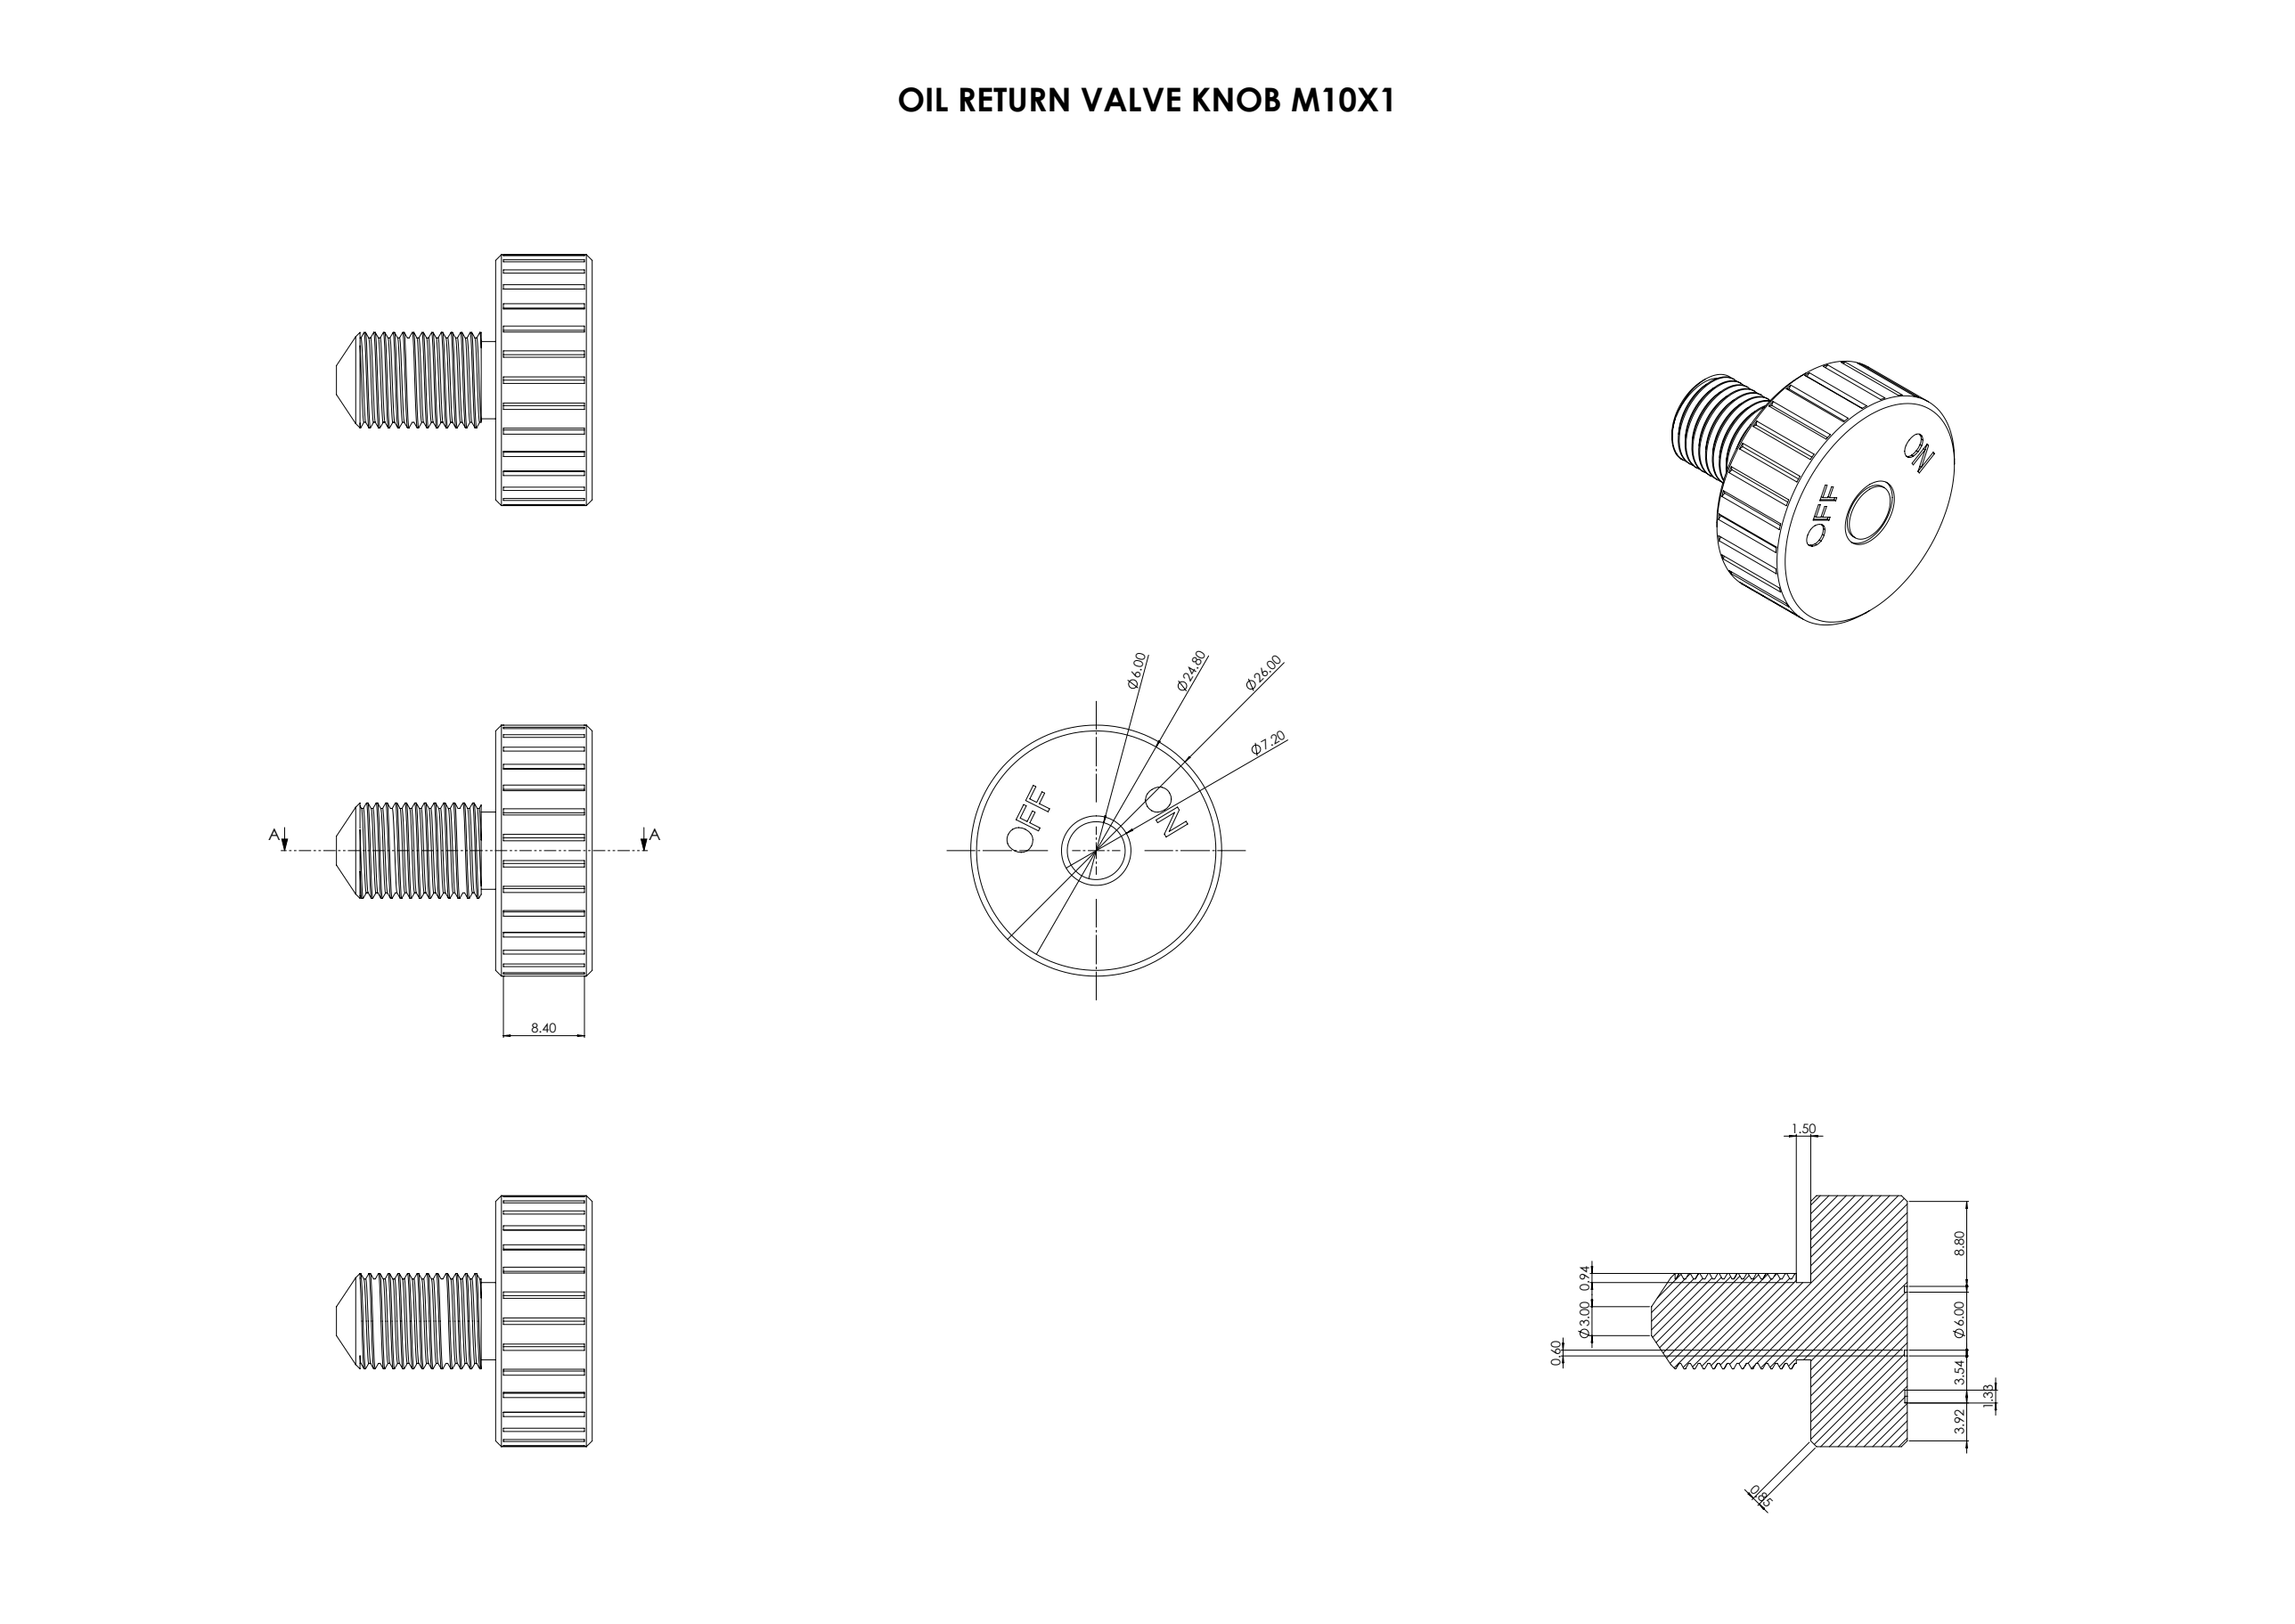
ISO-10303-21;
HEADER;
/* Generated by software containing ST-Developer
 * from STEP Tools, Inc. (www.steptools.com) 
 */

FILE_DESCRIPTION(
/* description */ (''),
/* implementation_level */ '2;1');

FILE_NAME(
/* name */ '20_Oil_Return_Valve_Knob_M10x1.step',
/* time_stamp */ '2026-10-26T03:55:20-07:00',
/* author */ (''),
/* organization */ (''),
/* preprocessor_version */ 'ST-DEVELOPER v20.2',
/* originating_system */ 'Autodesk Translation Framework v15.15.0.0',
/* authorisation */ '');

FILE_SCHEMA (('AUTOMOTIVE_DESIGN { 1 0 10303 214 3 1 1 }'));
ENDSEC;

DATA;
#10=MECHANICAL_DESIGN_GEOMETRIC_PRESENTATION_REPRESENTATION('',(#188),#45236);
#148=SHAPE_REPRESENTATION_RELATIONSHIP('SRR','None',#45327,#168);
#168=ADVANCED_BREP_SHAPE_REPRESENTATION('',(#208),#45229);
#188=STYLED_ITEM('',(#45477),#208);
#208=MANIFOLD_SOLID_BREP('Body1',#16530);
#688=B_SPLINE_CURVE_WITH_KNOTS('',3,(#40645,#40646,#40647,#40648,#40649,
#40650,#40651,#40652,#40653,#40654),.UNSPECIFIED.,.F.,.F.,(4,3,3,4),(-4.09293042013065,
-3.99861591915004,-2.99896193936253,-2.06773127522702),.UNSPECIFIED.);
#689=B_SPLINE_CURVE_WITH_KNOTS('',3,(#40657,#40658,#40659,#40660,#40661,
#40662,#40663,#40664,#40665,#40666),.UNSPECIFIED.,.F.,.F.,(4,3,3,4),(0.,
0.499826989893744,0.999653979787498,1.11639350868611),.UNSPECIFIED.);
#690=B_SPLINE_CURVE_WITH_KNOTS('',3,(#40671,#40672,#40673,#40674,#40675,
#40676,#40677,#40678,#40679,#40680,#40681,#40682,#40683,#40684,#40685,#40686,
#40687,#40688,#40689,#40690,#40691,#40692),.UNSPECIFIED.,.F.,.F.,(4,3,3,
3,3,3,3,4),(-10.3761157273102,-9.99653979787509,-8.99688581808759,-7.99723183830008,
-6.99757785851257,-5.99792387872506,-4.99826989893755,-4.09293042013065),
 .UNSPECIFIED.);
#691=B_SPLINE_CURVE_WITH_KNOTS('',3,(#40693,#40694,#40695,#40696,#40697,
#40698,#40699,#40700,#40701,#40702,#40703,#40704,#40705,#40706,#40707,#40708,
#40709,#40710,#40711,#40712,#40713,#40714),.UNSPECIFIED.,.F.,.F.,(4,3,3,
3,3,3,3,4),(1.11639350868611,1.99930795957501,2.99896193936252,3.99861591915003,
4.99826989893754,5.99792387872506,6.99757785851257,7.39957881586569),
 .UNSPECIFIED.);
#692=B_SPLINE_CURVE_WITH_KNOTS('',3,(#40719,#40720,#40721,#40722,#40723,
#40724,#40725,#40726,#40727,#40728,#40729,#40730,#40731,#40732,#40733,#40734,
#40735,#40736,#40737,#40738,#40739,#40740),.UNSPECIFIED.,.F.,.F.,(4,3,3,
3,3,3,3,4),(-16.6593010344898,-15.9944636766002,-14.9948096968126,-13.9951557170251,
-12.9955017372376,-11.9958477574501,-10.9961937776626,-10.3761157273102),
 .UNSPECIFIED.);
#693=B_SPLINE_CURVE_WITH_KNOTS('',3,(#40741,#40742,#40743,#40744,#40745,
#40746,#40747,#40748,#40749,#40750,#40751,#40752,#40753,#40754,#40755,#40756,
#40757,#40758,#40759,#40760,#40761,#40762),.UNSPECIFIED.,.F.,.F.,(4,3,3,
3,3,3,3,4),(7.39957881586569,7.99723183830008,8.99688581808759,9.9965397978751,
10.9961937776626,11.9958477574501,12.9955017372376,13.6827641230453),
 .UNSPECIFIED.);
#694=B_SPLINE_CURVE_WITH_KNOTS('',3,(#40767,#40768,#40769,#40770,#40771,
#40772,#40773,#40774,#40775,#40776,#40777,#40778,#40779,#40780,#40781,#40782,
#40783,#40784,#40785,#40786,#40787,#40788),.UNSPECIFIED.,.F.,.F.,(4,3,3,
3,3,3,3,4),(-22.9424863416694,-21.9923875553252,-20.9927335755377,-19.9930795957502,
-18.9934256159627,-17.9937716361752,-16.9941176563877,-16.6593010344898),
 .UNSPECIFIED.);
#695=B_SPLINE_CURVE_WITH_KNOTS('',3,(#40789,#40790,#40791,#40792,#40793,
#40794,#40795,#40796,#40797,#40798,#40799,#40800,#40801,#40802,#40803,#40804,
#40805,#40806,#40807,#40808,#40809,#40810),.UNSPECIFIED.,.F.,.F.,(4,3,3,
3,3,3,3,4),(13.6827641230453,13.9951557170251,14.9948096968126,15.9944636766002,
16.9941176563877,17.9937716361752,18.9934256159627,19.9659494302249),
 .UNSPECIFIED.);
#696=B_SPLINE_CURVE_WITH_KNOTS('',3,(#40815,#40816,#40817,#40818,#40819,
#40820,#40821,#40822,#40823,#40824,#40825,#40826,#40827,#40828,#40829,#40830,
#40831,#40832,#40833,#40834,#40835,#40836,#40837,#40838,#40839),
 .UNSPECIFIED.,.F.,.F.,(4,3,3,3,3,3,3,3,4),(-29.225671648849,-28.9899654138378,
-27.9903114340503,-26.9906574542627,-25.9910034744752,-24.9913494946877,
-23.9916955149002,-22.9920415351127,-22.9424863416694),.UNSPECIFIED.);
#697=B_SPLINE_CURVE_WITH_KNOTS('',3,(#40840,#40841,#40842,#40843,#40844,
#40845,#40846,#40847,#40848,#40849,#40850,#40851,#40852,#40853,#40854,#40855,
#40856,#40857,#40858,#40859,#40860,#40861,#40862,#40863,#40864),
 .UNSPECIFIED.,.F.,.F.,(4,3,3,3,3,3,3,3,4),(19.9659494302249,19.9930795957502,
20.9927335755377,21.9923875553252,22.9920415351127,23.9916955149002,24.9913494946877,
25.9910034744752,26.2491347374045),.UNSPECIFIED.);
#698=B_SPLINE_CURVE_WITH_KNOTS('',3,(#40869,#40870,#40871,#40872,#40873,
#40874,#40875,#40876,#40877,#40878,#40879,#40880,#40881,#40882,#40883,#40884,
#40885,#40886,#40887,#40888,#40889,#40890),.UNSPECIFIED.,.F.,.F.,(4,3,3,
3,3,3,3,4),(-35.5088569560286,-34.9878892925628,-33.9882353127753,-32.9885813329878,
-31.9889273532003,-30.9892733734128,-29.9896193936253,-29.225671648849),
 .UNSPECIFIED.);
#699=B_SPLINE_CURVE_WITH_KNOTS('',3,(#40891,#40892,#40893,#40894,#40895,
#40896,#40897,#40898,#40899,#40900,#40901,#40902,#40903,#40904,#40905,#40906,
#40907,#40908,#40909,#40910,#40911,#40912),.UNSPECIFIED.,.F.,.F.,(4,3,3,
3,3,3,3,4),(26.2491347374045,26.9906574542628,27.9903114340503,28.9899654138378,
29.9896193936253,30.9892733734128,31.9889273532003,32.532320044584),
 .UNSPECIFIED.);
#700=B_SPLINE_CURVE_WITH_KNOTS('',3,(#40917,#40918,#40919,#40920,#40921,
#40922,#40923,#40924,#40925,#40926,#40927,#40928,#40929,#40930,#40931,#40932,
#40933,#40934,#40935,#40936,#40937,#40938),.UNSPECIFIED.,.F.,.F.,(4,3,3,
3,3,3,3,4),(-41.7920422632082,-40.9858131712879,-39.9861591915004,-38.9865052117129,
-37.9868512319254,-36.9871972521378,-35.9875432723503,-35.5088569560286),
 .UNSPECIFIED.);
#701=B_SPLINE_CURVE_WITH_KNOTS('',3,(#40939,#40940,#40941,#40942,#40943,
#40944,#40945,#40946,#40947,#40948,#40949,#40950,#40951,#40952,#40953,#40954,
#40955,#40956,#40957,#40958,#40959,#40960),.UNSPECIFIED.,.F.,.F.,(4,3,3,
3,3,3,3,4),(32.532320044584,32.9885813329878,33.9882353127753,34.9878892925628,
35.9875432723503,36.9871972521378,37.9868512319253,38.8155053517636),
 .UNSPECIFIED.);
#702=B_SPLINE_CURVE_WITH_KNOTS('',3,(#40965,#40966,#40967,#40968,#40969,
#40970,#40971,#40972,#40973,#40974,#40975,#40976,#40977,#40978,#40979,#40980,
#40981,#40982,#40983,#40984,#40985,#40986,#40987,#40988,#40989),
 .UNSPECIFIED.,.F.,.F.,(4,3,3,3,3,3,3,3,4),(-48.0752275703878,-47.9833910298005,
-46.9837370500129,-45.9840830702254,-44.9844290904379,-43.9847751106504,
-42.9851211308629,-41.9854671510754,-41.7920422632082),.UNSPECIFIED.);
#703=B_SPLINE_CURVE_WITH_KNOTS('',3,(#40990,#40991,#40992,#40993,#40994,
#40995,#40996,#40997,#40998,#40999,#41000,#41001,#41002,#41003,#41004,#41005,
#41006,#41007,#41008,#41009,#41010,#41011,#41012,#41013,#41014),
 .UNSPECIFIED.,.F.,.F.,(4,3,3,3,3,3,3,3,4),(38.8155053517636,38.9865052117129,
39.9861591915004,40.9858131712879,41.9854671510754,42.9851211308629,43.9847751106504,
44.9844290904379,45.0986906589432),.UNSPECIFIED.);
#704=B_SPLINE_CURVE_WITH_KNOTS('',3,(#41019,#41020,#41021,#41022,#41023,
#41024,#41025,#41026,#41027,#41028,#41029,#41030,#41031,#41032,#41033,#41034,
#41035,#41036,#41037,#41038,#41039,#41040),.UNSPECIFIED.,.F.,.F.,(4,3,3,
3,3,3,3,4),(-54.3584128775673,-53.9813149085255,-52.981660928738,-51.9820069489505,
-50.982352969163,-49.9826989893755,-48.983045009588,-48.0752275703878),
 .UNSPECIFIED.);
#705=B_SPLINE_CURVE_WITH_KNOTS('',3,(#41041,#41042,#41043,#41044,#41045,
#41046,#41047,#41048,#41049,#41050,#41051,#41052,#41053,#41054,#41055,#41056,
#41057,#41058,#41059,#41060,#41061,#41062),.UNSPECIFIED.,.F.,.F.,(4,3,3,
3,3,3,3,4),(45.0986906589432,45.9840830702254,46.9837370500129,47.9833910298004,
48.9830450095879,49.9826989893755,50.982352969163,51.3818759661228),
 .UNSPECIFIED.);
#706=B_SPLINE_CURVE_WITH_KNOTS('',3,(#41067,#41068,#41069,#41070,#41071,
#41072,#41073,#41074,#41075,#41076,#41077,#41078,#41079,#41080,#41081,#41082,
#41083,#41084,#41085,#41086,#41087,#41088),.UNSPECIFIED.,.F.,.F.,(4,3,3,
3,3,3,3,4),(-60.641598184747,-59.9792387872506,-58.979584807463,-57.9799308276755,
-56.980276847888,-55.9806228681005,-54.980968888313,-54.3584128775673),
 .UNSPECIFIED.);
#707=B_SPLINE_CURVE_WITH_KNOTS('',3,(#41089,#41090,#41091,#41092,#41093,
#41094,#41095,#41096,#41097,#41098,#41099,#41100,#41101,#41102,#41103,#41104,
#41105,#41106,#41107,#41108,#41109,#41110),.UNSPECIFIED.,.F.,.F.,(4,3,3,
3,3,3,3,4),(51.3818759661228,51.9820069489505,52.981660928738,53.9813149085255,
54.980968888313,55.9806228681005,56.980276847888,57.6650612733024),
 .UNSPECIFIED.);
#708=B_SPLINE_CURVE_WITH_KNOTS('',3,(#41115,#41116,#41117,#41118,#41119,
#41120,#41121,#41122,#41123,#41124,#41125,#41126,#41127,#41128,#41129,#41130,
#41131,#41132,#41133,#41134,#41135,#41136),.UNSPECIFIED.,.F.,.F.,(4,3,3,
3,3,3,3,4),(-66.9247834919265,-65.9771626659756,-64.9775086861881,-63.9778547064006,
-62.9782007266131,-61.9785467468256,-60.9788927670381,-60.641598184747),
 .UNSPECIFIED.);
#709=B_SPLINE_CURVE_WITH_KNOTS('',3,(#41137,#41138,#41139,#41140,#41141,
#41142,#41143,#41144,#41145,#41146,#41147,#41148,#41149,#41150,#41151,#41152,
#41153,#41154,#41155,#41156,#41157,#41158),.UNSPECIFIED.,.F.,.F.,(4,3,3,
3,3,3,3,4),(57.6650612733024,57.9799308276755,58.9795848074631,59.9792387872506,
60.9788927670381,61.9785467468256,62.9782007266131,63.948246580482),
 .UNSPECIFIED.);
#710=B_SPLINE_CURVE_WITH_KNOTS('',3,(#41163,#41164,#41165,#41166,#41167,
#41168,#41169,#41170,#41171,#41172,#41173,#41174,#41175,#41176,#41177,#41178,
#41179,#41180,#41181,#41182,#41183,#41184,#41185,#41186,#41187),
 .UNSPECIFIED.,.F.,.F.,(4,3,3,3,3,3,3,3,4),(-73.2079687991061,-72.9747405244882,
-71.9750865447007,-70.9754325649132,-69.9757785851257,-68.9761246053381,
-67.9764706255506,-66.9768166457631,-66.9247834919265),.UNSPECIFIED.);
#711=B_SPLINE_CURVE_WITH_KNOTS('',3,(#41188,#41189,#41190,#41191,#41192,
#41193,#41194,#41195,#41196,#41197,#41198,#41199,#41200,#41201,#41202,#41203,
#41204,#41205,#41206,#41207,#41208,#41209,#41210,#41211,#41212),
 .UNSPECIFIED.,.F.,.F.,(4,3,3,3,3,3,3,3,4),(63.948246580482,63.9778547064006,
64.9775086861881,65.9771626659756,66.9768166457631,67.9764706255506,68.9761246053382,
69.9757785851257,70.2314318876616),.UNSPECIFIED.);
#712=B_SPLINE_CURVE_WITH_KNOTS('',3,(#41217,#41218,#41219,#41220,#41221,
#41222,#41223,#41224,#41225,#41226,#41227,#41228,#41229,#41230,#41231,#41232,
#41233,#41234,#41235,#41236,#41237,#41238),.UNSPECIFIED.,.F.,.F.,(4,3,3,
3,3,3,3,4),(-79.4911541062857,-78.9726644032132,-77.9730104234257,-76.9733564436382,
-75.9737024638507,-74.9740484840632,-73.9743945042757,-73.2079687991061),
 .UNSPECIFIED.);
#713=B_SPLINE_CURVE_WITH_KNOTS('',3,(#41239,#41240,#41241,#41242,#41243,
#41244,#41245,#41246,#41247,#41248,#41249,#41250,#41251,#41252,#41253,#41254,
#41255,#41256,#41257,#41258,#41259,#41260),.UNSPECIFIED.,.F.,.F.,(4,3,3,
3,3,3,3,4),(70.2314318876616,70.9754325649132,71.9750865447007,72.9747405244882,
73.9743945042757,74.9740484840632,75.9737024638507,76.5146171948412),
 .UNSPECIFIED.);
#714=B_SPLINE_CURVE_WITH_KNOTS('',3,(#41266,#41267,#41268,#41269,#41270,
#41271,#41272,#41273,#41274),.UNSPECIFIED.,.F.,.F.,(4,1,1,1,1,1,4),(84.8230016469244,
85.5894273520939,86.5890813318814,87.588735311669,88.5883892914565,89.588043271244,
90.5192739353795),.UNSPECIFIED.);
#715=B_SPLINE_CURVE_WITH_KNOTS('',3,(#41277,#41278,#41279,#41280,#41281,
#41282,#41283,#41284,#41285),.UNSPECIFIED.,.F.,.F.,(4,1,1,1,1,1,4),(84.8230016469244,
85.2817408957214,86.2813948755089,87.2810488552964,88.2807028350839,88.7805298249777,
89.2803568148714),.UNSPECIFIED.);
#716=B_SPLINE_CURVE_WITH_KNOTS('',3,(#41290,#41291,#41292,#41293,#41294,
#41295,#41296,#41297,#41298,#41299,#41300),.UNSPECIFIED.,.F.,.F.,(4,1,1,
1,1,1,1,1,4),(78.5398163397448,78.5918494935814,79.5915034733689,80.5911574531564,
81.5908114329439,82.5904654127314,83.5901193925189,84.5897733723064,84.8230016469244),
 .UNSPECIFIED.);
#717=B_SPLINE_CURVE_WITH_KNOTS('',3,(#41301,#41302,#41303,#41304,#41305,
#41306,#41307,#41308,#41309,#41310),.UNSPECIFIED.,.F.,.F.,(4,1,1,1,1,1,
1,4),(78.5398163397448,79.2838170169963,80.2834709967838,81.2831249765713,
82.2827789563588,83.2824329361463,84.2820869159339,84.8230016469244),
 .UNSPECIFIED.);
#718=B_SPLINE_CURVE_WITH_KNOTS('',3,(#41315,#41316,#41317,#41318,#41319,
#41320,#41321,#41322,#41323,#41324),.UNSPECIFIED.,.F.,.F.,(4,1,1,1,1,1,
1,4),(72.2566310325652,72.5939256148563,73.5935795946438,74.5932335744313,
75.5928875542188,76.5925415340064,77.5921955137939,78.5398163397448),
 .UNSPECIFIED.);
#719=B_SPLINE_CURVE_WITH_KNOTS('',3,(#41325,#41326,#41327,#41328,#41329,
#41330,#41331,#41332,#41333,#41334,#41335),.UNSPECIFIED.,.F.,.F.,(4,1,1,
1,1,1,1,1,4),(72.2566310325652,72.2862391584838,73.2858931382713,74.2855471180588,
75.2852010978463,76.2848550776338,77.2845090574213,78.2841630372088,78.5398163397448),
 .UNSPECIFIED.);
#720=B_SPLINE_CURVE_WITH_KNOTS('',3,(#41340,#41341,#41342,#41343,#41344,
#41345,#41346,#41347,#41348,#41349),.UNSPECIFIED.,.F.,.F.,(4,1,1,1,1,1,
1,4),(65.9734457253856,66.5960017361313,67.5956557159188,68.5953096957063,
69.5949636754938,70.5946176552813,71.5942716350688,72.2566310325652),
 .UNSPECIFIED.);
#721=B_SPLINE_CURVE_WITH_KNOTS('',3,(#41350,#41351,#41352,#41353,#41354,
#41355,#41356,#41357,#41358,#41359),.UNSPECIFIED.,.F.,.F.,(4,1,1,1,1,1,
1,4),(65.9734457253856,66.2883152797587,67.2879692595462,68.2876232393337,
69.2872772191212,70.2869311989087,71.2865851786962,72.2566310325652),
 .UNSPECIFIED.);
#722=B_SPLINE_CURVE_WITH_KNOTS('',3,(#41364,#41365,#41366,#41367,#41368,
#41369,#41370,#41371,#41372,#41373),.UNSPECIFIED.,.F.,.F.,(4,1,1,1,1,1,
1,4),(59.690260418206,60.5980778574062,61.5977318371937,62.5973858169812,
63.5970397967687,64.5966937765562,65.5963477563437,65.9734457253856),
 .UNSPECIFIED.);
#723=B_SPLINE_CURVE_WITH_KNOTS('',3,(#41374,#41375,#41376,#41377,#41378,
#41379,#41380,#41381,#41382,#41383),.UNSPECIFIED.,.F.,.F.,(4,1,1,1,1,1,
1,4),(59.690260418206,60.2903914010336,61.2900453808211,62.2896993606087,
63.2893533403962,64.2890073201837,65.2886612999712,65.9734457253856),
 .UNSPECIFIED.);
#724=B_SPLINE_CURVE_WITH_KNOTS('',3,(#41388,#41389,#41390,#41391,#41392,
#41393,#41394,#41395,#41396,#41397,#41398),.UNSPECIFIED.,.F.,.F.,(4,1,1,
1,1,1,1,1,4),(53.4070751110265,53.6004999988936,54.6001539786812,55.5998079584687,
56.5994619382562,57.5991159180437,58.5987698978312,59.5984238776187,59.690260418206),
 .UNSPECIFIED.);
#725=B_SPLINE_CURVE_WITH_KNOTS('',3,(#41399,#41400,#41401,#41402,#41403,
#41404,#41405,#41406,#41407,#41408),.UNSPECIFIED.,.F.,.F.,(4,1,1,1,1,1,
1,4),(53.4070751110264,54.2924675223086,55.2921215020961,56.2917754818836,
57.2914294616711,58.2910834414586,59.2907374212461,59.690260418206),
 .UNSPECIFIED.);
#726=B_SPLINE_CURVE_WITH_KNOTS('',3,(#41413,#41414,#41415,#41416,#41417,
#41418,#41419,#41420,#41421,#41422),.UNSPECIFIED.,.F.,.F.,(4,1,1,1,1,1,
1,4),(47.1238898038469,47.6025761201686,48.6022300999561,49.6018840797436,
50.6015380595311,51.6011920393186,52.6008460191061,53.4070751110265),
 .UNSPECIFIED.);
#727=B_SPLINE_CURVE_WITH_KNOTS('',3,(#41423,#41424,#41425,#41426,#41427,
#41428,#41429,#41430,#41431,#41432,#41433),.UNSPECIFIED.,.F.,.F.,(4,1,1,
1,1,1,1,1,4),(47.1238898038468,47.294889663796,48.2945436435835,49.294197623371,
50.2938516031585,51.2935055829461,52.2931595627336,53.2928135425211,53.4070751110264),
 .UNSPECIFIED.);
#728=B_SPLINE_CURVE_WITH_KNOTS('',3,(#41438,#41439,#41440,#41441,#41442,
#41443,#41444,#41445,#41446,#41447),.UNSPECIFIED.,.F.,.F.,(4,1,1,1,1,1,
1,4),(40.8407044966673,41.6046522414435,42.604306221231,43.6039602010186,
44.6036141808061,45.6032681605936,46.6029221403811,47.1238898038469),
 .UNSPECIFIED.);
#729=B_SPLINE_CURVE_WITH_KNOTS('',3,(#41448,#41449,#41450,#41451,#41452,
#41453,#41454,#41455,#41456,#41457),.UNSPECIFIED.,.F.,.F.,(4,1,1,1,1,1,
1,4),(40.8407044966673,41.296965785071,42.2966197648585,43.296273744646,
44.2959277244335,45.295581704221,46.2952356840085,47.1238898038468),
 .UNSPECIFIED.);
#730=B_SPLINE_CURVE_WITH_KNOTS('',3,(#41462,#41463,#41464,#41465,#41466,
#41467,#41468,#41469,#41470,#41471,#41472),.UNSPECIFIED.,.F.,.F.,(4,1,1,
1,1,1,1,1,4),(34.5575191894877,34.607074382931,35.6067283627185,36.606382342506,
37.6060363222935,38.605690302081,39.6053442818685,40.604998261656,40.8407044966673),
 .UNSPECIFIED.);
#731=B_SPLINE_CURVE_WITH_KNOTS('',3,(#41473,#41474,#41475,#41476,#41477,
#41478,#41479,#41480,#41481,#41482),.UNSPECIFIED.,.F.,.F.,(4,1,1,1,1,1,
1,4),(34.5575191894877,35.2990419063459,36.2986958861334,37.2983498659209,
38.2980038457084,39.2976578254959,40.2973118052834,40.8407044966673),
 .UNSPECIFIED.);
#732=B_SPLINE_CURVE_WITH_KNOTS('',3,(#41487,#41488,#41489,#41490,#41491,
#41492,#41493,#41494,#41495,#41496),.UNSPECIFIED.,.F.,.F.,(4,1,1,1,1,1,
1,4),(28.2743338823081,28.6091505042059,29.6088044839934,30.6084584637809,
31.6081124435684,32.6077664233559,33.6074204031435,34.5575191894877),
 .UNSPECIFIED.);
#733=B_SPLINE_CURVE_WITH_KNOTS('',3,(#41497,#41498,#41499,#41500,#41501,
#41502,#41503,#41504,#41505,#41506,#41507),.UNSPECIFIED.,.F.,.F.,(4,1,1,
1,1,1,1,1,4),(28.2743338823081,28.3014640478333,29.3011180276209,30.3007720074084,
31.3004259871959,32.3000799669834,33.2997339467709,34.2993879265584,34.5575191894877),
 .UNSPECIFIED.);
#734=B_SPLINE_CURVE_WITH_KNOTS('',3,(#41512,#41513,#41514,#41515,#41516,
#41517,#41518,#41519,#41520,#41521),.UNSPECIFIED.,.F.,.F.,(4,1,1,1,1,1,
1,4),(21.9911485751285,22.6112266254809,23.6108806052684,24.6105345850559,
25.6101885648434,26.6098425446309,27.6094965244184,28.2743338823081),
 .UNSPECIFIED.);
#735=B_SPLINE_CURVE_WITH_KNOTS('',3,(#41522,#41523,#41524,#41525,#41526,
#41527,#41528,#41529,#41530,#41531),.UNSPECIFIED.,.F.,.F.,(4,1,1,1,1,1,
1,4),(21.9911485751285,22.3035401691083,23.3031941488958,24.3028481286833,
25.3025021084708,26.3021560882583,27.3018100680458,28.2743338823081),
 .UNSPECIFIED.);
#736=B_SPLINE_CURVE_WITH_KNOTS('',3,(#41536,#41537,#41538,#41539,#41540,
#41541,#41542,#41543,#41544,#41545),.UNSPECIFIED.,.F.,.F.,(4,1,1,1,1,1,
1,4),(15.7079632679489,16.6133027467558,17.6129567265433,18.6126107063308,
19.6122646861183,20.6119186659058,21.6115726456933,21.9911485751285),
 .UNSPECIFIED.);
#737=B_SPLINE_CURVE_WITH_KNOTS('',3,(#41546,#41547,#41548,#41549,#41550,
#41551,#41552,#41553,#41554,#41555),.UNSPECIFIED.,.F.,.F.,(4,1,1,1,1,1,
1,4),(15.7079632679489,16.3056162903832,17.3052702701707,18.3049242499582,
19.3045782297458,20.3042322095333,21.3038861893208,21.9911485751285),
 .UNSPECIFIED.);
#738=B_SPLINE_CURVE_WITH_KNOTS('',3,(#41901,#41902,#41903,#41904,#41905,
#41906,#41907,#41908,#41909,#41910,#41911,#41912,#41913,#41914,#41915,#41916,
#41917,#41918,#41919,#41920,#41921,#41922,#41923,#41924,#41925,#41926,#41927,
#41928,#41929,#41930,#41931,#41932,#41933,#41934,#41935,#41936,#41937,#41938,
#41939,#41940,#41941,#41942,#41943,#41944,#41945,#41946,#41947,#41948,#41949,
#41950,#41951,#41952,#41953,#41954,#41955,#41956,#41957,#41958,#41959,#41960,
#41961,#41962,#41963,#41964,#41965,#41966,#41967,#41968,#41969,#41970,#41971,
#41972,#41973,#41974,#41975,#41976,#41977,#41978,#41979,#41980,#41981,#41982,
#41983,#41984,#41985,#41986,#41987,#41988,#41989,#41990,#41991,#41992,#41993,
#41994,#41995,#41996,#41997,#41998,#41999,#42000,#42001,#42002,#42003,#42004,
#42005,#42006),.UNSPECIFIED.,.F.,.F.,(4,3,3,3,3,3,3,3,3,3,3,3,3,3,3,3,3,
3,3,3,3,3,3,3,3,3,3,3,3,3,3,3,3,3,3,4),(0.,0.0338555796810951,0.0769233841266441,
0.120787014647652,0.164925431151007,0.18768890800956,0.194695307248219,
0.238000863207828,0.281439200502724,0.324499409932901,0.366791407667859,
0.3748100813225,0.380721434265749,0.423140467769373,0.465072972528112,0.506007047124889,
0.514994378647384,0.543782123537011,0.559160795079789,0.5652443143728,0.606242278680173,
0.647897807448946,0.68940569438575,0.717351016075074,0.73199453794532,0.73810671067074,
0.744081074726445,0.745296337764399,0.786338138284623,0.827324070719474,
0.844968273899783,0.854029216944208,0.860905275211015,0.901330989685579,
0.941119121741644,0.968477696161942),.UNSPECIFIED.);
#739=B_SPLINE_CURVE_WITH_KNOTS('',3,(#42007,#42008,#42009,#42010,#42011,
#42012,#42013,#42014,#42015,#42016),.UNSPECIFIED.,.F.,.F.,(4,3,3,4),(76.5146171948412,
76.9733564436382,77.9730104234257,78.9042410875612),.UNSPECIFIED.);
#740=B_SPLINE_CURVE_WITH_KNOTS('',3,(#42018,#42019,#42020,#42021,#42022,
#42023,#42024,#42025,#42026,#42027,#42028,#42029,#42030,#42031,#42032,#42033,
#42034,#42035,#42036,#42037,#42038,#42039,#42040,#42041,#42042,#42043,#42044,
#42045,#42046,#42047,#42048,#42049,#42050,#42051,#42052,#42053,#42054,#42055,
#42056,#42057,#42058,#42059,#42060,#42061,#42062,#42063,#42064,#42065,#42066,
#42067,#42068,#42069,#42070,#42071,#42072,#42073,#42074,#42075,#42076,#42077,
#42078,#42079,#42080,#42081,#42082,#42083,#42084,#42085,#42086,#42087,#42088,
#42089,#42090,#42091,#42092,#42093,#42094,#42095,#42096,#42097,#42098,#42099,
#42100,#42101,#42102,#42103,#42104,#42105,#42106,#42107,#42108,#42109,#42110,
#42111,#42112,#42113,#42114,#42115,#42116,#42117,#42118,#42119,#42120,#42121,
#42122,#42123),.UNSPECIFIED.,.F.,.F.,(4,3,3,3,3,3,3,3,3,3,3,3,3,3,3,3,3,
3,3,3,3,3,3,3,3,3,3,3,3,3,3,3,3,3,3,4),(-0.968477696161962,-0.93834507440756,
-0.898946379179402,-0.87294341376282,-0.858683439823016,-0.849690155368511,
-0.809511368983842,-0.768684814425123,-0.750823196805684,-0.741908901548402,
-0.734140763767536,-0.692650400513915,-0.650694074697968,-0.608745289151999,
-0.577283699992522,-0.564269250932409,-0.556001088558624,-0.513396717295649,
-0.482898932514091,-0.441404470015905,-0.399314127094565,-0.388144431730235,
-0.378349906522554,-0.373280079897934,-0.331122936037102,-0.287943314322124,
-0.244763692607147,-0.214168231031253,-0.200545763543443,-0.193054146419399,
-0.187017976020424,-0.143637415837001,-0.0997905213121978,-0.0560615532128227,
-0.0129908569656951,0.),.UNSPECIFIED.);
#741=B_SPLINE_CURVE_WITH_KNOTS('',3,(#42124,#42125,#42126,#42127,#42128,
#42129,#42130,#42131,#42132),.UNSPECIFIED.,.F.,.F.,(4,1,1,1,1,1,4),(10.3761157273102,
11.3073463914457,12.3070003712332,13.3066543510207,14.3063083308082,15.3059623105957,
15.7079632679489),.UNSPECIFIED.);
#742=B_SPLINE_CURVE_WITH_KNOTS('',3,(#42138,#42139,#42140,#42141,#42142,
#42143,#42144,#42145,#42146,#42147,#42148,#42149,#42150,#42151,#42152,#42153,
#42154,#42155,#42156,#42157,#42158,#42159,#42160,#42161,#42162,#42163,#42164,
#42165,#42166,#42167,#42168,#42169,#42170,#42171,#42172,#42173,#42174,#42175,
#42176,#42177,#42178,#42179,#42180,#42181,#42182,#42183,#42184,#42185,#42186,
#42187,#42188,#42189,#42190,#42191,#42192,#42193,#42194,#42195,#42196,#42197,
#42198,#42199,#42200,#42201,#42202,#42203,#42204,#42205,#42206,#42207,#42208,
#42209,#42210,#42211,#42212,#42213,#42214,#42215,#42216,#42217,#42218,#42219,
#42220,#42221,#42222,#42223,#42224,#42225,#42226,#42227,#42228,#42229,#42230,
#42231,#42232,#42233,#42234,#42235,#42236,#42237,#42238,#42239,#42240,#42241,
#42242,#42243,#42244,#42245,#42246,#42247,#42248,#42249),.UNSPECIFIED.,
 .F.,.F.,(4,3,3,3,3,3,3,3,3,3,3,3,3,3,3,3,3,3,3,3,3,3,3,3,3,3,3,3,3,3,3,
3,3,3,3,3,3,4),(-0.965990216419493,-0.932232205964582,-0.888725512381132,
-0.86148182111266,-0.845752215774746,-0.838628962985686,-0.795398770998977,
-0.752577231134802,-0.732526991421503,-0.722290315506079,-0.715478178658122,
-0.709647482806995,-0.666593990274609,-0.623625418609477,-0.580925676978502,
-0.54890087075527,-0.536423601193463,-0.530582682015647,-0.525159930165745,
-0.483534316458395,-0.452826452085574,-0.410953138863345,-0.368980079811334,
-0.356959708801849,-0.350330796437256,-0.345496631210951,-0.304366782550378,
-0.263166867623492,-0.222981343541229,-0.195108675598575,-0.181421822833585,
-0.173192140728228,-0.16726444049677,-0.125448330372578,-0.0850057436766688,
-0.0449541457505024,-0.00571652159400748,0.),.UNSPECIFIED.);
#743=B_SPLINE_CURVE_WITH_KNOTS('',3,(#42252,#42253,#42254,#42255,#42256,
#42257,#42258,#42259,#42260),.UNSPECIFIED.,.F.,.F.,(4,1,1,1,1,1,4),(11.6150328478183,
12.114859837712,12.6146868276058,13.6143408073933,14.6139947871808,15.6136487669683,
15.7079632679489),.UNSPECIFIED.);
#744=B_SPLINE_CURVE_WITH_KNOTS('',3,(#42606,#42607,#42608,#42609,#42610,
#42611,#42612,#42613,#42614,#42615,#42616,#42617,#42618,#42619,#42620,#42621,
#42622,#42623,#42624,#42625,#42626,#42627,#42628,#42629,#42630,#42631,#42632,
#42633,#42634,#42635,#42636,#42637,#42638,#42639,#42640,#42641,#42642,#42643,
#42644,#42645,#42646,#42647,#42648,#42649,#42650,#42651,#42652,#42653,#42654,
#42655,#42656,#42657,#42658,#42659,#42660,#42661,#42662,#42663,#42664,#42665,
#42666,#42667,#42668,#42669,#42670,#42671,#42672,#42673,#42674,#42675,#42676,
#42677,#42678,#42679,#42680,#42681,#42682,#42683,#42684,#42685,#42686,#42687,
#42688,#42689,#42690,#42691,#42692,#42693,#42694,#42695,#42696,#42697,#42698,
#42699,#42700,#42701,#42702,#42703,#42704,#42705,#42706,#42707,#42708,#42709,
#42710,#42711,#42712,#42713,#42714),.UNSPECIFIED.,.F.,.F.,(4,3,3,3,3,3,
3,3,3,3,3,3,3,3,3,3,3,3,3,3,3,3,3,3,3,3,3,3,3,3,3,3,3,3,3,3,4),(0.,0.0300808882250601,
0.0690837691274257,0.108977971558979,0.149535303300715,0.161775980247188,
0.169677926634296,0.176345077737452,0.217218238973177,0.258694872125898,
0.300344044967144,0.341653389143491,0.347771209594167,0.352609284959025,
0.39494049143562,0.437189104774325,0.478722267806855,0.48483985412653,0.51451003945568,
0.524490292215405,0.530274299792254,0.571233373520478,0.613481573281312,
0.656140144392953,0.689170740576341,0.705686038668035,0.714536893087061,
0.720494023679387,0.722201336759729,0.765231119221639,0.808568534613332,
0.828246244839095,0.838610463895481,0.846178719169224,0.890004704789425,
0.933557298850571,0.965990216419437),.UNSPECIFIED.);
#745=B_SPLINE_CURVE_WITH_KNOTS('',3,(#42715,#42716,#42717,#42718,#42719,
#42720,#42721,#42722,#42723,#42724),.UNSPECIFIED.,.F.,.F.,(4,3,3,4),(-80.9719723627883,
-80.4721453728945,-79.9723183830007,-79.4911541062857),.UNSPECIFIED.);
#746=B_SPLINE_CURVE_WITH_KNOTS('',2,(#42737,#42738,#42739),
 .UNSPECIFIED.,.F.,.F.,(3,3),(0.,1.),.UNSPECIFIED.);
#747=B_SPLINE_CURVE_WITH_KNOTS('',2,(#42743,#42744,#42745),
 .UNSPECIFIED.,.F.,.F.,(3,3),(0.,1.),.UNSPECIFIED.);
#748=B_SPLINE_CURVE_WITH_KNOTS('',2,(#42754,#42755,#42756),
 .UNSPECIFIED.,.F.,.F.,(3,3),(0.,1.),.UNSPECIFIED.);
#749=B_SPLINE_CURVE_WITH_KNOTS('',2,(#42759,#42760,#42761),
 .UNSPECIFIED.,.F.,.F.,(3,3),(0.,1.),.UNSPECIFIED.);
#750=B_SPLINE_CURVE_WITH_KNOTS('',2,(#42769,#42770,#42771),
 .UNSPECIFIED.,.F.,.F.,(3,3),(0.,1.),.UNSPECIFIED.);
#751=B_SPLINE_CURVE_WITH_KNOTS('',2,(#42774,#42775,#42776),
 .UNSPECIFIED.,.F.,.F.,(3,3),(0.,1.),.UNSPECIFIED.);
#752=B_SPLINE_CURVE_WITH_KNOTS('',2,(#42784,#42785,#42786),
 .UNSPECIFIED.,.F.,.F.,(3,3),(0.,1.),.UNSPECIFIED.);
#753=B_SPLINE_CURVE_WITH_KNOTS('',2,(#42789,#42790,#42791),
 .UNSPECIFIED.,.F.,.F.,(3,3),(0.,1.),.UNSPECIFIED.);
#754=B_SPLINE_CURVE_WITH_KNOTS('',2,(#42799,#42800,#42801),
 .UNSPECIFIED.,.F.,.F.,(3,3),(0.,1.),.UNSPECIFIED.);
#755=B_SPLINE_CURVE_WITH_KNOTS('',2,(#42804,#42805,#42806),
 .UNSPECIFIED.,.F.,.F.,(3,3),(0.,1.),.UNSPECIFIED.);
#756=B_SPLINE_CURVE_WITH_KNOTS('',2,(#42814,#42815,#42816),
 .UNSPECIFIED.,.F.,.F.,(3,3),(0.,1.),.UNSPECIFIED.);
#757=B_SPLINE_CURVE_WITH_KNOTS('',2,(#42819,#42820,#42821),
 .UNSPECIFIED.,.F.,.F.,(3,3),(0.,1.),.UNSPECIFIED.);
#758=B_SPLINE_CURVE_WITH_KNOTS('',2,(#42829,#42830,#42831),
 .UNSPECIFIED.,.F.,.F.,(3,3),(0.,1.),.UNSPECIFIED.);
#759=B_SPLINE_CURVE_WITH_KNOTS('',2,(#42834,#42835,#42836),
 .UNSPECIFIED.,.F.,.F.,(3,3),(0.,1.),.UNSPECIFIED.);
#760=B_SPLINE_CURVE_WITH_KNOTS('',2,(#42844,#42845,#42846),
 .UNSPECIFIED.,.F.,.F.,(3,3),(0.,1.),.UNSPECIFIED.);
#761=B_SPLINE_CURVE_WITH_KNOTS('',2,(#42849,#42850,#42851),
 .UNSPECIFIED.,.F.,.F.,(3,3),(0.,1.),.UNSPECIFIED.);
#762=B_SPLINE_CURVE_WITH_KNOTS('',2,(#42859,#42860,#42861),
 .UNSPECIFIED.,.F.,.F.,(3,3),(0.,1.),.UNSPECIFIED.);
#763=B_SPLINE_CURVE_WITH_KNOTS('',2,(#42864,#42865,#42866),
 .UNSPECIFIED.,.F.,.F.,(3,3),(0.,1.),.UNSPECIFIED.);
#764=B_SPLINE_CURVE_WITH_KNOTS('',2,(#42874,#42875,#42876),
 .UNSPECIFIED.,.F.,.F.,(3,3),(0.,1.),.UNSPECIFIED.);
#765=B_SPLINE_CURVE_WITH_KNOTS('',2,(#42879,#42880,#42881),
 .UNSPECIFIED.,.F.,.F.,(3,3),(0.,1.),.UNSPECIFIED.);
#766=B_SPLINE_CURVE_WITH_KNOTS('',2,(#42888,#42889,#42890),
 .UNSPECIFIED.,.F.,.F.,(3,3),(0.,1.),.UNSPECIFIED.);
#767=B_SPLINE_CURVE_WITH_KNOTS('',2,(#42891,#42892,#42893),
 .UNSPECIFIED.,.F.,.F.,(3,3),(0.,1.),.UNSPECIFIED.);
#768=B_SPLINE_CURVE_WITH_KNOTS('',2,(#42964,#42965,#42966),
 .UNSPECIFIED.,.F.,.F.,(3,3),(0.,1.),.UNSPECIFIED.);
#769=B_SPLINE_CURVE_WITH_KNOTS('',2,(#42970,#42971,#42972),
 .UNSPECIFIED.,.F.,.F.,(3,3),(0.,1.),.UNSPECIFIED.);
#770=B_SPLINE_CURVE_WITH_KNOTS('',2,(#42981,#42982,#42983),
 .UNSPECIFIED.,.F.,.F.,(3,3),(0.,1.),.UNSPECIFIED.);
#771=B_SPLINE_CURVE_WITH_KNOTS('',2,(#42986,#42987,#42988),
 .UNSPECIFIED.,.F.,.F.,(3,3),(0.,1.),.UNSPECIFIED.);
#772=B_SPLINE_CURVE_WITH_KNOTS('',2,(#42996,#42997,#42998),
 .UNSPECIFIED.,.F.,.F.,(3,3),(0.,1.),.UNSPECIFIED.);
#773=B_SPLINE_CURVE_WITH_KNOTS('',2,(#43001,#43002,#43003),
 .UNSPECIFIED.,.F.,.F.,(3,3),(0.,1.),.UNSPECIFIED.);
#774=B_SPLINE_CURVE_WITH_KNOTS('',2,(#43011,#43012,#43013),
 .UNSPECIFIED.,.F.,.F.,(3,3),(0.,1.),.UNSPECIFIED.);
#775=B_SPLINE_CURVE_WITH_KNOTS('',2,(#43016,#43017,#43018),
 .UNSPECIFIED.,.F.,.F.,(3,3),(0.,1.),.UNSPECIFIED.);
#776=B_SPLINE_CURVE_WITH_KNOTS('',2,(#43026,#43027,#43028),
 .UNSPECIFIED.,.F.,.F.,(3,3),(0.,1.),.UNSPECIFIED.);
#777=B_SPLINE_CURVE_WITH_KNOTS('',2,(#43031,#43032,#43033),
 .UNSPECIFIED.,.F.,.F.,(3,3),(0.,1.),.UNSPECIFIED.);
#778=B_SPLINE_CURVE_WITH_KNOTS('',2,(#43041,#43042,#43043),
 .UNSPECIFIED.,.F.,.F.,(3,3),(0.,1.),.UNSPECIFIED.);
#779=B_SPLINE_CURVE_WITH_KNOTS('',2,(#43046,#43047,#43048),
 .UNSPECIFIED.,.F.,.F.,(3,3),(0.,1.),.UNSPECIFIED.);
#780=B_SPLINE_CURVE_WITH_KNOTS('',2,(#43056,#43057,#43058),
 .UNSPECIFIED.,.F.,.F.,(3,3),(0.,1.),.UNSPECIFIED.);
#781=B_SPLINE_CURVE_WITH_KNOTS('',2,(#43061,#43062,#43063),
 .UNSPECIFIED.,.F.,.F.,(3,3),(0.,1.),.UNSPECIFIED.);
#782=B_SPLINE_CURVE_WITH_KNOTS('',2,(#43071,#43072,#43073),
 .UNSPECIFIED.,.F.,.F.,(3,3),(0.,1.),.UNSPECIFIED.);
#783=B_SPLINE_CURVE_WITH_KNOTS('',2,(#43076,#43077,#43078),
 .UNSPECIFIED.,.F.,.F.,(3,3),(0.,1.),.UNSPECIFIED.);
#784=B_SPLINE_CURVE_WITH_KNOTS('',2,(#43086,#43087,#43088),
 .UNSPECIFIED.,.F.,.F.,(3,3),(0.,1.),.UNSPECIFIED.);
#785=B_SPLINE_CURVE_WITH_KNOTS('',2,(#43091,#43092,#43093),
 .UNSPECIFIED.,.F.,.F.,(3,3),(0.,1.),.UNSPECIFIED.);
#786=B_SPLINE_CURVE_WITH_KNOTS('',2,(#43101,#43102,#43103),
 .UNSPECIFIED.,.F.,.F.,(3,3),(0.,1.),.UNSPECIFIED.);
#787=B_SPLINE_CURVE_WITH_KNOTS('',2,(#43106,#43107,#43108),
 .UNSPECIFIED.,.F.,.F.,(3,3),(0.,1.),.UNSPECIFIED.);
#788=B_SPLINE_CURVE_WITH_KNOTS('',2,(#43115,#43116,#43117),
 .UNSPECIFIED.,.F.,.F.,(3,3),(0.,1.),.UNSPECIFIED.);
#789=B_SPLINE_CURVE_WITH_KNOTS('',2,(#43118,#43119,#43120),
 .UNSPECIFIED.,.F.,.F.,(3,3),(0.,1.),.UNSPECIFIED.);
#907=B_SPLINE_SURFACE_WITH_KNOTS('',3,3,((#41556,#41557,#41558,#41559,#41560,
#41561,#41562,#41563,#41564,#41565,#41566,#41567,#41568,#41569,#41570,#41571,
#41572,#41573,#41574,#41575,#41576,#41577,#41578,#41579,#41580,#41581,#41582,
#41583,#41584,#41585,#41586,#41587,#41588,#41589,#41590,#41591,#41592,#41593,
#41594,#41595,#41596,#41597,#41598,#41599,#41600,#41601,#41602,#41603,#41604,
#41605,#41606,#41607,#41608,#41609,#41610,#41611,#41612,#41613,#41614,#41615,
#41616,#41617,#41618,#41619,#41620,#41621,#41622,#41623,#41624,#41625,#41626,
#41627,#41628,#41629,#41630,#41631,#41632,#41633,#41634,#41635,#41636,#41637,
#41638,#41639,#41640,#41641),(#41642,#41643,#41644,#41645,#41646,#41647,
#41648,#41649,#41650,#41651,#41652,#41653,#41654,#41655,#41656,#41657,#41658,
#41659,#41660,#41661,#41662,#41663,#41664,#41665,#41666,#41667,#41668,#41669,
#41670,#41671,#41672,#41673,#41674,#41675,#41676,#41677,#41678,#41679,#41680,
#41681,#41682,#41683,#41684,#41685,#41686,#41687,#41688,#41689,#41690,#41691,
#41692,#41693,#41694,#41695,#41696,#41697,#41698,#41699,#41700,#41701,#41702,
#41703,#41704,#41705,#41706,#41707,#41708,#41709,#41710,#41711,#41712,#41713,
#41714,#41715,#41716,#41717,#41718,#41719,#41720,#41721,#41722,#41723,#41724,
#41725,#41726,#41727),(#41728,#41729,#41730,#41731,#41732,#41733,#41734,
#41735,#41736,#41737,#41738,#41739,#41740,#41741,#41742,#41743,#41744,#41745,
#41746,#41747,#41748,#41749,#41750,#41751,#41752,#41753,#41754,#41755,#41756,
#41757,#41758,#41759,#41760,#41761,#41762,#41763,#41764,#41765,#41766,#41767,
#41768,#41769,#41770,#41771,#41772,#41773,#41774,#41775,#41776,#41777,#41778,
#41779,#41780,#41781,#41782,#41783,#41784,#41785,#41786,#41787,#41788,#41789,
#41790,#41791,#41792,#41793,#41794,#41795,#41796,#41797,#41798,#41799,#41800,
#41801,#41802,#41803,#41804,#41805,#41806,#41807,#41808,#41809,#41810,#41811,
#41812,#41813),(#41814,#41815,#41816,#41817,#41818,#41819,#41820,#41821,
#41822,#41823,#41824,#41825,#41826,#41827,#41828,#41829,#41830,#41831,#41832,
#41833,#41834,#41835,#41836,#41837,#41838,#41839,#41840,#41841,#41842,#41843,
#41844,#41845,#41846,#41847,#41848,#41849,#41850,#41851,#41852,#41853,#41854,
#41855,#41856,#41857,#41858,#41859,#41860,#41861,#41862,#41863,#41864,#41865,
#41866,#41867,#41868,#41869,#41870,#41871,#41872,#41873,#41874,#41875,#41876,
#41877,#41878,#41879,#41880,#41881,#41882,#41883,#41884,#41885,#41886,#41887,
#41888,#41889,#41890,#41891,#41892,#41893,#41894,#41895,#41896,#41897,#41898,
#41899)),.UNSPECIFIED.,.F.,.F.,.F.,(4,4),(4,1,1,1,1,1,1,1,1,1,1,1,1,1,1,
1,1,1,1,1,1,1,1,1,1,1,1,1,1,1,1,1,1,1,1,1,1,1,1,1,1,1,1,1,1,1,1,1,1,1,1,
1,1,1,1,1,1,1,1,1,1,1,1,1,1,1,1,1,1,1,1,1,1,1,1,1,1,1,1,1,1,1,1,4),(0.,
0.0658179306876173),(8.30838445208316,8.80821144197691,9.30803843187066,
10.3076924116582,11.3073463914457,12.3070003712332,13.3066543510207,14.3063083308082,
15.3059623105957,16.3056162903832,17.3052702701707,18.3049242499582,19.3045782297458,
20.3042322095333,21.3038861893208,22.3035401691083,23.3031941488958,24.3028481286833,
25.3025021084708,26.3021560882583,27.3018100680458,28.3014640478333,29.3011180276209,
30.3007720074084,31.3004259871959,32.3000799669834,33.2997339467709,34.2993879265584,
35.2990419063459,36.2986958861334,37.2983498659209,38.2980038457084,39.2976578254959,
40.2973118052834,41.296965785071,42.2966197648585,43.296273744646,44.2959277244335,
45.295581704221,46.2952356840085,47.294889663796,48.2945436435835,49.294197623371,
50.2938516031585,51.2935055829461,52.2931595627336,53.2928135425211,54.2924675223086,
55.2921215020961,56.2917754818836,57.2914294616711,58.2910834414586,59.2907374212461,
60.2903914010336,61.2900453808211,62.2896993606087,63.2893533403962,64.2890073201837,
65.2886612999712,66.2883152797587,67.2879692595462,68.2876232393337,69.2872772191212,
70.2869311989087,71.2865851786962,72.2862391584838,73.2858931382713,74.2855471180588,
75.2852010978463,76.2848550776338,77.2845090574213,78.2841630372088,79.2838170169963,
80.2834709967838,81.2831249765713,82.2827789563588,83.2824329361463,84.2820869159339,
85.2817408957214,86.2813948755089,87.2810488552964,88.2807028350839,88.7805298249777,
89.2803568148714),.UNSPECIFIED.);
#908=B_SPLINE_SURFACE_WITH_KNOTS('',3,3,((#42261,#42262,#42263,#42264,#42265,
#42266,#42267,#42268,#42269,#42270,#42271,#42272,#42273,#42274,#42275,#42276,
#42277,#42278,#42279,#42280,#42281,#42282,#42283,#42284,#42285,#42286,#42287,
#42288,#42289,#42290,#42291,#42292,#42293,#42294,#42295,#42296,#42297,#42298,
#42299,#42300,#42301,#42302,#42303,#42304,#42305,#42306,#42307,#42308,#42309,
#42310,#42311,#42312,#42313,#42314,#42315,#42316,#42317,#42318,#42319,#42320,
#42321,#42322,#42323,#42324,#42325,#42326,#42327,#42328,#42329,#42330,#42331,
#42332,#42333,#42334,#42335,#42336,#42337,#42338,#42339,#42340,#42341,#42342,
#42343,#42344,#42345,#42346),(#42347,#42348,#42349,#42350,#42351,#42352,
#42353,#42354,#42355,#42356,#42357,#42358,#42359,#42360,#42361,#42362,#42363,
#42364,#42365,#42366,#42367,#42368,#42369,#42370,#42371,#42372,#42373,#42374,
#42375,#42376,#42377,#42378,#42379,#42380,#42381,#42382,#42383,#42384,#42385,
#42386,#42387,#42388,#42389,#42390,#42391,#42392,#42393,#42394,#42395,#42396,
#42397,#42398,#42399,#42400,#42401,#42402,#42403,#42404,#42405,#42406,#42407,
#42408,#42409,#42410,#42411,#42412,#42413,#42414,#42415,#42416,#42417,#42418,
#42419,#42420,#42421,#42422,#42423,#42424,#42425,#42426,#42427,#42428,#42429,
#42430,#42431,#42432),(#42433,#42434,#42435,#42436,#42437,#42438,#42439,
#42440,#42441,#42442,#42443,#42444,#42445,#42446,#42447,#42448,#42449,#42450,
#42451,#42452,#42453,#42454,#42455,#42456,#42457,#42458,#42459,#42460,#42461,
#42462,#42463,#42464,#42465,#42466,#42467,#42468,#42469,#42470,#42471,#42472,
#42473,#42474,#42475,#42476,#42477,#42478,#42479,#42480,#42481,#42482,#42483,
#42484,#42485,#42486,#42487,#42488,#42489,#42490,#42491,#42492,#42493,#42494,
#42495,#42496,#42497,#42498,#42499,#42500,#42501,#42502,#42503,#42504,#42505,
#42506,#42507,#42508,#42509,#42510,#42511,#42512,#42513,#42514,#42515,#42516,
#42517,#42518),(#42519,#42520,#42521,#42522,#42523,#42524,#42525,#42526,
#42527,#42528,#42529,#42530,#42531,#42532,#42533,#42534,#42535,#42536,#42537,
#42538,#42539,#42540,#42541,#42542,#42543,#42544,#42545,#42546,#42547,#42548,
#42549,#42550,#42551,#42552,#42553,#42554,#42555,#42556,#42557,#42558,#42559,
#42560,#42561,#42562,#42563,#42564,#42565,#42566,#42567,#42568,#42569,#42570,
#42571,#42572,#42573,#42574,#42575,#42576,#42577,#42578,#42579,#42580,#42581,
#42582,#42583,#42584,#42585,#42586,#42587,#42588,#42589,#42590,#42591,#42592,
#42593,#42594,#42595,#42596,#42597,#42598,#42599,#42600,#42601,#42602,#42603,
#42604)),.UNSPECIFIED.,.F.,.F.,.F.,(4,4),(4,1,1,1,1,1,1,1,1,1,1,1,1,1,1,
1,1,1,1,1,1,1,1,1,1,1,1,1,1,1,1,1,1,1,1,1,1,1,1,1,1,1,1,1,1,1,1,1,1,1,1,
1,1,1,1,1,1,1,1,1,1,1,1,1,1,1,1,1,1,1,1,1,1,1,1,1,1,1,1,1,1,1,1,4),(0.,
0.0658179306876173),(11.6150328478183,12.114859837712,12.6146868276058,
13.6143408073933,14.6139947871808,15.6136487669683,16.6133027467558,17.6129567265433,
18.6126107063308,19.6122646861183,20.6119186659058,21.6115726456933,22.6112266254809,
23.6108806052684,24.6105345850559,25.6101885648434,26.6098425446309,27.6094965244184,
28.6091505042059,29.6088044839934,30.6084584637809,31.6081124435684,32.6077664233559,
33.6074204031435,34.607074382931,35.6067283627185,36.606382342506,37.6060363222935,
38.605690302081,39.6053442818685,40.604998261656,41.6046522414435,42.604306221231,
43.6039602010186,44.6036141808061,45.6032681605936,46.6029221403811,47.6025761201686,
48.6022300999561,49.6018840797436,50.6015380595311,51.6011920393186,52.6008460191061,
53.6004999988936,54.6001539786812,55.5998079584687,56.5994619382562,57.5991159180437,
58.5987698978312,59.5984238776187,60.5980778574062,61.5977318371937,62.5973858169812,
63.5970397967687,64.5966937765562,65.5963477563437,66.5960017361313,67.5956557159188,
68.5953096957063,69.5949636754938,70.5946176552813,71.5942716350688,72.5939256148563,
73.5935795946438,74.5932335744313,75.5928875542188,76.5925415340064,77.5921955137939,
78.5918494935814,79.5915034733689,80.5911574531564,81.5908114329439,82.5904654127314,
83.5901193925189,84.5897733723064,85.5894273520939,86.5890813318814,87.588735311669,
88.5883892914565,89.588043271244,90.5876972510315,91.587351230819,92.0871782207128,
92.5870052106065),.UNSPECIFIED.);
#909=B_SPLINE_SURFACE_WITH_KNOTS('',2,1,((#42729,#42730),(#42731,#42732),
(#42733,#42734)),.UNSPECIFIED.,.F.,.F.,.F.,(3,3),(2,2),(0.,1.),(0.,0.0249999999999999),
 .UNSPECIFIED.);
#910=B_SPLINE_SURFACE_WITH_KNOTS('',2,1,((#42747,#42748),(#42749,#42750),
(#42751,#42752)),.UNSPECIFIED.,.F.,.F.,.F.,(3,3),(2,2),(0.,1.),(0.,0.0249999999999999),
 .UNSPECIFIED.);
#911=B_SPLINE_SURFACE_WITH_KNOTS('',2,1,((#42762,#42763),(#42764,#42765),
(#42766,#42767)),.UNSPECIFIED.,.F.,.F.,.F.,(3,3),(2,2),(0.,1.),(0.,0.0249999999999999),
 .UNSPECIFIED.);
#912=B_SPLINE_SURFACE_WITH_KNOTS('',2,1,((#42777,#42778),(#42779,#42780),
(#42781,#42782)),.UNSPECIFIED.,.F.,.F.,.F.,(3,3),(2,2),(0.,1.),(0.,0.0249999999999999),
 .UNSPECIFIED.);
#913=B_SPLINE_SURFACE_WITH_KNOTS('',2,1,((#42792,#42793),(#42794,#42795),
(#42796,#42797)),.UNSPECIFIED.,.F.,.F.,.F.,(3,3),(2,2),(0.,1.),(0.,0.0249999999999999),
 .UNSPECIFIED.);
#914=B_SPLINE_SURFACE_WITH_KNOTS('',2,1,((#42807,#42808),(#42809,#42810),
(#42811,#42812)),.UNSPECIFIED.,.F.,.F.,.F.,(3,3),(2,2),(0.,1.),(0.,0.0249999999999999),
 .UNSPECIFIED.);
#915=B_SPLINE_SURFACE_WITH_KNOTS('',2,1,((#42822,#42823),(#42824,#42825),
(#42826,#42827)),.UNSPECIFIED.,.F.,.F.,.F.,(3,3),(2,2),(0.,1.),(0.,0.0249999999999999),
 .UNSPECIFIED.);
#916=B_SPLINE_SURFACE_WITH_KNOTS('',2,1,((#42837,#42838),(#42839,#42840),
(#42841,#42842)),.UNSPECIFIED.,.F.,.F.,.F.,(3,3),(2,2),(0.,1.),(0.,0.0249999999999999),
 .UNSPECIFIED.);
#917=B_SPLINE_SURFACE_WITH_KNOTS('',2,1,((#42852,#42853),(#42854,#42855),
(#42856,#42857)),.UNSPECIFIED.,.F.,.F.,.F.,(3,3),(2,2),(0.,1.),(0.,0.0249999999999999),
 .UNSPECIFIED.);
#918=B_SPLINE_SURFACE_WITH_KNOTS('',2,1,((#42867,#42868),(#42869,#42870),
(#42871,#42872)),.UNSPECIFIED.,.F.,.F.,.F.,(3,3),(2,2),(0.,1.),(0.,0.0249999999999999),
 .UNSPECIFIED.);
#919=B_SPLINE_SURFACE_WITH_KNOTS('',2,1,((#42882,#42883),(#42884,#42885),
(#42886,#42887)),.UNSPECIFIED.,.F.,.F.,.F.,(3,3),(2,2),(0.,1.),(0.,0.0249999999999999),
 .UNSPECIFIED.);
#920=B_SPLINE_SURFACE_WITH_KNOTS('',2,1,((#42956,#42957),(#42958,#42959),
(#42960,#42961)),.UNSPECIFIED.,.F.,.F.,.F.,(3,3),(2,2),(0.,1.),(0.,0.0249999999999999),
 .UNSPECIFIED.);
#921=B_SPLINE_SURFACE_WITH_KNOTS('',2,1,((#42974,#42975),(#42976,#42977),
(#42978,#42979)),.UNSPECIFIED.,.F.,.F.,.F.,(3,3),(2,2),(0.,1.),(0.,0.0249999999999999),
 .UNSPECIFIED.);
#922=B_SPLINE_SURFACE_WITH_KNOTS('',2,1,((#42989,#42990),(#42991,#42992),
(#42993,#42994)),.UNSPECIFIED.,.F.,.F.,.F.,(3,3),(2,2),(0.,1.),(0.,0.0249999999999999),
 .UNSPECIFIED.);
#923=B_SPLINE_SURFACE_WITH_KNOTS('',2,1,((#43004,#43005),(#43006,#43007),
(#43008,#43009)),.UNSPECIFIED.,.F.,.F.,.F.,(3,3),(2,2),(0.,1.),(0.,0.0249999999999999),
 .UNSPECIFIED.);
#924=B_SPLINE_SURFACE_WITH_KNOTS('',2,1,((#43019,#43020),(#43021,#43022),
(#43023,#43024)),.UNSPECIFIED.,.F.,.F.,.F.,(3,3),(2,2),(0.,1.),(0.,0.0249999999999999),
 .UNSPECIFIED.);
#925=B_SPLINE_SURFACE_WITH_KNOTS('',2,1,((#43034,#43035),(#43036,#43037),
(#43038,#43039)),.UNSPECIFIED.,.F.,.F.,.F.,(3,3),(2,2),(0.,1.),(0.,0.0249999999999999),
 .UNSPECIFIED.);
#926=B_SPLINE_SURFACE_WITH_KNOTS('',2,1,((#43049,#43050),(#43051,#43052),
(#43053,#43054)),.UNSPECIFIED.,.F.,.F.,.F.,(3,3),(2,2),(0.,1.),(0.,0.0249999999999999),
 .UNSPECIFIED.);
#927=B_SPLINE_SURFACE_WITH_KNOTS('',2,1,((#43064,#43065),(#43066,#43067),
(#43068,#43069)),.UNSPECIFIED.,.F.,.F.,.F.,(3,3),(2,2),(0.,1.),(0.,0.0249999999999999),
 .UNSPECIFIED.);
#928=B_SPLINE_SURFACE_WITH_KNOTS('',2,1,((#43079,#43080),(#43081,#43082),
(#43083,#43084)),.UNSPECIFIED.,.F.,.F.,.F.,(3,3),(2,2),(0.,1.),(0.,0.0249999999999999),
 .UNSPECIFIED.);
#929=B_SPLINE_SURFACE_WITH_KNOTS('',2,1,((#43094,#43095),(#43096,#43097),
(#43098,#43099)),.UNSPECIFIED.,.F.,.F.,.F.,(3,3),(2,2),(0.,1.),(0.,0.0249999999999999),
 .UNSPECIFIED.);
#930=B_SPLINE_SURFACE_WITH_KNOTS('',2,1,((#43109,#43110),(#43111,#43112),
(#43113,#43114)),.UNSPECIFIED.,.F.,.F.,.F.,(3,3),(2,2),(0.,1.),(0.,0.0249999999999999),
 .UNSPECIFIED.);
#1004=FACE_BOUND('',#3508,.T.);
#1005=FACE_BOUND('',#3567,.T.);
#1006=FACE_BOUND('',#3697,.T.);
#1007=FACE_BOUND('',#3700,.T.);
#1008=FACE_BOUND('',#3701,.T.);
#1009=FACE_BOUND('',#3702,.T.);
#1010=FACE_BOUND('',#3703,.T.);
#1011=FACE_BOUND('',#3704,.T.);
#1012=FACE_BOUND('',#3705,.T.);
#1013=FACE_BOUND('',#3706,.T.);
#1014=FACE_BOUND('',#3707,.T.);
#1015=FACE_BOUND('',#3708,.T.);
#1016=FACE_BOUND('',#3709,.T.);
#1017=FACE_BOUND('',#3710,.T.);
#1018=FACE_BOUND('',#3711,.T.);
#1019=FACE_BOUND('',#3712,.T.);
#1020=FACE_BOUND('',#3713,.T.);
#1021=FACE_BOUND('',#3714,.T.);
#1022=FACE_BOUND('',#3715,.T.);
#1023=FACE_BOUND('',#3716,.T.);
#1024=FACE_BOUND('',#3717,.T.);
#1025=FACE_BOUND('',#3718,.T.);
#1026=FACE_BOUND('',#3719,.T.);
#1027=FACE_BOUND('',#3720,.T.);
#1028=FACE_BOUND('',#3721,.T.);
#1029=FACE_BOUND('',#3722,.T.);
#1030=FACE_BOUND('',#3723,.T.);
#1031=FACE_BOUND('',#3724,.T.);
#1032=FACE_BOUND('',#3725,.T.);
#1033=FACE_BOUND('',#3726,.T.);
#1034=FACE_BOUND('',#3727,.T.);
#1035=FACE_BOUND('',#3728,.T.);
#1036=FACE_BOUND('',#3731,.T.);
#1037=FACE_BOUND('',#3732,.T.);
#1038=FACE_BOUND('',#3733,.T.);
#1039=FACE_BOUND('',#3734,.T.);
#1040=FACE_BOUND('',#3735,.T.);
#1041=FACE_BOUND('',#3736,.T.);
#1336=PLANE('',#17629);
#1337=PLANE('',#17634);
#1338=PLANE('',#17637);
#1339=PLANE('',#17638);
#1340=PLANE('',#17639);
#1341=PLANE('',#17640);
#1342=PLANE('',#17641);
#1343=PLANE('',#17642);
#1344=PLANE('',#17643);
#1345=PLANE('',#17644);
#1346=PLANE('',#17645);
#1347=PLANE('',#17646);
#1348=PLANE('',#17647);
#1349=PLANE('',#17648);
#1350=PLANE('',#17649);
#1351=PLANE('',#17650);
#1352=PLANE('',#17651);
#1353=PLANE('',#17652);
#1354=PLANE('',#17653);
#1355=PLANE('',#17654);
#1356=PLANE('',#17655);
#1357=PLANE('',#17656);
#1358=PLANE('',#17657);
#1359=PLANE('',#17658);
#1360=PLANE('',#17659);
#1361=PLANE('',#17660);
#1362=PLANE('',#17661);
#1363=PLANE('',#17662);
#1364=PLANE('',#17663);
#1365=PLANE('',#17664);
#1366=PLANE('',#17665);
#1367=PLANE('',#17666);
#1368=PLANE('',#17667);
#1369=PLANE('',#17668);
#1370=PLANE('',#17669);
#1371=PLANE('',#17670);
#1372=PLANE('',#17671);
#1373=PLANE('',#17672);
#1374=PLANE('',#17679);
#1375=PLANE('',#17680);
#1376=PLANE('',#17681);
#1377=PLANE('',#17683);
#1378=PLANE('',#17684);
#1379=PLANE('',#17686);
#1380=PLANE('',#17687);
#1381=PLANE('',#17689);
#1382=PLANE('',#17690);
#1383=PLANE('',#17692);
#1384=PLANE('',#17693);
#1385=PLANE('',#17695);
#1386=PLANE('',#17696);
#1387=PLANE('',#17698);
#1388=PLANE('',#17699);
#1389=PLANE('',#17701);
#1390=PLANE('',#17702);
#1391=PLANE('',#17704);
#1392=PLANE('',#17705);
#1393=PLANE('',#17707);
#1394=PLANE('',#17708);
#1395=PLANE('',#17710);
#1396=PLANE('',#17711);
#1397=PLANE('',#17713);
#1398=PLANE('',#17714);
#1399=PLANE('',#17716);
#1400=PLANE('',#17717);
#1401=PLANE('',#17719);
#1402=PLANE('',#17720);
#1403=PLANE('',#17722);
#1404=PLANE('',#17723);
#1405=PLANE('',#17725);
#1406=PLANE('',#17726);
#1407=PLANE('',#17728);
#1408=PLANE('',#17729);
#1409=PLANE('',#17731);
#1410=PLANE('',#17732);
#1411=PLANE('',#17734);
#1412=PLANE('',#17735);
#1413=PLANE('',#17737);
#1414=PLANE('',#17738);
#1415=PLANE('',#17740);
#1416=PLANE('',#17741);
#1417=PLANE('',#17743);
#1418=PLANE('',#17744);
#1419=PLANE('',#17746);
#1420=PLANE('',#17747);
#1421=PLANE('',#17749);
#1422=PLANE('',#17750);
#1423=PLANE('',#17752);
#1424=PLANE('',#17753);
#1425=PLANE('',#17755);
#1426=PLANE('',#17756);
#1427=PLANE('',#17758);
#1428=PLANE('',#17759);
#1429=PLANE('',#17761);
#1430=PLANE('',#17762);
#1431=PLANE('',#17764);
#1432=PLANE('',#17765);
#1433=PLANE('',#17768);
#1434=PLANE('',#17769);
#1435=PLANE('',#17772);
#1436=PLANE('',#17773);
#1437=PLANE('',#17775);
#1438=PLANE('',#17776);
#1439=PLANE('',#17778);
#1440=PLANE('',#17779);
#1441=PLANE('',#17781);
#1442=PLANE('',#17782);
#1443=PLANE('',#17784);
#1444=PLANE('',#17785);
#1445=PLANE('',#17787);
#1446=PLANE('',#17788);
#1447=PLANE('',#17790);
#1448=PLANE('',#17791);
#1449=PLANE('',#17793);
#1450=PLANE('',#17794);
#1451=PLANE('',#17796);
#1452=PLANE('',#17797);
#1453=PLANE('',#17799);
#1454=PLANE('',#17800);
#1455=PLANE('',#17802);
#1456=PLANE('',#17803);
#1457=PLANE('',#17805);
#1458=PLANE('',#17806);
#1459=PLANE('',#17808);
#1460=PLANE('',#17809);
#1461=PLANE('',#17811);
#1462=PLANE('',#17812);
#1463=PLANE('',#17814);
#1464=PLANE('',#17815);
#1465=PLANE('',#17817);
#1466=PLANE('',#17818);
#1467=PLANE('',#17820);
#1468=PLANE('',#17821);
#1469=PLANE('',#17823);
#1470=PLANE('',#17824);
#1471=PLANE('',#17826);
#1472=PLANE('',#17827);
#1473=PLANE('',#17829);
#1474=PLANE('',#17830);
#1475=PLANE('',#17832);
#1476=PLANE('',#17833);
#1477=PLANE('',#17835);
#1478=PLANE('',#17836);
#1479=PLANE('',#17838);
#1480=PLANE('',#17839);
#1481=PLANE('',#17841);
#1482=PLANE('',#17842);
#1483=PLANE('',#17844);
#1484=PLANE('',#17845);
#1485=PLANE('',#17847);
#1486=PLANE('',#17848);
#1487=PLANE('',#17850);
#1488=PLANE('',#17851);
#1489=PLANE('',#17853);
#1490=PLANE('',#17854);
#1491=PLANE('',#17856);
#1492=PLANE('',#17857);
#1493=PLANE('',#17859);
#1494=PLANE('',#17860);
#1495=PLANE('',#17862);
#1496=PLANE('',#17870);
#1497=PLANE('',#17878);
#1752=CYLINDRICAL_SURFACE('',#17602,4.942);
#1753=CYLINDRICAL_SURFACE('',#17604,4.942);
#1754=CYLINDRICAL_SURFACE('',#17605,4.942);
#1755=CYLINDRICAL_SURFACE('',#17606,4.942);
#1756=CYLINDRICAL_SURFACE('',#17607,4.942);
#1757=CYLINDRICAL_SURFACE('',#17608,4.942);
#1758=CYLINDRICAL_SURFACE('',#17609,4.942);
#1759=CYLINDRICAL_SURFACE('',#17610,4.942);
#1760=CYLINDRICAL_SURFACE('',#17611,4.942);
#1761=CYLINDRICAL_SURFACE('',#17612,4.942);
#1762=CYLINDRICAL_SURFACE('',#17613,4.942);
#1763=CYLINDRICAL_SURFACE('',#17614,4.942);
#1764=CYLINDRICAL_SURFACE('',#17615,4.942);
#1765=CYLINDRICAL_SURFACE('',#17616,4.372);
#1766=CYLINDRICAL_SURFACE('',#17618,4.372);
#1767=CYLINDRICAL_SURFACE('',#17619,4.372);
#1768=CYLINDRICAL_SURFACE('',#17620,4.372);
#1769=CYLINDRICAL_SURFACE('',#17621,4.372);
#1770=CYLINDRICAL_SURFACE('',#17622,4.372);
#1771=CYLINDRICAL_SURFACE('',#17623,4.372);
#1772=CYLINDRICAL_SURFACE('',#17624,4.372);
#1773=CYLINDRICAL_SURFACE('',#17625,4.372);
#1774=CYLINDRICAL_SURFACE('',#17626,4.372);
#1775=CYLINDRICAL_SURFACE('',#17627,4.372);
#1776=CYLINDRICAL_SURFACE('',#17628,4.372);
#1777=CYLINDRICAL_SURFACE('',#17633,4.372);
#1778=CYLINDRICAL_SURFACE('',#17675,3.6);
#1779=CYLINDRICAL_SURFACE('',#17677,3.);
#1780=CYLINDRICAL_SURFACE('',#17867,4.942);
#1781=CYLINDRICAL_SURFACE('',#17868,4.);
#1782=CYLINDRICAL_SURFACE('',#17874,13.);
#2439=FACE_OUTER_BOUND('',#3478,.T.);
#2440=FACE_OUTER_BOUND('',#3479,.T.);
#2441=FACE_OUTER_BOUND('',#3480,.T.);
#2442=FACE_OUTER_BOUND('',#3481,.T.);
#2443=FACE_OUTER_BOUND('',#3482,.T.);
#2444=FACE_OUTER_BOUND('',#3483,.T.);
#2445=FACE_OUTER_BOUND('',#3484,.T.);
#2446=FACE_OUTER_BOUND('',#3485,.T.);
#2447=FACE_OUTER_BOUND('',#3486,.T.);
#2448=FACE_OUTER_BOUND('',#3487,.T.);
#2449=FACE_OUTER_BOUND('',#3488,.T.);
#2450=FACE_OUTER_BOUND('',#3489,.T.);
#2451=FACE_OUTER_BOUND('',#3490,.T.);
#2452=FACE_OUTER_BOUND('',#3491,.T.);
#2453=FACE_OUTER_BOUND('',#3492,.T.);
#2454=FACE_OUTER_BOUND('',#3493,.T.);
#2455=FACE_OUTER_BOUND('',#3494,.T.);
#2456=FACE_OUTER_BOUND('',#3495,.T.);
#2457=FACE_OUTER_BOUND('',#3496,.T.);
#2458=FACE_OUTER_BOUND('',#3497,.T.);
#2459=FACE_OUTER_BOUND('',#3498,.T.);
#2460=FACE_OUTER_BOUND('',#3499,.T.);
#2461=FACE_OUTER_BOUND('',#3500,.T.);
#2462=FACE_OUTER_BOUND('',#3501,.T.);
#2463=FACE_OUTER_BOUND('',#3502,.T.);
#2464=FACE_OUTER_BOUND('',#3503,.T.);
#2465=FACE_OUTER_BOUND('',#3504,.T.);
#2466=FACE_OUTER_BOUND('',#3505,.T.);
#2467=FACE_OUTER_BOUND('',#3506,.T.);
#2468=FACE_OUTER_BOUND('',#3507,.T.);
#2469=FACE_OUTER_BOUND('',#3509,.T.);
#2470=FACE_OUTER_BOUND('',#3510,.T.);
#2471=FACE_OUTER_BOUND('',#3511,.T.);
#2472=FACE_OUTER_BOUND('',#3512,.T.);
#2473=FACE_OUTER_BOUND('',#3513,.T.);
#2474=FACE_OUTER_BOUND('',#3514,.T.);
#2475=FACE_OUTER_BOUND('',#3515,.T.);
#2476=FACE_OUTER_BOUND('',#3516,.T.);
#2477=FACE_OUTER_BOUND('',#3517,.T.);
#2478=FACE_OUTER_BOUND('',#3518,.T.);
#2479=FACE_OUTER_BOUND('',#3519,.T.);
#2480=FACE_OUTER_BOUND('',#3520,.T.);
#2481=FACE_OUTER_BOUND('',#3521,.T.);
#2482=FACE_OUTER_BOUND('',#3522,.T.);
#2483=FACE_OUTER_BOUND('',#3523,.T.);
#2484=FACE_OUTER_BOUND('',#3524,.T.);
#2485=FACE_OUTER_BOUND('',#3525,.T.);
#2486=FACE_OUTER_BOUND('',#3526,.T.);
#2487=FACE_OUTER_BOUND('',#3527,.T.);
#2488=FACE_OUTER_BOUND('',#3528,.T.);
#2489=FACE_OUTER_BOUND('',#3529,.T.);
#2490=FACE_OUTER_BOUND('',#3530,.T.);
#2491=FACE_OUTER_BOUND('',#3531,.T.);
#2492=FACE_OUTER_BOUND('',#3532,.T.);
#2493=FACE_OUTER_BOUND('',#3533,.T.);
#2494=FACE_OUTER_BOUND('',#3534,.T.);
#2495=FACE_OUTER_BOUND('',#3535,.T.);
#2496=FACE_OUTER_BOUND('',#3536,.T.);
#2497=FACE_OUTER_BOUND('',#3537,.T.);
#2498=FACE_OUTER_BOUND('',#3538,.T.);
#2499=FACE_OUTER_BOUND('',#3539,.T.);
#2500=FACE_OUTER_BOUND('',#3540,.T.);
#2501=FACE_OUTER_BOUND('',#3541,.T.);
#2502=FACE_OUTER_BOUND('',#3542,.T.);
#2503=FACE_OUTER_BOUND('',#3543,.T.);
#2504=FACE_OUTER_BOUND('',#3544,.T.);
#2505=FACE_OUTER_BOUND('',#3545,.T.);
#2506=FACE_OUTER_BOUND('',#3546,.T.);
#2507=FACE_OUTER_BOUND('',#3547,.T.);
#2508=FACE_OUTER_BOUND('',#3548,.T.);
#2509=FACE_OUTER_BOUND('',#3549,.T.);
#2510=FACE_OUTER_BOUND('',#3550,.T.);
#2511=FACE_OUTER_BOUND('',#3551,.T.);
#2512=FACE_OUTER_BOUND('',#3552,.T.);
#2513=FACE_OUTER_BOUND('',#3553,.T.);
#2514=FACE_OUTER_BOUND('',#3554,.T.);
#2515=FACE_OUTER_BOUND('',#3555,.T.);
#2516=FACE_OUTER_BOUND('',#3556,.T.);
#2517=FACE_OUTER_BOUND('',#3557,.T.);
#2518=FACE_OUTER_BOUND('',#3558,.T.);
#2519=FACE_OUTER_BOUND('',#3559,.T.);
#2520=FACE_OUTER_BOUND('',#3560,.T.);
#2521=FACE_OUTER_BOUND('',#3561,.T.);
#2522=FACE_OUTER_BOUND('',#3562,.T.);
#2523=FACE_OUTER_BOUND('',#3563,.T.);
#2524=FACE_OUTER_BOUND('',#3564,.T.);
#2525=FACE_OUTER_BOUND('',#3565,.T.);
#2526=FACE_OUTER_BOUND('',#3566,.T.);
#2527=FACE_OUTER_BOUND('',#3568,.T.);
#2528=FACE_OUTER_BOUND('',#3569,.T.);
#2529=FACE_OUTER_BOUND('',#3570,.T.);
#2530=FACE_OUTER_BOUND('',#3571,.T.);
#2531=FACE_OUTER_BOUND('',#3572,.T.);
#2532=FACE_OUTER_BOUND('',#3573,.T.);
#2533=FACE_OUTER_BOUND('',#3574,.T.);
#2534=FACE_OUTER_BOUND('',#3575,.T.);
#2535=FACE_OUTER_BOUND('',#3576,.T.);
#2536=FACE_OUTER_BOUND('',#3577,.T.);
#2537=FACE_OUTER_BOUND('',#3578,.T.);
#2538=FACE_OUTER_BOUND('',#3579,.T.);
#2539=FACE_OUTER_BOUND('',#3580,.T.);
#2540=FACE_OUTER_BOUND('',#3581,.T.);
#2541=FACE_OUTER_BOUND('',#3582,.T.);
#2542=FACE_OUTER_BOUND('',#3583,.T.);
#2543=FACE_OUTER_BOUND('',#3584,.T.);
#2544=FACE_OUTER_BOUND('',#3585,.T.);
#2545=FACE_OUTER_BOUND('',#3586,.T.);
#2546=FACE_OUTER_BOUND('',#3587,.T.);
#2547=FACE_OUTER_BOUND('',#3588,.T.);
#2548=FACE_OUTER_BOUND('',#3589,.T.);
#2549=FACE_OUTER_BOUND('',#3590,.T.);
#2550=FACE_OUTER_BOUND('',#3591,.T.);
#2551=FACE_OUTER_BOUND('',#3592,.T.);
#2552=FACE_OUTER_BOUND('',#3593,.T.);
#2553=FACE_OUTER_BOUND('',#3594,.T.);
#2554=FACE_OUTER_BOUND('',#3595,.T.);
#2555=FACE_OUTER_BOUND('',#3596,.T.);
#2556=FACE_OUTER_BOUND('',#3597,.T.);
#2557=FACE_OUTER_BOUND('',#3598,.T.);
#2558=FACE_OUTER_BOUND('',#3599,.T.);
#2559=FACE_OUTER_BOUND('',#3600,.T.);
#2560=FACE_OUTER_BOUND('',#3601,.T.);
#2561=FACE_OUTER_BOUND('',#3602,.T.);
#2562=FACE_OUTER_BOUND('',#3603,.T.);
#2563=FACE_OUTER_BOUND('',#3604,.T.);
#2564=FACE_OUTER_BOUND('',#3605,.T.);
#2565=FACE_OUTER_BOUND('',#3606,.T.);
#2566=FACE_OUTER_BOUND('',#3607,.T.);
#2567=FACE_OUTER_BOUND('',#3608,.T.);
#2568=FACE_OUTER_BOUND('',#3609,.T.);
#2569=FACE_OUTER_BOUND('',#3610,.T.);
#2570=FACE_OUTER_BOUND('',#3611,.T.);
#2571=FACE_OUTER_BOUND('',#3612,.T.);
#2572=FACE_OUTER_BOUND('',#3613,.T.);
#2573=FACE_OUTER_BOUND('',#3614,.T.);
#2574=FACE_OUTER_BOUND('',#3615,.T.);
#2575=FACE_OUTER_BOUND('',#3616,.T.);
#2576=FACE_OUTER_BOUND('',#3617,.T.);
#2577=FACE_OUTER_BOUND('',#3618,.T.);
#2578=FACE_OUTER_BOUND('',#3619,.T.);
#2579=FACE_OUTER_BOUND('',#3620,.T.);
#2580=FACE_OUTER_BOUND('',#3621,.T.);
#2581=FACE_OUTER_BOUND('',#3622,.T.);
#2582=FACE_OUTER_BOUND('',#3623,.T.);
#2583=FACE_OUTER_BOUND('',#3624,.T.);
#2584=FACE_OUTER_BOUND('',#3625,.T.);
#2585=FACE_OUTER_BOUND('',#3626,.T.);
#2586=FACE_OUTER_BOUND('',#3627,.T.);
#2587=FACE_OUTER_BOUND('',#3628,.T.);
#2588=FACE_OUTER_BOUND('',#3629,.T.);
#2589=FACE_OUTER_BOUND('',#3630,.T.);
#2590=FACE_OUTER_BOUND('',#3631,.T.);
#2591=FACE_OUTER_BOUND('',#3632,.T.);
#2592=FACE_OUTER_BOUND('',#3633,.T.);
#2593=FACE_OUTER_BOUND('',#3634,.T.);
#2594=FACE_OUTER_BOUND('',#3635,.T.);
#2595=FACE_OUTER_BOUND('',#3636,.T.);
#2596=FACE_OUTER_BOUND('',#3637,.T.);
#2597=FACE_OUTER_BOUND('',#3638,.T.);
#2598=FACE_OUTER_BOUND('',#3639,.T.);
#2599=FACE_OUTER_BOUND('',#3640,.T.);
#2600=FACE_OUTER_BOUND('',#3641,.T.);
#2601=FACE_OUTER_BOUND('',#3642,.T.);
#2602=FACE_OUTER_BOUND('',#3643,.T.);
#2603=FACE_OUTER_BOUND('',#3644,.T.);
#2604=FACE_OUTER_BOUND('',#3645,.T.);
#2605=FACE_OUTER_BOUND('',#3646,.T.);
#2606=FACE_OUTER_BOUND('',#3647,.T.);
#2607=FACE_OUTER_BOUND('',#3648,.T.);
#2608=FACE_OUTER_BOUND('',#3649,.T.);
#2609=FACE_OUTER_BOUND('',#3650,.T.);
#2610=FACE_OUTER_BOUND('',#3651,.T.);
#2611=FACE_OUTER_BOUND('',#3652,.T.);
#2612=FACE_OUTER_BOUND('',#3653,.T.);
#2613=FACE_OUTER_BOUND('',#3654,.T.);
#2614=FACE_OUTER_BOUND('',#3655,.T.);
#2615=FACE_OUTER_BOUND('',#3656,.T.);
#2616=FACE_OUTER_BOUND('',#3657,.T.);
#2617=FACE_OUTER_BOUND('',#3658,.T.);
#2618=FACE_OUTER_BOUND('',#3659,.T.);
#2619=FACE_OUTER_BOUND('',#3660,.T.);
#2620=FACE_OUTER_BOUND('',#3661,.T.);
#2621=FACE_OUTER_BOUND('',#3662,.T.);
#2622=FACE_OUTER_BOUND('',#3663,.T.);
#2623=FACE_OUTER_BOUND('',#3664,.T.);
#2624=FACE_OUTER_BOUND('',#3665,.T.);
#2625=FACE_OUTER_BOUND('',#3666,.T.);
#2626=FACE_OUTER_BOUND('',#3667,.T.);
#2627=FACE_OUTER_BOUND('',#3668,.T.);
#2628=FACE_OUTER_BOUND('',#3669,.T.);
#2629=FACE_OUTER_BOUND('',#3670,.T.);
#2630=FACE_OUTER_BOUND('',#3671,.T.);
#2631=FACE_OUTER_BOUND('',#3672,.T.);
#2632=FACE_OUTER_BOUND('',#3673,.T.);
#2633=FACE_OUTER_BOUND('',#3674,.T.);
#2634=FACE_OUTER_BOUND('',#3675,.T.);
#2635=FACE_OUTER_BOUND('',#3676,.T.);
#2636=FACE_OUTER_BOUND('',#3677,.T.);
#2637=FACE_OUTER_BOUND('',#3678,.T.);
#2638=FACE_OUTER_BOUND('',#3679,.T.);
#2639=FACE_OUTER_BOUND('',#3680,.T.);
#2640=FACE_OUTER_BOUND('',#3681,.T.);
#2641=FACE_OUTER_BOUND('',#3682,.T.);
#2642=FACE_OUTER_BOUND('',#3683,.T.);
#2643=FACE_OUTER_BOUND('',#3684,.T.);
#2644=FACE_OUTER_BOUND('',#3685,.T.);
#2645=FACE_OUTER_BOUND('',#3686,.T.);
#2646=FACE_OUTER_BOUND('',#3687,.T.);
#2647=FACE_OUTER_BOUND('',#3688,.T.);
#2648=FACE_OUTER_BOUND('',#3689,.T.);
#2649=FACE_OUTER_BOUND('',#3690,.T.);
#2650=FACE_OUTER_BOUND('',#3691,.T.);
#2651=FACE_OUTER_BOUND('',#3692,.T.);
#2652=FACE_OUTER_BOUND('',#3693,.T.);
#2653=FACE_OUTER_BOUND('',#3694,.T.);
#2654=FACE_OUTER_BOUND('',#3695,.T.);
#2655=FACE_OUTER_BOUND('',#3696,.T.);
#2656=FACE_OUTER_BOUND('',#3698,.T.);
#2657=FACE_OUTER_BOUND('',#3699,.T.);
#2658=FACE_OUTER_BOUND('',#3729,.T.);
#2659=FACE_OUTER_BOUND('',#3730,.T.);
#3478=EDGE_LOOP('',(#13850,#13851,#13852,#13853));
#3479=EDGE_LOOP('',(#13854,#13855,#13856,#13857));
#3480=EDGE_LOOP('',(#13858,#13859,#13860,#13861));
#3481=EDGE_LOOP('',(#13862,#13863,#13864,#13865));
#3482=EDGE_LOOP('',(#13866,#13867,#13868,#13869));
#3483=EDGE_LOOP('',(#13870,#13871,#13872,#13873));
#3484=EDGE_LOOP('',(#13874,#13875,#13876,#13877));
#3485=EDGE_LOOP('',(#13878,#13879,#13880,#13881));
#3486=EDGE_LOOP('',(#13882,#13883,#13884,#13885));
#3487=EDGE_LOOP('',(#13886,#13887,#13888,#13889));
#3488=EDGE_LOOP('',(#13890,#13891,#13892,#13893));
#3489=EDGE_LOOP('',(#13894,#13895,#13896,#13897));
#3490=EDGE_LOOP('',(#13898,#13899,#13900,#13901));
#3491=EDGE_LOOP('',(#13902,#13903,#13904,#13905));
#3492=EDGE_LOOP('',(#13906,#13907,#13908,#13909));
#3493=EDGE_LOOP('',(#13910,#13911,#13912,#13913));
#3494=EDGE_LOOP('',(#13914,#13915,#13916,#13917));
#3495=EDGE_LOOP('',(#13918,#13919,#13920,#13921));
#3496=EDGE_LOOP('',(#13922,#13923,#13924,#13925));
#3497=EDGE_LOOP('',(#13926,#13927,#13928,#13929));
#3498=EDGE_LOOP('',(#13930,#13931,#13932,#13933));
#3499=EDGE_LOOP('',(#13934,#13935,#13936,#13937));
#3500=EDGE_LOOP('',(#13938,#13939,#13940,#13941));
#3501=EDGE_LOOP('',(#13942,#13943,#13944,#13945));
#3502=EDGE_LOOP('',(#13946,#13947,#13948,#13949));
#3503=EDGE_LOOP('',(#13950,#13951,#13952,#13953,#13954,#13955,#13956,#13957,
#13958,#13959,#13960,#13961,#13962,#13963,#13964,#13965,#13966,#13967,#13968,
#13969,#13970,#13971,#13972,#13973,#13974,#13975,#13976,#13977,#13978));
#3504=EDGE_LOOP('',(#13979,#13980,#13981,#13982,#13983));
#3505=EDGE_LOOP('',(#13984,#13985,#13986,#13987));
#3506=EDGE_LOOP('',(#13988,#13989,#13990,#13991,#13992,#13993,#13994,#13995,
#13996,#13997,#13998,#13999,#14000,#14001,#14002,#14003,#14004,#14005,#14006,
#14007,#14008,#14009,#14010,#14011,#14012,#14013,#14014,#14015,#14016));
#3507=EDGE_LOOP('',(#14017,#14018,#14019,#14020));
#3508=EDGE_LOOP('',(#14021));
#3509=EDGE_LOOP('',(#14022,#14023,#14024,#14025));
#3510=EDGE_LOOP('',(#14026,#14027,#14028,#14029));
#3511=EDGE_LOOP('',(#14030,#14031,#14032,#14033));
#3512=EDGE_LOOP('',(#14034,#14035,#14036,#14037));
#3513=EDGE_LOOP('',(#14038,#14039,#14040,#14041));
#3514=EDGE_LOOP('',(#14042,#14043,#14044,#14045));
#3515=EDGE_LOOP('',(#14046,#14047,#14048,#14049));
#3516=EDGE_LOOP('',(#14050,#14051,#14052,#14053));
#3517=EDGE_LOOP('',(#14054,#14055,#14056,#14057));
#3518=EDGE_LOOP('',(#14058,#14059,#14060,#14061));
#3519=EDGE_LOOP('',(#14062,#14063,#14064,#14065));
#3520=EDGE_LOOP('',(#14066,#14067,#14068,#14069,#14070,#14071,#14072,#14073,
#14074,#14075,#14076));
#3521=EDGE_LOOP('',(#14077,#14078,#14079,#14080));
#3522=EDGE_LOOP('',(#14081,#14082,#14083,#14084));
#3523=EDGE_LOOP('',(#14085,#14086,#14087,#14088));
#3524=EDGE_LOOP('',(#14089,#14090,#14091,#14092));
#3525=EDGE_LOOP('',(#14093,#14094,#14095,#14096));
#3526=EDGE_LOOP('',(#14097,#14098,#14099,#14100));
#3527=EDGE_LOOP('',(#14101,#14102,#14103,#14104));
#3528=EDGE_LOOP('',(#14105,#14106,#14107,#14108));
#3529=EDGE_LOOP('',(#14109,#14110,#14111,#14112));
#3530=EDGE_LOOP('',(#14113,#14114,#14115,#14116));
#3531=EDGE_LOOP('',(#14117,#14118,#14119,#14120,#14121,#14122,#14123,#14124,
#14125,#14126));
#3532=EDGE_LOOP('',(#14127,#14128,#14129,#14130));
#3533=EDGE_LOOP('',(#14131,#14132,#14133,#14134));
#3534=EDGE_LOOP('',(#14135,#14136,#14137,#14138));
#3535=EDGE_LOOP('',(#14139,#14140,#14141,#14142));
#3536=EDGE_LOOP('',(#14143,#14144,#14145,#14146));
#3537=EDGE_LOOP('',(#14147,#14148,#14149,#14150));
#3538=EDGE_LOOP('',(#14151,#14152,#14153,#14154));
#3539=EDGE_LOOP('',(#14155,#14156,#14157,#14158));
#3540=EDGE_LOOP('',(#14159,#14160,#14161,#14162));
#3541=EDGE_LOOP('',(#14163,#14164,#14165,#14166));
#3542=EDGE_LOOP('',(#14167,#14168,#14169,#14170));
#3543=EDGE_LOOP('',(#14171,#14172,#14173,#14174,#14175,#14176,#14177,#14178,
#14179,#14180,#14181));
#3544=EDGE_LOOP('',(#14182,#14183,#14184,#14185));
#3545=EDGE_LOOP('',(#14186,#14187,#14188,#14189));
#3546=EDGE_LOOP('',(#14190,#14191,#14192,#14193));
#3547=EDGE_LOOP('',(#14194,#14195,#14196,#14197));
#3548=EDGE_LOOP('',(#14198,#14199,#14200,#14201));
#3549=EDGE_LOOP('',(#14202,#14203,#14204,#14205));
#3550=EDGE_LOOP('',(#14206,#14207,#14208,#14209));
#3551=EDGE_LOOP('',(#14210,#14211,#14212,#14213));
#3552=EDGE_LOOP('',(#14214,#14215,#14216,#14217));
#3553=EDGE_LOOP('',(#14218,#14219,#14220,#14221));
#3554=EDGE_LOOP('',(#14222,#14223,#14224,#14225,#14226,#14227,#14228,#14229,
#14230,#14231));
#3555=EDGE_LOOP('',(#14232,#14233,#14234,#14235));
#3556=EDGE_LOOP('',(#14236,#14237,#14238,#14239));
#3557=EDGE_LOOP('',(#14240,#14241,#14242,#14243));
#3558=EDGE_LOOP('',(#14244,#14245,#14246,#14247));
#3559=EDGE_LOOP('',(#14248,#14249,#14250,#14251));
#3560=EDGE_LOOP('',(#14252,#14253,#14254,#14255));
#3561=EDGE_LOOP('',(#14256,#14257,#14258,#14259));
#3562=EDGE_LOOP('',(#14260,#14261,#14262,#14263));
#3563=EDGE_LOOP('',(#14264,#14265,#14266,#14267));
#3564=EDGE_LOOP('',(#14268,#14269,#14270,#14271));
#3565=EDGE_LOOP('',(#14272,#14273,#14274,#14275,#14276,#14277,#14278,#14279,
#14280,#14281));
#3566=EDGE_LOOP('',(#14282));
#3567=EDGE_LOOP('',(#14283));
#3568=EDGE_LOOP('',(#14284,#14285,#14286,#14287));
#3569=EDGE_LOOP('',(#14288,#14289,#14290,#14291));
#3570=EDGE_LOOP('',(#14292));
#3571=EDGE_LOOP('',(#14293,#14294,#14295,#14296));
#3572=EDGE_LOOP('',(#14297,#14298,#14299));
#3573=EDGE_LOOP('',(#14300,#14301,#14302,#14303));
#3574=EDGE_LOOP('',(#14304,#14305,#14306));
#3575=EDGE_LOOP('',(#14307,#14308,#14309,#14310));
#3576=EDGE_LOOP('',(#14311,#14312,#14313));
#3577=EDGE_LOOP('',(#14314,#14315,#14316,#14317));
#3578=EDGE_LOOP('',(#14318,#14319,#14320));
#3579=EDGE_LOOP('',(#14321,#14322,#14323,#14324));
#3580=EDGE_LOOP('',(#14325,#14326,#14327));
#3581=EDGE_LOOP('',(#14328,#14329,#14330,#14331));
#3582=EDGE_LOOP('',(#14332,#14333,#14334));
#3583=EDGE_LOOP('',(#14335,#14336,#14337,#14338));
#3584=EDGE_LOOP('',(#14339,#14340,#14341));
#3585=EDGE_LOOP('',(#14342,#14343,#14344,#14345));
#3586=EDGE_LOOP('',(#14346,#14347,#14348));
#3587=EDGE_LOOP('',(#14349,#14350,#14351,#14352));
#3588=EDGE_LOOP('',(#14353,#14354,#14355));
#3589=EDGE_LOOP('',(#14356,#14357,#14358,#14359));
#3590=EDGE_LOOP('',(#14360,#14361,#14362));
#3591=EDGE_LOOP('',(#14363,#14364,#14365,#14366));
#3592=EDGE_LOOP('',(#14367,#14368,#14369));
#3593=EDGE_LOOP('',(#14370,#14371,#14372,#14373));
#3594=EDGE_LOOP('',(#14374,#14375,#14376));
#3595=EDGE_LOOP('',(#14377,#14378,#14379,#14380));
#3596=EDGE_LOOP('',(#14381,#14382,#14383));
#3597=EDGE_LOOP('',(#14384,#14385,#14386,#14387));
#3598=EDGE_LOOP('',(#14388,#14389,#14390));
#3599=EDGE_LOOP('',(#14391,#14392,#14393,#14394));
#3600=EDGE_LOOP('',(#14395,#14396,#14397));
#3601=EDGE_LOOP('',(#14398,#14399,#14400,#14401));
#3602=EDGE_LOOP('',(#14402,#14403,#14404));
#3603=EDGE_LOOP('',(#14405,#14406,#14407,#14408));
#3604=EDGE_LOOP('',(#14409,#14410,#14411));
#3605=EDGE_LOOP('',(#14412,#14413,#14414,#14415));
#3606=EDGE_LOOP('',(#14416,#14417,#14418));
#3607=EDGE_LOOP('',(#14419,#14420,#14421,#14422));
#3608=EDGE_LOOP('',(#14423,#14424,#14425));
#3609=EDGE_LOOP('',(#14426,#14427,#14428,#14429));
#3610=EDGE_LOOP('',(#14430,#14431,#14432));
#3611=EDGE_LOOP('',(#14433,#14434,#14435,#14436));
#3612=EDGE_LOOP('',(#14437,#14438,#14439));
#3613=EDGE_LOOP('',(#14440,#14441,#14442,#14443));
#3614=EDGE_LOOP('',(#14444,#14445,#14446));
#3615=EDGE_LOOP('',(#14447,#14448,#14449,#14450));
#3616=EDGE_LOOP('',(#14451,#14452,#14453));
#3617=EDGE_LOOP('',(#14454,#14455,#14456,#14457));
#3618=EDGE_LOOP('',(#14458,#14459,#14460));
#3619=EDGE_LOOP('',(#14461,#14462,#14463,#14464));
#3620=EDGE_LOOP('',(#14465,#14466,#14467));
#3621=EDGE_LOOP('',(#14468,#14469,#14470,#14471));
#3622=EDGE_LOOP('',(#14472,#14473,#14474));
#3623=EDGE_LOOP('',(#14475,#14476,#14477,#14478));
#3624=EDGE_LOOP('',(#14479,#14480,#14481));
#3625=EDGE_LOOP('',(#14482,#14483,#14484,#14485));
#3626=EDGE_LOOP('',(#14486,#14487,#14488));
#3627=EDGE_LOOP('',(#14489,#14490,#14491,#14492));
#3628=EDGE_LOOP('',(#14493,#14494,#14495,#14496));
#3629=EDGE_LOOP('',(#14497,#14498,#14499,#14500));
#3630=EDGE_LOOP('',(#14501,#14502,#14503,#14504));
#3631=EDGE_LOOP('',(#14505,#14506,#14507,#14508));
#3632=EDGE_LOOP('',(#14509,#14510,#14511));
#3633=EDGE_LOOP('',(#14512,#14513,#14514,#14515));
#3634=EDGE_LOOP('',(#14516,#14517,#14518));
#3635=EDGE_LOOP('',(#14519,#14520,#14521,#14522));
#3636=EDGE_LOOP('',(#14523,#14524,#14525));
#3637=EDGE_LOOP('',(#14526,#14527,#14528,#14529));
#3638=EDGE_LOOP('',(#14530,#14531,#14532));
#3639=EDGE_LOOP('',(#14533,#14534,#14535,#14536));
#3640=EDGE_LOOP('',(#14537,#14538,#14539));
#3641=EDGE_LOOP('',(#14540,#14541,#14542,#14543));
#3642=EDGE_LOOP('',(#14544,#14545,#14546));
#3643=EDGE_LOOP('',(#14547,#14548,#14549,#14550));
#3644=EDGE_LOOP('',(#14551,#14552,#14553));
#3645=EDGE_LOOP('',(#14554,#14555,#14556,#14557));
#3646=EDGE_LOOP('',(#14558,#14559,#14560));
#3647=EDGE_LOOP('',(#14561,#14562,#14563,#14564));
#3648=EDGE_LOOP('',(#14565,#14566,#14567));
#3649=EDGE_LOOP('',(#14568,#14569,#14570,#14571));
#3650=EDGE_LOOP('',(#14572,#14573,#14574));
#3651=EDGE_LOOP('',(#14575,#14576,#14577,#14578));
#3652=EDGE_LOOP('',(#14579,#14580,#14581));
#3653=EDGE_LOOP('',(#14582,#14583,#14584,#14585));
#3654=EDGE_LOOP('',(#14586,#14587,#14588));
#3655=EDGE_LOOP('',(#14589,#14590,#14591,#14592));
#3656=EDGE_LOOP('',(#14593,#14594,#14595));
#3657=EDGE_LOOP('',(#14596,#14597,#14598,#14599));
#3658=EDGE_LOOP('',(#14600,#14601,#14602));
#3659=EDGE_LOOP('',(#14603,#14604,#14605,#14606));
#3660=EDGE_LOOP('',(#14607,#14608,#14609));
#3661=EDGE_LOOP('',(#14610,#14611,#14612,#14613));
#3662=EDGE_LOOP('',(#14614,#14615,#14616));
#3663=EDGE_LOOP('',(#14617,#14618,#14619,#14620));
#3664=EDGE_LOOP('',(#14621,#14622,#14623));
#3665=EDGE_LOOP('',(#14624,#14625,#14626,#14627));
#3666=EDGE_LOOP('',(#14628,#14629,#14630));
#3667=EDGE_LOOP('',(#14631,#14632,#14633,#14634));
#3668=EDGE_LOOP('',(#14635,#14636,#14637));
#3669=EDGE_LOOP('',(#14638,#14639,#14640,#14641));
#3670=EDGE_LOOP('',(#14642,#14643,#14644));
#3671=EDGE_LOOP('',(#14645,#14646,#14647,#14648));
#3672=EDGE_LOOP('',(#14649,#14650,#14651));
#3673=EDGE_LOOP('',(#14652,#14653,#14654,#14655));
#3674=EDGE_LOOP('',(#14656,#14657,#14658));
#3675=EDGE_LOOP('',(#14659,#14660,#14661,#14662));
#3676=EDGE_LOOP('',(#14663,#14664,#14665));
#3677=EDGE_LOOP('',(#14666,#14667,#14668,#14669));
#3678=EDGE_LOOP('',(#14670,#14671,#14672));
#3679=EDGE_LOOP('',(#14673,#14674,#14675,#14676));
#3680=EDGE_LOOP('',(#14677,#14678,#14679));
#3681=EDGE_LOOP('',(#14680,#14681,#14682,#14683));
#3682=EDGE_LOOP('',(#14684,#14685,#14686));
#3683=EDGE_LOOP('',(#14687,#14688,#14689,#14690));
#3684=EDGE_LOOP('',(#14691,#14692,#14693));
#3685=EDGE_LOOP('',(#14694,#14695,#14696,#14697));
#3686=EDGE_LOOP('',(#14698,#14699,#14700));
#3687=EDGE_LOOP('',(#14701,#14702,#14703,#14704));
#3688=EDGE_LOOP('',(#14705,#14706,#14707));
#3689=EDGE_LOOP('',(#14708,#14709,#14710,#14711));
#3690=EDGE_LOOP('',(#14712,#14713,#14714));
#3691=EDGE_LOOP('',(#14715));
#3692=EDGE_LOOP('',(#14716,#14717,#14718,#14719));
#3693=EDGE_LOOP('',(#14720,#14721,#14722,#14723,#14724,#14725));
#3694=EDGE_LOOP('',(#14726,#14727,#14728,#14729));
#3695=EDGE_LOOP('',(#14730,#14731,#14732,#14733));
#3696=EDGE_LOOP('',(#14734));
#3697=EDGE_LOOP('',(#14735));
#3698=EDGE_LOOP('',(#14736,#14737,#14738,#14739));
#3699=EDGE_LOOP('',(#14740,#14741,#14742,#14743,#14744,#14745,#14746,#14747,
#14748,#14749,#14750,#14751));
#3700=EDGE_LOOP('',(#14752,#14753,#14754,#14755));
#3701=EDGE_LOOP('',(#14756,#14757,#14758,#14759));
#3702=EDGE_LOOP('',(#14760,#14761,#14762,#14763));
#3703=EDGE_LOOP('',(#14764,#14765,#14766,#14767));
#3704=EDGE_LOOP('',(#14768,#14769,#14770,#14771));
#3705=EDGE_LOOP('',(#14772,#14773,#14774,#14775));
#3706=EDGE_LOOP('',(#14776,#14777,#14778,#14779));
#3707=EDGE_LOOP('',(#14780,#14781,#14782,#14783));
#3708=EDGE_LOOP('',(#14784,#14785,#14786,#14787));
#3709=EDGE_LOOP('',(#14788,#14789,#14790,#14791));
#3710=EDGE_LOOP('',(#14792,#14793,#14794,#14795));
#3711=EDGE_LOOP('',(#14796,#14797,#14798,#14799));
#3712=EDGE_LOOP('',(#14800,#14801,#14802,#14803));
#3713=EDGE_LOOP('',(#14804,#14805,#14806,#14807));
#3714=EDGE_LOOP('',(#14808,#14809,#14810,#14811));
#3715=EDGE_LOOP('',(#14812,#14813,#14814,#14815));
#3716=EDGE_LOOP('',(#14816,#14817,#14818,#14819));
#3717=EDGE_LOOP('',(#14820,#14821,#14822,#14823));
#3718=EDGE_LOOP('',(#14824,#14825,#14826,#14827));
#3719=EDGE_LOOP('',(#14828,#14829,#14830,#14831));
#3720=EDGE_LOOP('',(#14832,#14833,#14834,#14835));
#3721=EDGE_LOOP('',(#14836,#14837,#14838,#14839));
#3722=EDGE_LOOP('',(#14840,#14841,#14842,#14843));
#3723=EDGE_LOOP('',(#14844,#14845,#14846,#14847));
#3724=EDGE_LOOP('',(#14848,#14849,#14850,#14851));
#3725=EDGE_LOOP('',(#14852,#14853,#14854,#14855));
#3726=EDGE_LOOP('',(#14856,#14857,#14858,#14859));
#3727=EDGE_LOOP('',(#14860,#14861,#14862,#14863));
#3728=EDGE_LOOP('',(#14864,#14865,#14866,#14867));
#3729=EDGE_LOOP('',(#14868,#14869,#14870,#14871));
#3730=EDGE_LOOP('',(#14872));
#3731=EDGE_LOOP('',(#14873,#14874,#14875,#14876,#14877,#14878,#14879,#14880,
#14881,#14882,#14883));
#3732=EDGE_LOOP('',(#14884,#14885,#14886,#14887,#14888,#14889,#14890,#14891,
#14892,#14893));
#3733=EDGE_LOOP('',(#14894,#14895,#14896,#14897,#14898,#14899,#14900,#14901,
#14902,#14903,#14904));
#3734=EDGE_LOOP('',(#14905,#14906,#14907,#14908,#14909,#14910,#14911,#14912,
#14913,#14914));
#3735=EDGE_LOOP('',(#14915,#14916,#14917,#14918,#14919,#14920,#14921,#14922,
#14923,#14924));
#3736=EDGE_LOOP('',(#14925));
#4676=LINE('',#40643,#5987);
#4677=LINE('',#40670,#5988);
#4678=LINE('',#40718,#5989);
#4679=LINE('',#40766,#5990);
#4680=LINE('',#40814,#5991);
#4681=LINE('',#40868,#5992);
#4682=LINE('',#40916,#5993);
#4683=LINE('',#40964,#5994);
#4684=LINE('',#41018,#5995);
#4685=LINE('',#41066,#5996);
#4686=LINE('',#41114,#5997);
#4687=LINE('',#41162,#5998);
#4688=LINE('',#41216,#5999);
#4689=LINE('',#41264,#6000);
#4690=LINE('',#41289,#6001);
#4691=LINE('',#41314,#6002);
#4692=LINE('',#41339,#6003);
#4693=LINE('',#41363,#6004);
#4694=LINE('',#41387,#6005);
#4695=LINE('',#41412,#6006);
#4696=LINE('',#41437,#6007);
#4697=LINE('',#41461,#6008);
#4698=LINE('',#41486,#6009);
#4699=LINE('',#41511,#6010);
#4700=LINE('',#41535,#6011);
#4701=LINE('',#42741,#6012);
#4702=LINE('',#42746,#6013);
#4703=LINE('',#42758,#6014);
#4704=LINE('',#42773,#6015);
#4705=LINE('',#42788,#6016);
#4706=LINE('',#42803,#6017);
#4707=LINE('',#42818,#6018);
#4708=LINE('',#42833,#6019);
#4709=LINE('',#42848,#6020);
#4710=LINE('',#42863,#6021);
#4711=LINE('',#42878,#6022);
#4712=LINE('',#42898,#6023);
#4713=LINE('',#42900,#6024);
#4714=LINE('',#42902,#6025);
#4715=LINE('',#42903,#6026);
#4716=LINE('',#42906,#6027);
#4717=LINE('',#42908,#6028);
#4718=LINE('',#42909,#6029);
#4719=LINE('',#42912,#6030);
#4720=LINE('',#42914,#6031);
#4721=LINE('',#42915,#6032);
#4722=LINE('',#42918,#6033);
#4723=LINE('',#42920,#6034);
#4724=LINE('',#42921,#6035);
#4725=LINE('',#42924,#6036);
#4726=LINE('',#42926,#6037);
#4727=LINE('',#42927,#6038);
#4728=LINE('',#42930,#6039);
#4729=LINE('',#42932,#6040);
#4730=LINE('',#42933,#6041);
#4731=LINE('',#42936,#6042);
#4732=LINE('',#42938,#6043);
#4733=LINE('',#42939,#6044);
#4734=LINE('',#42942,#6045);
#4735=LINE('',#42944,#6046);
#4736=LINE('',#42945,#6047);
#4737=LINE('',#42948,#6048);
#4738=LINE('',#42950,#6049);
#4739=LINE('',#42951,#6050);
#4740=LINE('',#42953,#6051);
#4741=LINE('',#42954,#6052);
#4742=LINE('',#42968,#6053);
#4743=LINE('',#42973,#6054);
#4744=LINE('',#42985,#6055);
#4745=LINE('',#43000,#6056);
#4746=LINE('',#43015,#6057);
#4747=LINE('',#43030,#6058);
#4748=LINE('',#43045,#6059);
#4749=LINE('',#43060,#6060);
#4750=LINE('',#43075,#6061);
#4751=LINE('',#43090,#6062);
#4752=LINE('',#43105,#6063);
#4753=LINE('',#43125,#6064);
#4754=LINE('',#43127,#6065);
#4755=LINE('',#43129,#6066);
#4756=LINE('',#43130,#6067);
#4757=LINE('',#43133,#6068);
#4758=LINE('',#43135,#6069);
#4759=LINE('',#43136,#6070);
#4760=LINE('',#43139,#6071);
#4761=LINE('',#43141,#6072);
#4762=LINE('',#43142,#6073);
#4763=LINE('',#43145,#6074);
#4764=LINE('',#43147,#6075);
#4765=LINE('',#43148,#6076);
#4766=LINE('',#43151,#6077);
#4767=LINE('',#43153,#6078);
#4768=LINE('',#43154,#6079);
#4769=LINE('',#43157,#6080);
#4770=LINE('',#43159,#6081);
#4771=LINE('',#43160,#6082);
#4772=LINE('',#43163,#6083);
#4773=LINE('',#43165,#6084);
#4774=LINE('',#43166,#6085);
#4775=LINE('',#43169,#6086);
#4776=LINE('',#43171,#6087);
#4777=LINE('',#43172,#6088);
#4778=LINE('',#43175,#6089);
#4779=LINE('',#43177,#6090);
#4780=LINE('',#43178,#6091);
#4781=LINE('',#43180,#6092);
#4782=LINE('',#43181,#6093);
#4783=LINE('',#43186,#6094);
#4784=LINE('',#43188,#6095);
#4785=LINE('',#43190,#6096);
#4786=LINE('',#43191,#6097);
#4787=LINE('',#43194,#6098);
#4788=LINE('',#43196,#6099);
#4789=LINE('',#43197,#6100);
#4790=LINE('',#43200,#6101);
#4791=LINE('',#43202,#6102);
#4792=LINE('',#43203,#6103);
#4793=LINE('',#43206,#6104);
#4794=LINE('',#43208,#6105);
#4795=LINE('',#43209,#6106);
#4796=LINE('',#43212,#6107);
#4797=LINE('',#43214,#6108);
#4798=LINE('',#43215,#6109);
#4799=LINE('',#43218,#6110);
#4800=LINE('',#43220,#6111);
#4801=LINE('',#43221,#6112);
#4802=LINE('',#43224,#6113);
#4803=LINE('',#43226,#6114);
#4804=LINE('',#43227,#6115);
#4805=LINE('',#43230,#6116);
#4806=LINE('',#43232,#6117);
#4807=LINE('',#43233,#6118);
#4808=LINE('',#43236,#6119);
#4809=LINE('',#43238,#6120);
#4810=LINE('',#43239,#6121);
#4811=LINE('',#43241,#6122);
#4812=LINE('',#43242,#6123);
#4813=LINE('',#43251,#6124);
#4814=LINE('',#43255,#6125);
#4815=LINE('',#43261,#6126);
#4816=LINE('',#43263,#6127);
#4817=LINE('',#43265,#6128);
#4818=LINE('',#43266,#6129);
#4819=LINE('',#43270,#6130);
#4820=LINE('',#43273,#6131);
#4821=LINE('',#43274,#6132);
#4822=LINE('',#43280,#6133);
#4823=LINE('',#43282,#6134);
#4824=LINE('',#43284,#6135);
#4825=LINE('',#43285,#6136);
#4826=LINE('',#43289,#6137);
#4827=LINE('',#43292,#6138);
#4828=LINE('',#43293,#6139);
#4829=LINE('',#43299,#6140);
#4830=LINE('',#43301,#6141);
#4831=LINE('',#43303,#6142);
#4832=LINE('',#43304,#6143);
#4833=LINE('',#43308,#6144);
#4834=LINE('',#43311,#6145);
#4835=LINE('',#43312,#6146);
#4836=LINE('',#43318,#6147);
#4837=LINE('',#43320,#6148);
#4838=LINE('',#43322,#6149);
#4839=LINE('',#43323,#6150);
#4840=LINE('',#43327,#6151);
#4841=LINE('',#43330,#6152);
#4842=LINE('',#43331,#6153);
#4843=LINE('',#43337,#6154);
#4844=LINE('',#43339,#6155);
#4845=LINE('',#43341,#6156);
#4846=LINE('',#43342,#6157);
#4847=LINE('',#43346,#6158);
#4848=LINE('',#43349,#6159);
#4849=LINE('',#43350,#6160);
#4850=LINE('',#43356,#6161);
#4851=LINE('',#43358,#6162);
#4852=LINE('',#43360,#6163);
#4853=LINE('',#43361,#6164);
#4854=LINE('',#43365,#6165);
#4855=LINE('',#43368,#6166);
#4856=LINE('',#43369,#6167);
#4857=LINE('',#43375,#6168);
#4858=LINE('',#43377,#6169);
#4859=LINE('',#43379,#6170);
#4860=LINE('',#43380,#6171);
#4861=LINE('',#43384,#6172);
#4862=LINE('',#43387,#6173);
#4863=LINE('',#43388,#6174);
#4864=LINE('',#43394,#6175);
#4865=LINE('',#43396,#6176);
#4866=LINE('',#43398,#6177);
#4867=LINE('',#43399,#6178);
#4868=LINE('',#43403,#6179);
#4869=LINE('',#43406,#6180);
#4870=LINE('',#43407,#6181);
#4871=LINE('',#43413,#6182);
#4872=LINE('',#43415,#6183);
#4873=LINE('',#43417,#6184);
#4874=LINE('',#43418,#6185);
#4875=LINE('',#43422,#6186);
#4876=LINE('',#43425,#6187);
#4877=LINE('',#43426,#6188);
#4878=LINE('',#43432,#6189);
#4879=LINE('',#43434,#6190);
#4880=LINE('',#43436,#6191);
#4881=LINE('',#43437,#6192);
#4882=LINE('',#43441,#6193);
#4883=LINE('',#43444,#6194);
#4884=LINE('',#43445,#6195);
#4885=LINE('',#43451,#6196);
#4886=LINE('',#43453,#6197);
#4887=LINE('',#43455,#6198);
#4888=LINE('',#43456,#6199);
#4889=LINE('',#43460,#6200);
#4890=LINE('',#43463,#6201);
#4891=LINE('',#43464,#6202);
#4892=LINE('',#43470,#6203);
#4893=LINE('',#43472,#6204);
#4894=LINE('',#43474,#6205);
#4895=LINE('',#43475,#6206);
#4896=LINE('',#43479,#6207);
#4897=LINE('',#43482,#6208);
#4898=LINE('',#43483,#6209);
#4899=LINE('',#43489,#6210);
#4900=LINE('',#43491,#6211);
#4901=LINE('',#43493,#6212);
#4902=LINE('',#43494,#6213);
#4903=LINE('',#43498,#6214);
#4904=LINE('',#43501,#6215);
#4905=LINE('',#43502,#6216);
#4906=LINE('',#43508,#6217);
#4907=LINE('',#43510,#6218);
#4908=LINE('',#43512,#6219);
#4909=LINE('',#43513,#6220);
#4910=LINE('',#43517,#6221);
#4911=LINE('',#43520,#6222);
#4912=LINE('',#43521,#6223);
#4913=LINE('',#43527,#6224);
#4914=LINE('',#43529,#6225);
#4915=LINE('',#43531,#6226);
#4916=LINE('',#43532,#6227);
#4917=LINE('',#43537,#6228);
#4918=LINE('',#43541,#6229);
#4919=LINE('',#43542,#6230);
#4920=LINE('',#43550,#6231);
#4921=LINE('',#43552,#6232);
#4922=LINE('',#43554,#6233);
#4923=LINE('',#43555,#6234);
#4924=LINE('',#43559,#6235);
#4925=LINE('',#43562,#6236);
#4926=LINE('',#43563,#6237);
#4927=LINE('',#43569,#6238);
#4928=LINE('',#43571,#6239);
#4929=LINE('',#43573,#6240);
#4930=LINE('',#43574,#6241);
#4931=LINE('',#43578,#6242);
#4932=LINE('',#43581,#6243);
#4933=LINE('',#43582,#6244);
#4934=LINE('',#43588,#6245);
#4935=LINE('',#43590,#6246);
#4936=LINE('',#43592,#6247);
#4937=LINE('',#43593,#6248);
#4938=LINE('',#43597,#6249);
#4939=LINE('',#43600,#6250);
#4940=LINE('',#43601,#6251);
#4941=LINE('',#43607,#6252);
#4942=LINE('',#43609,#6253);
#4943=LINE('',#43611,#6254);
#4944=LINE('',#43612,#6255);
#4945=LINE('',#43616,#6256);
#4946=LINE('',#43619,#6257);
#4947=LINE('',#43620,#6258);
#4948=LINE('',#43626,#6259);
#4949=LINE('',#43628,#6260);
#4950=LINE('',#43630,#6261);
#4951=LINE('',#43631,#6262);
#4952=LINE('',#43635,#6263);
#4953=LINE('',#43638,#6264);
#4954=LINE('',#43639,#6265);
#4955=LINE('',#43645,#6266);
#4956=LINE('',#43647,#6267);
#4957=LINE('',#43649,#6268);
#4958=LINE('',#43650,#6269);
#4959=LINE('',#43654,#6270);
#4960=LINE('',#43657,#6271);
#4961=LINE('',#43658,#6272);
#4962=LINE('',#43664,#6273);
#4963=LINE('',#43666,#6274);
#4964=LINE('',#43668,#6275);
#4965=LINE('',#43669,#6276);
#4966=LINE('',#43673,#6277);
#4967=LINE('',#43676,#6278);
#4968=LINE('',#43677,#6279);
#4969=LINE('',#43683,#6280);
#4970=LINE('',#43685,#6281);
#4971=LINE('',#43687,#6282);
#4972=LINE('',#43688,#6283);
#4973=LINE('',#43692,#6284);
#4974=LINE('',#43695,#6285);
#4975=LINE('',#43696,#6286);
#4976=LINE('',#43702,#6287);
#4977=LINE('',#43704,#6288);
#4978=LINE('',#43706,#6289);
#4979=LINE('',#43707,#6290);
#4980=LINE('',#43711,#6291);
#4981=LINE('',#43714,#6292);
#4982=LINE('',#43715,#6293);
#4983=LINE('',#43721,#6294);
#4984=LINE('',#43723,#6295);
#4985=LINE('',#43725,#6296);
#4986=LINE('',#43726,#6297);
#4987=LINE('',#43730,#6298);
#4988=LINE('',#43733,#6299);
#4989=LINE('',#43734,#6300);
#4990=LINE('',#43740,#6301);
#4991=LINE('',#43742,#6302);
#4992=LINE('',#43744,#6303);
#4993=LINE('',#43745,#6304);
#4994=LINE('',#43749,#6305);
#4995=LINE('',#43752,#6306);
#4996=LINE('',#43753,#6307);
#4997=LINE('',#43759,#6308);
#4998=LINE('',#43761,#6309);
#4999=LINE('',#43763,#6310);
#5000=LINE('',#43764,#6311);
#5001=LINE('',#43768,#6312);
#5002=LINE('',#43771,#6313);
#5003=LINE('',#43772,#6314);
#5004=LINE('',#43778,#6315);
#5005=LINE('',#43780,#6316);
#5006=LINE('',#43782,#6317);
#5007=LINE('',#43783,#6318);
#5008=LINE('',#43787,#6319);
#5009=LINE('',#43790,#6320);
#5010=LINE('',#43791,#6321);
#5011=LINE('',#43797,#6322);
#5012=LINE('',#43799,#6323);
#5013=LINE('',#43801,#6324);
#5014=LINE('',#43802,#6325);
#5015=LINE('',#43806,#6326);
#5016=LINE('',#43809,#6327);
#5017=LINE('',#43810,#6328);
#5018=LINE('',#43816,#6329);
#5019=LINE('',#43818,#6330);
#5020=LINE('',#43820,#6331);
#5021=LINE('',#43821,#6332);
#5022=LINE('',#43825,#6333);
#5023=LINE('',#43828,#6334);
#5024=LINE('',#43829,#6335);
#5025=LINE('',#43838,#6336);
#5026=LINE('',#43840,#6337);
#5027=LINE('',#43845,#6338);
#5028=LINE('',#43852,#6339);
#5029=LINE('',#43856,#6340);
#5030=LINE('',#43857,#6341);
#5031=LINE('',#43861,#6342);
#5987=VECTOR('',#20603,5.);
#5988=VECTOR('',#20608,5.);
#5989=VECTOR('',#20611,5.);
#5990=VECTOR('',#20614,5.);
#5991=VECTOR('',#20617,5.);
#5992=VECTOR('',#20620,5.);
#5993=VECTOR('',#20623,5.);
#5994=VECTOR('',#20626,5.);
#5995=VECTOR('',#20629,5.);
#5996=VECTOR('',#20632,5.);
#5997=VECTOR('',#20635,5.);
#5998=VECTOR('',#20638,5.);
#5999=VECTOR('',#20641,5.);
#6000=VECTOR('',#20644,4.372);
#6001=VECTOR('',#20649,4.372);
#6002=VECTOR('',#20652,4.372);
#6003=VECTOR('',#20655,4.372);
#6004=VECTOR('',#20658,4.372);
#6005=VECTOR('',#20661,4.372);
#6006=VECTOR('',#20664,4.372);
#6007=VECTOR('',#20667,4.372);
#6008=VECTOR('',#20670,4.372);
#6009=VECTOR('',#20673,4.372);
#6010=VECTOR('',#20676,4.372);
#6011=VECTOR('',#20679,4.372);
#6012=VECTOR('',#20696,10.);
#6013=VECTOR('',#20697,10.);
#6014=VECTOR('',#20698,10.);
#6015=VECTOR('',#20699,10.);
#6016=VECTOR('',#20700,10.);
#6017=VECTOR('',#20701,10.);
#6018=VECTOR('',#20702,10.);
#6019=VECTOR('',#20703,10.);
#6020=VECTOR('',#20704,10.);
#6021=VECTOR('',#20705,10.);
#6022=VECTOR('',#20706,10.);
#6023=VECTOR('',#20711,10.);
#6024=VECTOR('',#20712,10.);
#6025=VECTOR('',#20713,10.);
#6026=VECTOR('',#20714,10.);
#6027=VECTOR('',#20717,10.);
#6028=VECTOR('',#20718,10.);
#6029=VECTOR('',#20719,10.);
#6030=VECTOR('',#20722,10.);
#6031=VECTOR('',#20723,10.);
#6032=VECTOR('',#20724,10.);
#6033=VECTOR('',#20727,10.);
#6034=VECTOR('',#20728,10.);
#6035=VECTOR('',#20729,10.);
#6036=VECTOR('',#20732,10.);
#6037=VECTOR('',#20733,10.);
#6038=VECTOR('',#20734,10.);
#6039=VECTOR('',#20737,10.);
#6040=VECTOR('',#20738,10.);
#6041=VECTOR('',#20739,10.);
#6042=VECTOR('',#20742,10.);
#6043=VECTOR('',#20743,10.);
#6044=VECTOR('',#20744,10.);
#6045=VECTOR('',#20747,10.);
#6046=VECTOR('',#20748,10.);
#6047=VECTOR('',#20749,10.);
#6048=VECTOR('',#20752,10.);
#6049=VECTOR('',#20753,10.);
#6050=VECTOR('',#20754,10.);
#6051=VECTOR('',#20757,10.);
#6052=VECTOR('',#20758,10.);
#6053=VECTOR('',#20761,10.);
#6054=VECTOR('',#20762,10.);
#6055=VECTOR('',#20763,10.);
#6056=VECTOR('',#20764,10.);
#6057=VECTOR('',#20765,10.);
#6058=VECTOR('',#20766,10.);
#6059=VECTOR('',#20767,10.);
#6060=VECTOR('',#20768,10.);
#6061=VECTOR('',#20769,10.);
#6062=VECTOR('',#20770,10.);
#6063=VECTOR('',#20771,10.);
#6064=VECTOR('',#20776,10.);
#6065=VECTOR('',#20777,10.);
#6066=VECTOR('',#20778,10.);
#6067=VECTOR('',#20779,10.);
#6068=VECTOR('',#20782,10.);
#6069=VECTOR('',#20783,10.);
#6070=VECTOR('',#20784,10.);
#6071=VECTOR('',#20787,10.);
#6072=VECTOR('',#20788,10.);
#6073=VECTOR('',#20789,10.);
#6074=VECTOR('',#20792,10.);
#6075=VECTOR('',#20793,10.);
#6076=VECTOR('',#20794,10.);
#6077=VECTOR('',#20797,10.);
#6078=VECTOR('',#20798,10.);
#6079=VECTOR('',#20799,10.);
#6080=VECTOR('',#20802,10.);
#6081=VECTOR('',#20803,10.);
#6082=VECTOR('',#20804,10.);
#6083=VECTOR('',#20807,10.);
#6084=VECTOR('',#20808,10.);
#6085=VECTOR('',#20809,10.);
#6086=VECTOR('',#20812,10.);
#6087=VECTOR('',#20813,10.);
#6088=VECTOR('',#20814,10.);
#6089=VECTOR('',#20817,10.);
#6090=VECTOR('',#20818,10.);
#6091=VECTOR('',#20819,10.);
#6092=VECTOR('',#20822,10.);
#6093=VECTOR('',#20823,10.);
#6094=VECTOR('',#20828,10.);
#6095=VECTOR('',#20829,10.);
#6096=VECTOR('',#20830,10.);
#6097=VECTOR('',#20831,10.);
#6098=VECTOR('',#20834,10.);
#6099=VECTOR('',#20835,10.);
#6100=VECTOR('',#20836,10.);
#6101=VECTOR('',#20839,10.);
#6102=VECTOR('',#20840,10.);
#6103=VECTOR('',#20841,10.);
#6104=VECTOR('',#20844,10.);
#6105=VECTOR('',#20845,10.);
#6106=VECTOR('',#20846,10.);
#6107=VECTOR('',#20849,10.);
#6108=VECTOR('',#20850,10.);
#6109=VECTOR('',#20851,10.);
#6110=VECTOR('',#20854,10.);
#6111=VECTOR('',#20855,10.);
#6112=VECTOR('',#20856,10.);
#6113=VECTOR('',#20859,10.);
#6114=VECTOR('',#20860,10.);
#6115=VECTOR('',#20861,10.);
#6116=VECTOR('',#20864,10.);
#6117=VECTOR('',#20865,10.);
#6118=VECTOR('',#20866,10.);
#6119=VECTOR('',#20869,10.);
#6120=VECTOR('',#20870,10.);
#6121=VECTOR('',#20871,10.);
#6122=VECTOR('',#20874,10.);
#6123=VECTOR('',#20875,10.);
#6124=VECTOR('',#20886,3.6);
#6125=VECTOR('',#20891,3.);
#6126=VECTOR('',#20898,10.);
#6127=VECTOR('',#20899,10.);
#6128=VECTOR('',#20900,10.);
#6129=VECTOR('',#20901,10.);
#6130=VECTOR('',#20906,10.);
#6131=VECTOR('',#20909,10.);
#6132=VECTOR('',#20910,10.);
#6133=VECTOR('',#20917,10.);
#6134=VECTOR('',#20918,10.);
#6135=VECTOR('',#20919,10.);
#6136=VECTOR('',#20920,10.);
#6137=VECTOR('',#20925,10.);
#6138=VECTOR('',#20928,10.);
#6139=VECTOR('',#20929,10.);
#6140=VECTOR('',#20936,10.);
#6141=VECTOR('',#20937,10.);
#6142=VECTOR('',#20938,10.);
#6143=VECTOR('',#20939,10.);
#6144=VECTOR('',#20944,10.);
#6145=VECTOR('',#20947,10.);
#6146=VECTOR('',#20948,10.);
#6147=VECTOR('',#20955,10.);
#6148=VECTOR('',#20956,10.);
#6149=VECTOR('',#20957,10.);
#6150=VECTOR('',#20958,10.);
#6151=VECTOR('',#20963,10.);
#6152=VECTOR('',#20966,10.);
#6153=VECTOR('',#20967,10.);
#6154=VECTOR('',#20974,10.);
#6155=VECTOR('',#20975,10.);
#6156=VECTOR('',#20976,10.);
#6157=VECTOR('',#20977,10.);
#6158=VECTOR('',#20982,10.);
#6159=VECTOR('',#20985,10.);
#6160=VECTOR('',#20986,10.);
#6161=VECTOR('',#20993,10.);
#6162=VECTOR('',#20994,10.);
#6163=VECTOR('',#20995,10.);
#6164=VECTOR('',#20996,10.);
#6165=VECTOR('',#21001,10.);
#6166=VECTOR('',#21004,10.);
#6167=VECTOR('',#21005,10.);
#6168=VECTOR('',#21012,10.);
#6169=VECTOR('',#21013,10.);
#6170=VECTOR('',#21014,10.);
#6171=VECTOR('',#21015,10.);
#6172=VECTOR('',#21020,10.);
#6173=VECTOR('',#21023,10.);
#6174=VECTOR('',#21024,10.);
#6175=VECTOR('',#21031,10.);
#6176=VECTOR('',#21032,10.);
#6177=VECTOR('',#21033,10.);
#6178=VECTOR('',#21034,10.);
#6179=VECTOR('',#21039,10.);
#6180=VECTOR('',#21042,10.);
#6181=VECTOR('',#21043,10.);
#6182=VECTOR('',#21050,10.);
#6183=VECTOR('',#21051,10.);
#6184=VECTOR('',#21052,10.);
#6185=VECTOR('',#21053,10.);
#6186=VECTOR('',#21058,10.);
#6187=VECTOR('',#21061,10.);
#6188=VECTOR('',#21062,10.);
#6189=VECTOR('',#21069,10.);
#6190=VECTOR('',#21070,10.);
#6191=VECTOR('',#21071,10.);
#6192=VECTOR('',#21072,10.);
#6193=VECTOR('',#21077,10.);
#6194=VECTOR('',#21080,10.);
#6195=VECTOR('',#21081,10.);
#6196=VECTOR('',#21088,10.);
#6197=VECTOR('',#21089,10.);
#6198=VECTOR('',#21090,10.);
#6199=VECTOR('',#21091,10.);
#6200=VECTOR('',#21096,10.);
#6201=VECTOR('',#21099,10.);
#6202=VECTOR('',#21100,10.);
#6203=VECTOR('',#21107,10.);
#6204=VECTOR('',#21108,10.);
#6205=VECTOR('',#21109,10.);
#6206=VECTOR('',#21110,10.);
#6207=VECTOR('',#21115,10.);
#6208=VECTOR('',#21118,10.);
#6209=VECTOR('',#21119,10.);
#6210=VECTOR('',#21126,10.);
#6211=VECTOR('',#21127,10.);
#6212=VECTOR('',#21128,10.);
#6213=VECTOR('',#21129,10.);
#6214=VECTOR('',#21134,10.);
#6215=VECTOR('',#21137,10.);
#6216=VECTOR('',#21138,10.);
#6217=VECTOR('',#21145,10.);
#6218=VECTOR('',#21146,10.);
#6219=VECTOR('',#21147,10.);
#6220=VECTOR('',#21148,10.);
#6221=VECTOR('',#21153,10.);
#6222=VECTOR('',#21156,10.);
#6223=VECTOR('',#21157,10.);
#6224=VECTOR('',#21164,10.);
#6225=VECTOR('',#21165,10.);
#6226=VECTOR('',#21166,10.);
#6227=VECTOR('',#21167,10.);
#6228=VECTOR('',#21172,10.);
#6229=VECTOR('',#21177,10.);
#6230=VECTOR('',#21178,10.);
#6231=VECTOR('',#21187,10.);
#6232=VECTOR('',#21188,10.);
#6233=VECTOR('',#21189,10.);
#6234=VECTOR('',#21190,10.);
#6235=VECTOR('',#21195,10.);
#6236=VECTOR('',#21198,10.);
#6237=VECTOR('',#21199,10.);
#6238=VECTOR('',#21206,10.);
#6239=VECTOR('',#21207,10.);
#6240=VECTOR('',#21208,10.);
#6241=VECTOR('',#21209,10.);
#6242=VECTOR('',#21214,10.);
#6243=VECTOR('',#21217,10.);
#6244=VECTOR('',#21218,10.);
#6245=VECTOR('',#21225,10.);
#6246=VECTOR('',#21226,10.);
#6247=VECTOR('',#21227,10.);
#6248=VECTOR('',#21228,10.);
#6249=VECTOR('',#21233,10.);
#6250=VECTOR('',#21236,10.);
#6251=VECTOR('',#21237,10.);
#6252=VECTOR('',#21244,10.);
#6253=VECTOR('',#21245,10.);
#6254=VECTOR('',#21246,10.);
#6255=VECTOR('',#21247,10.);
#6256=VECTOR('',#21252,10.);
#6257=VECTOR('',#21255,10.);
#6258=VECTOR('',#21256,10.);
#6259=VECTOR('',#21263,10.);
#6260=VECTOR('',#21264,10.);
#6261=VECTOR('',#21265,10.);
#6262=VECTOR('',#21266,10.);
#6263=VECTOR('',#21271,10.);
#6264=VECTOR('',#21274,10.);
#6265=VECTOR('',#21275,10.);
#6266=VECTOR('',#21282,10.);
#6267=VECTOR('',#21283,10.);
#6268=VECTOR('',#21284,10.);
#6269=VECTOR('',#21285,10.);
#6270=VECTOR('',#21290,10.);
#6271=VECTOR('',#21293,10.);
#6272=VECTOR('',#21294,10.);
#6273=VECTOR('',#21301,10.);
#6274=VECTOR('',#21302,10.);
#6275=VECTOR('',#21303,10.);
#6276=VECTOR('',#21304,10.);
#6277=VECTOR('',#21309,10.);
#6278=VECTOR('',#21312,10.);
#6279=VECTOR('',#21313,10.);
#6280=VECTOR('',#21320,10.);
#6281=VECTOR('',#21321,10.);
#6282=VECTOR('',#21322,10.);
#6283=VECTOR('',#21323,10.);
#6284=VECTOR('',#21328,10.);
#6285=VECTOR('',#21331,10.);
#6286=VECTOR('',#21332,10.);
#6287=VECTOR('',#21339,10.);
#6288=VECTOR('',#21340,10.);
#6289=VECTOR('',#21341,10.);
#6290=VECTOR('',#21342,10.);
#6291=VECTOR('',#21347,10.);
#6292=VECTOR('',#21350,10.);
#6293=VECTOR('',#21351,10.);
#6294=VECTOR('',#21358,10.);
#6295=VECTOR('',#21359,10.);
#6296=VECTOR('',#21360,10.);
#6297=VECTOR('',#21361,10.);
#6298=VECTOR('',#21366,10.);
#6299=VECTOR('',#21369,10.);
#6300=VECTOR('',#21370,10.);
#6301=VECTOR('',#21377,10.);
#6302=VECTOR('',#21378,10.);
#6303=VECTOR('',#21379,10.);
#6304=VECTOR('',#21380,10.);
#6305=VECTOR('',#21385,10.);
#6306=VECTOR('',#21388,10.);
#6307=VECTOR('',#21389,10.);
#6308=VECTOR('',#21396,10.);
#6309=VECTOR('',#21397,10.);
#6310=VECTOR('',#21398,10.);
#6311=VECTOR('',#21399,10.);
#6312=VECTOR('',#21404,10.);
#6313=VECTOR('',#21407,10.);
#6314=VECTOR('',#21408,10.);
#6315=VECTOR('',#21415,10.);
#6316=VECTOR('',#21416,10.);
#6317=VECTOR('',#21417,10.);
#6318=VECTOR('',#21418,10.);
#6319=VECTOR('',#21423,10.);
#6320=VECTOR('',#21426,10.);
#6321=VECTOR('',#21427,10.);
#6322=VECTOR('',#21434,10.);
#6323=VECTOR('',#21435,10.);
#6324=VECTOR('',#21436,10.);
#6325=VECTOR('',#21437,10.);
#6326=VECTOR('',#21442,10.);
#6327=VECTOR('',#21445,10.);
#6328=VECTOR('',#21446,10.);
#6329=VECTOR('',#21453,10.);
#6330=VECTOR('',#21454,10.);
#6331=VECTOR('',#21455,10.);
#6332=VECTOR('',#21456,10.);
#6333=VECTOR('',#21461,10.);
#6334=VECTOR('',#21464,10.);
#6335=VECTOR('',#21465,10.);
#6336=VECTOR('',#21478,3.);
#6337=VECTOR('',#21481,4.75);
#6338=VECTOR('',#21488,4.);
#6339=VECTOR('',#21497,12.7);
#6340=VECTOR('',#21502,13.);
#6341=VECTOR('',#21503,13.);
#6342=VECTOR('',#21508,12.7);
#6800=CIRCLE('',#17603,4.942);
#6801=CIRCLE('',#17617,4.372);
#6802=CIRCLE('',#17630,4.942);
#6803=CIRCLE('',#17631,4.942);
#6804=CIRCLE('',#17632,4.372);
#6805=CIRCLE('',#17635,4.942);
#6806=CIRCLE('',#17636,4.);
#6807=CIRCLE('',#17673,3.6);
#6808=CIRCLE('',#17674,3.);
#6809=CIRCLE('',#17676,3.6);
#6810=CIRCLE('',#17678,3.);
#6811=CIRCLE('',#17682,13.);
#6812=CIRCLE('',#17685,13.);
#6813=CIRCLE('',#17688,13.);
#6814=CIRCLE('',#17691,13.);
#6815=CIRCLE('',#17694,13.);
#6816=CIRCLE('',#17697,13.);
#6817=CIRCLE('',#17700,13.);
#6818=CIRCLE('',#17703,13.);
#6819=CIRCLE('',#17706,13.);
#6820=CIRCLE('',#17709,13.);
#6821=CIRCLE('',#17712,13.);
#6822=CIRCLE('',#17715,13.);
#6823=CIRCLE('',#17718,13.);
#6824=CIRCLE('',#17721,13.);
#6825=CIRCLE('',#17724,13.);
#6826=CIRCLE('',#17727,13.);
#6827=CIRCLE('',#17730,13.);
#6828=CIRCLE('',#17733,13.);
#6829=CIRCLE('',#17736,13.);
#6830=CIRCLE('',#17739,13.);
#6831=CIRCLE('',#17742,13.);
#6832=CIRCLE('',#17745,13.);
#6833=CIRCLE('',#17748,13.);
#6834=CIRCLE('',#17751,13.);
#6835=CIRCLE('',#17754,13.);
#6836=CIRCLE('',#17757,13.);
#6837=CIRCLE('',#17760,13.);
#6838=CIRCLE('',#17763,13.);
#6839=CIRCLE('',#17766,13.);
#6840=CIRCLE('',#17767,13.);
#6841=CIRCLE('',#17770,13.);
#6842=CIRCLE('',#17771,13.);
#6843=CIRCLE('',#17774,13.);
#6844=CIRCLE('',#17777,13.);
#6845=CIRCLE('',#17780,13.);
#6846=CIRCLE('',#17783,13.);
#6847=CIRCLE('',#17786,13.);
#6848=CIRCLE('',#17789,13.);
#6849=CIRCLE('',#17792,13.);
#6850=CIRCLE('',#17795,13.);
#6851=CIRCLE('',#17798,13.);
#6852=CIRCLE('',#17801,13.);
#6853=CIRCLE('',#17804,13.);
#6854=CIRCLE('',#17807,13.);
#6855=CIRCLE('',#17810,13.);
#6856=CIRCLE('',#17813,13.);
#6857=CIRCLE('',#17816,13.);
#6858=CIRCLE('',#17819,13.);
#6859=CIRCLE('',#17822,13.);
#6860=CIRCLE('',#17825,13.);
#6861=CIRCLE('',#17828,13.);
#6862=CIRCLE('',#17831,13.);
#6863=CIRCLE('',#17834,13.);
#6864=CIRCLE('',#17837,13.);
#6865=CIRCLE('',#17840,13.);
#6866=CIRCLE('',#17843,13.);
#6867=CIRCLE('',#17846,13.);
#6868=CIRCLE('',#17849,13.);
#6869=CIRCLE('',#17852,13.);
#6870=CIRCLE('',#17855,13.);
#6871=CIRCLE('',#17858,13.);
#6872=CIRCLE('',#17861,13.);
#6873=CIRCLE('',#17863,1.5);
#6874=CIRCLE('',#17865,4.5);
#6875=CIRCLE('',#17869,4.);
#6876=CIRCLE('',#17871,12.4);
#6877=CIRCLE('',#17873,13.);
#6878=CIRCLE('',#17875,13.);
#6879=CIRCLE('',#17877,12.4);
#7942=VERTEX_POINT('',#40641);
#7943=VERTEX_POINT('',#40642);
#7944=VERTEX_POINT('',#40644);
#7945=VERTEX_POINT('',#40655);
#7946=VERTEX_POINT('',#40668);
#7947=VERTEX_POINT('',#40669);
#7948=VERTEX_POINT('',#40716);
#7949=VERTEX_POINT('',#40717);
#7950=VERTEX_POINT('',#40764);
#7951=VERTEX_POINT('',#40765);
#7952=VERTEX_POINT('',#40812);
#7953=VERTEX_POINT('',#40813);
#7954=VERTEX_POINT('',#40866);
#7955=VERTEX_POINT('',#40867);
#7956=VERTEX_POINT('',#40914);
#7957=VERTEX_POINT('',#40915);
#7958=VERTEX_POINT('',#40962);
#7959=VERTEX_POINT('',#40963);
#7960=VERTEX_POINT('',#41016);
#7961=VERTEX_POINT('',#41017);
#7962=VERTEX_POINT('',#41064);
#7963=VERTEX_POINT('',#41065);
#7964=VERTEX_POINT('',#41112);
#7965=VERTEX_POINT('',#41113);
#7966=VERTEX_POINT('',#41160);
#7967=VERTEX_POINT('',#41161);
#7968=VERTEX_POINT('',#41214);
#7969=VERTEX_POINT('',#41215);
#7970=VERTEX_POINT('',#41262);
#7971=VERTEX_POINT('',#41263);
#7972=VERTEX_POINT('',#41265);
#7973=VERTEX_POINT('',#41275);
#7974=VERTEX_POINT('',#41287);
#7975=VERTEX_POINT('',#41288);
#7976=VERTEX_POINT('',#41312);
#7977=VERTEX_POINT('',#41313);
#7978=VERTEX_POINT('',#41337);
#7979=VERTEX_POINT('',#41338);
#7980=VERTEX_POINT('',#41361);
#7981=VERTEX_POINT('',#41362);
#7982=VERTEX_POINT('',#41385);
#7983=VERTEX_POINT('',#41386);
#7984=VERTEX_POINT('',#41410);
#7985=VERTEX_POINT('',#41411);
#7986=VERTEX_POINT('',#41435);
#7987=VERTEX_POINT('',#41436);
#7988=VERTEX_POINT('',#41459);
#7989=VERTEX_POINT('',#41460);
#7990=VERTEX_POINT('',#41484);
#7991=VERTEX_POINT('',#41485);
#7992=VERTEX_POINT('',#41509);
#7993=VERTEX_POINT('',#41510);
#7994=VERTEX_POINT('',#41533);
#7995=VERTEX_POINT('',#41534);
#7996=VERTEX_POINT('',#41900);
#7997=VERTEX_POINT('',#42017);
#7998=VERTEX_POINT('',#42134);
#7999=VERTEX_POINT('',#42137);
#8000=VERTEX_POINT('',#42605);
#8001=VERTEX_POINT('',#42727);
#8002=VERTEX_POINT('',#42735);
#8003=VERTEX_POINT('',#42736);
#8004=VERTEX_POINT('',#42740);
#8005=VERTEX_POINT('',#42742);
#8006=VERTEX_POINT('',#42753);
#8007=VERTEX_POINT('',#42757);
#8008=VERTEX_POINT('',#42768);
#8009=VERTEX_POINT('',#42772);
#8010=VERTEX_POINT('',#42783);
#8011=VERTEX_POINT('',#42787);
#8012=VERTEX_POINT('',#42798);
#8013=VERTEX_POINT('',#42802);
#8014=VERTEX_POINT('',#42813);
#8015=VERTEX_POINT('',#42817);
#8016=VERTEX_POINT('',#42828);
#8017=VERTEX_POINT('',#42832);
#8018=VERTEX_POINT('',#42843);
#8019=VERTEX_POINT('',#42847);
#8020=VERTEX_POINT('',#42858);
#8021=VERTEX_POINT('',#42862);
#8022=VERTEX_POINT('',#42873);
#8023=VERTEX_POINT('',#42877);
#8024=VERTEX_POINT('',#42896);
#8025=VERTEX_POINT('',#42897);
#8026=VERTEX_POINT('',#42899);
#8027=VERTEX_POINT('',#42901);
#8028=VERTEX_POINT('',#42905);
#8029=VERTEX_POINT('',#42907);
#8030=VERTEX_POINT('',#42911);
#8031=VERTEX_POINT('',#42913);
#8032=VERTEX_POINT('',#42917);
#8033=VERTEX_POINT('',#42919);
#8034=VERTEX_POINT('',#42923);
#8035=VERTEX_POINT('',#42925);
#8036=VERTEX_POINT('',#42929);
#8037=VERTEX_POINT('',#42931);
#8038=VERTEX_POINT('',#42935);
#8039=VERTEX_POINT('',#42937);
#8040=VERTEX_POINT('',#42941);
#8041=VERTEX_POINT('',#42943);
#8042=VERTEX_POINT('',#42947);
#8043=VERTEX_POINT('',#42949);
#8044=VERTEX_POINT('',#42962);
#8045=VERTEX_POINT('',#42963);
#8046=VERTEX_POINT('',#42967);
#8047=VERTEX_POINT('',#42969);
#8048=VERTEX_POINT('',#42980);
#8049=VERTEX_POINT('',#42984);
#8050=VERTEX_POINT('',#42995);
#8051=VERTEX_POINT('',#42999);
#8052=VERTEX_POINT('',#43010);
#8053=VERTEX_POINT('',#43014);
#8054=VERTEX_POINT('',#43025);
#8055=VERTEX_POINT('',#43029);
#8056=VERTEX_POINT('',#43040);
#8057=VERTEX_POINT('',#43044);
#8058=VERTEX_POINT('',#43055);
#8059=VERTEX_POINT('',#43059);
#8060=VERTEX_POINT('',#43070);
#8061=VERTEX_POINT('',#43074);
#8062=VERTEX_POINT('',#43085);
#8063=VERTEX_POINT('',#43089);
#8064=VERTEX_POINT('',#43100);
#8065=VERTEX_POINT('',#43104);
#8066=VERTEX_POINT('',#43123);
#8067=VERTEX_POINT('',#43124);
#8068=VERTEX_POINT('',#43126);
#8069=VERTEX_POINT('',#43128);
#8070=VERTEX_POINT('',#43132);
#8071=VERTEX_POINT('',#43134);
#8072=VERTEX_POINT('',#43138);
#8073=VERTEX_POINT('',#43140);
#8074=VERTEX_POINT('',#43144);
#8075=VERTEX_POINT('',#43146);
#8076=VERTEX_POINT('',#43150);
#8077=VERTEX_POINT('',#43152);
#8078=VERTEX_POINT('',#43156);
#8079=VERTEX_POINT('',#43158);
#8080=VERTEX_POINT('',#43162);
#8081=VERTEX_POINT('',#43164);
#8082=VERTEX_POINT('',#43168);
#8083=VERTEX_POINT('',#43170);
#8084=VERTEX_POINT('',#43174);
#8085=VERTEX_POINT('',#43176);
#8086=VERTEX_POINT('',#43184);
#8087=VERTEX_POINT('',#43185);
#8088=VERTEX_POINT('',#43187);
#8089=VERTEX_POINT('',#43189);
#8090=VERTEX_POINT('',#43193);
#8091=VERTEX_POINT('',#43195);
#8092=VERTEX_POINT('',#43199);
#8093=VERTEX_POINT('',#43201);
#8094=VERTEX_POINT('',#43205);
#8095=VERTEX_POINT('',#43207);
#8096=VERTEX_POINT('',#43211);
#8097=VERTEX_POINT('',#43213);
#8098=VERTEX_POINT('',#43217);
#8099=VERTEX_POINT('',#43219);
#8100=VERTEX_POINT('',#43223);
#8101=VERTEX_POINT('',#43225);
#8102=VERTEX_POINT('',#43229);
#8103=VERTEX_POINT('',#43231);
#8104=VERTEX_POINT('',#43235);
#8105=VERTEX_POINT('',#43237);
#8106=VERTEX_POINT('',#43245);
#8107=VERTEX_POINT('',#43247);
#8108=VERTEX_POINT('',#43250);
#8109=VERTEX_POINT('',#43254);
#8110=VERTEX_POINT('',#43259);
#8111=VERTEX_POINT('',#43260);
#8112=VERTEX_POINT('',#43262);
#8113=VERTEX_POINT('',#43264);
#8114=VERTEX_POINT('',#43268);
#8115=VERTEX_POINT('',#43272);
#8116=VERTEX_POINT('',#43278);
#8117=VERTEX_POINT('',#43279);
#8118=VERTEX_POINT('',#43281);
#8119=VERTEX_POINT('',#43283);
#8120=VERTEX_POINT('',#43287);
#8121=VERTEX_POINT('',#43291);
#8122=VERTEX_POINT('',#43297);
#8123=VERTEX_POINT('',#43298);
#8124=VERTEX_POINT('',#43300);
#8125=VERTEX_POINT('',#43302);
#8126=VERTEX_POINT('',#43306);
#8127=VERTEX_POINT('',#43310);
#8128=VERTEX_POINT('',#43316);
#8129=VERTEX_POINT('',#43317);
#8130=VERTEX_POINT('',#43319);
#8131=VERTEX_POINT('',#43321);
#8132=VERTEX_POINT('',#43325);
#8133=VERTEX_POINT('',#43329);
#8134=VERTEX_POINT('',#43335);
#8135=VERTEX_POINT('',#43336);
#8136=VERTEX_POINT('',#43338);
#8137=VERTEX_POINT('',#43340);
#8138=VERTEX_POINT('',#43344);
#8139=VERTEX_POINT('',#43348);
#8140=VERTEX_POINT('',#43354);
#8141=VERTEX_POINT('',#43355);
#8142=VERTEX_POINT('',#43357);
#8143=VERTEX_POINT('',#43359);
#8144=VERTEX_POINT('',#43363);
#8145=VERTEX_POINT('',#43367);
#8146=VERTEX_POINT('',#43373);
#8147=VERTEX_POINT('',#43374);
#8148=VERTEX_POINT('',#43376);
#8149=VERTEX_POINT('',#43378);
#8150=VERTEX_POINT('',#43382);
#8151=VERTEX_POINT('',#43386);
#8152=VERTEX_POINT('',#43392);
#8153=VERTEX_POINT('',#43393);
#8154=VERTEX_POINT('',#43395);
#8155=VERTEX_POINT('',#43397);
#8156=VERTEX_POINT('',#43401);
#8157=VERTEX_POINT('',#43405);
#8158=VERTEX_POINT('',#43411);
#8159=VERTEX_POINT('',#43412);
#8160=VERTEX_POINT('',#43414);
#8161=VERTEX_POINT('',#43416);
#8162=VERTEX_POINT('',#43420);
#8163=VERTEX_POINT('',#43424);
#8164=VERTEX_POINT('',#43430);
#8165=VERTEX_POINT('',#43431);
#8166=VERTEX_POINT('',#43433);
#8167=VERTEX_POINT('',#43435);
#8168=VERTEX_POINT('',#43439);
#8169=VERTEX_POINT('',#43443);
#8170=VERTEX_POINT('',#43449);
#8171=VERTEX_POINT('',#43450);
#8172=VERTEX_POINT('',#43452);
#8173=VERTEX_POINT('',#43454);
#8174=VERTEX_POINT('',#43458);
#8175=VERTEX_POINT('',#43462);
#8176=VERTEX_POINT('',#43468);
#8177=VERTEX_POINT('',#43469);
#8178=VERTEX_POINT('',#43471);
#8179=VERTEX_POINT('',#43473);
#8180=VERTEX_POINT('',#43477);
#8181=VERTEX_POINT('',#43481);
#8182=VERTEX_POINT('',#43487);
#8183=VERTEX_POINT('',#43488);
#8184=VERTEX_POINT('',#43490);
#8185=VERTEX_POINT('',#43492);
#8186=VERTEX_POINT('',#43496);
#8187=VERTEX_POINT('',#43500);
#8188=VERTEX_POINT('',#43506);
#8189=VERTEX_POINT('',#43507);
#8190=VERTEX_POINT('',#43509);
#8191=VERTEX_POINT('',#43511);
#8192=VERTEX_POINT('',#43515);
#8193=VERTEX_POINT('',#43519);
#8194=VERTEX_POINT('',#43525);
#8195=VERTEX_POINT('',#43526);
#8196=VERTEX_POINT('',#43528);
#8197=VERTEX_POINT('',#43530);
#8198=VERTEX_POINT('',#43534);
#8199=VERTEX_POINT('',#43536);
#8200=VERTEX_POINT('',#43540);
#8201=VERTEX_POINT('',#43544);
#8202=VERTEX_POINT('',#43548);
#8203=VERTEX_POINT('',#43549);
#8204=VERTEX_POINT('',#43551);
#8205=VERTEX_POINT('',#43553);
#8206=VERTEX_POINT('',#43557);
#8207=VERTEX_POINT('',#43561);
#8208=VERTEX_POINT('',#43567);
#8209=VERTEX_POINT('',#43568);
#8210=VERTEX_POINT('',#43570);
#8211=VERTEX_POINT('',#43572);
#8212=VERTEX_POINT('',#43576);
#8213=VERTEX_POINT('',#43580);
#8214=VERTEX_POINT('',#43586);
#8215=VERTEX_POINT('',#43587);
#8216=VERTEX_POINT('',#43589);
#8217=VERTEX_POINT('',#43591);
#8218=VERTEX_POINT('',#43595);
#8219=VERTEX_POINT('',#43599);
#8220=VERTEX_POINT('',#43605);
#8221=VERTEX_POINT('',#43606);
#8222=VERTEX_POINT('',#43608);
#8223=VERTEX_POINT('',#43610);
#8224=VERTEX_POINT('',#43614);
#8225=VERTEX_POINT('',#43618);
#8226=VERTEX_POINT('',#43624);
#8227=VERTEX_POINT('',#43625);
#8228=VERTEX_POINT('',#43627);
#8229=VERTEX_POINT('',#43629);
#8230=VERTEX_POINT('',#43633);
#8231=VERTEX_POINT('',#43637);
#8232=VERTEX_POINT('',#43643);
#8233=VERTEX_POINT('',#43644);
#8234=VERTEX_POINT('',#43646);
#8235=VERTEX_POINT('',#43648);
#8236=VERTEX_POINT('',#43652);
#8237=VERTEX_POINT('',#43656);
#8238=VERTEX_POINT('',#43662);
#8239=VERTEX_POINT('',#43663);
#8240=VERTEX_POINT('',#43665);
#8241=VERTEX_POINT('',#43667);
#8242=VERTEX_POINT('',#43671);
#8243=VERTEX_POINT('',#43675);
#8244=VERTEX_POINT('',#43681);
#8245=VERTEX_POINT('',#43682);
#8246=VERTEX_POINT('',#43684);
#8247=VERTEX_POINT('',#43686);
#8248=VERTEX_POINT('',#43690);
#8249=VERTEX_POINT('',#43694);
#8250=VERTEX_POINT('',#43700);
#8251=VERTEX_POINT('',#43701);
#8252=VERTEX_POINT('',#43703);
#8253=VERTEX_POINT('',#43705);
#8254=VERTEX_POINT('',#43709);
#8255=VERTEX_POINT('',#43713);
#8256=VERTEX_POINT('',#43719);
#8257=VERTEX_POINT('',#43720);
#8258=VERTEX_POINT('',#43722);
#8259=VERTEX_POINT('',#43724);
#8260=VERTEX_POINT('',#43728);
#8261=VERTEX_POINT('',#43732);
#8262=VERTEX_POINT('',#43738);
#8263=VERTEX_POINT('',#43739);
#8264=VERTEX_POINT('',#43741);
#8265=VERTEX_POINT('',#43743);
#8266=VERTEX_POINT('',#43747);
#8267=VERTEX_POINT('',#43751);
#8268=VERTEX_POINT('',#43757);
#8269=VERTEX_POINT('',#43758);
#8270=VERTEX_POINT('',#43760);
#8271=VERTEX_POINT('',#43762);
#8272=VERTEX_POINT('',#43766);
#8273=VERTEX_POINT('',#43770);
#8274=VERTEX_POINT('',#43776);
#8275=VERTEX_POINT('',#43777);
#8276=VERTEX_POINT('',#43779);
#8277=VERTEX_POINT('',#43781);
#8278=VERTEX_POINT('',#43785);
#8279=VERTEX_POINT('',#43789);
#8280=VERTEX_POINT('',#43795);
#8281=VERTEX_POINT('',#43796);
#8282=VERTEX_POINT('',#43798);
#8283=VERTEX_POINT('',#43800);
#8284=VERTEX_POINT('',#43804);
#8285=VERTEX_POINT('',#43808);
#8286=VERTEX_POINT('',#43814);
#8287=VERTEX_POINT('',#43815);
#8288=VERTEX_POINT('',#43817);
#8289=VERTEX_POINT('',#43819);
#8290=VERTEX_POINT('',#43823);
#8291=VERTEX_POINT('',#43827);
#8292=VERTEX_POINT('',#43833);
#8293=VERTEX_POINT('',#43836);
#8294=VERTEX_POINT('',#43843);
#8295=VERTEX_POINT('',#43847);
#8296=VERTEX_POINT('',#43850);
#8297=VERTEX_POINT('',#43854);
#8298=VERTEX_POINT('',#43859);
#9988=EDGE_CURVE('',#7942,#7943,#4676,.T.);
#9989=EDGE_CURVE('',#7942,#7944,#688,.T.);
#9990=EDGE_CURVE('',#7944,#7945,#6800,.T.);
#9991=EDGE_CURVE('',#7945,#7943,#689,.T.);
#9992=EDGE_CURVE('',#7946,#7947,#4677,.T.);
#9993=EDGE_CURVE('',#7946,#7942,#690,.T.);
#9994=EDGE_CURVE('',#7943,#7947,#691,.T.);
#9995=EDGE_CURVE('',#7948,#7949,#4678,.T.);
#9996=EDGE_CURVE('',#7948,#7946,#692,.T.);
#9997=EDGE_CURVE('',#7947,#7949,#693,.T.);
#9998=EDGE_CURVE('',#7950,#7951,#4679,.T.);
#9999=EDGE_CURVE('',#7950,#7948,#694,.T.);
#10000=EDGE_CURVE('',#7949,#7951,#695,.T.);
#10001=EDGE_CURVE('',#7952,#7953,#4680,.T.);
#10002=EDGE_CURVE('',#7952,#7950,#696,.T.);
#10003=EDGE_CURVE('',#7951,#7953,#697,.T.);
#10004=EDGE_CURVE('',#7954,#7955,#4681,.T.);
#10005=EDGE_CURVE('',#7954,#7952,#698,.T.);
#10006=EDGE_CURVE('',#7953,#7955,#699,.T.);
#10007=EDGE_CURVE('',#7956,#7957,#4682,.T.);
#10008=EDGE_CURVE('',#7956,#7954,#700,.T.);
#10009=EDGE_CURVE('',#7955,#7957,#701,.T.);
#10010=EDGE_CURVE('',#7958,#7959,#4683,.T.);
#10011=EDGE_CURVE('',#7958,#7956,#702,.T.);
#10012=EDGE_CURVE('',#7957,#7959,#703,.T.);
#10013=EDGE_CURVE('',#7960,#7961,#4684,.T.);
#10014=EDGE_CURVE('',#7960,#7958,#704,.T.);
#10015=EDGE_CURVE('',#7959,#7961,#705,.T.);
#10016=EDGE_CURVE('',#7962,#7963,#4685,.T.);
#10017=EDGE_CURVE('',#7962,#7960,#706,.T.);
#10018=EDGE_CURVE('',#7961,#7963,#707,.T.);
#10019=EDGE_CURVE('',#7964,#7965,#4686,.T.);
#10020=EDGE_CURVE('',#7964,#7962,#708,.T.);
#10021=EDGE_CURVE('',#7963,#7965,#709,.T.);
#10022=EDGE_CURVE('',#7966,#7967,#4687,.T.);
#10023=EDGE_CURVE('',#7966,#7964,#710,.T.);
#10024=EDGE_CURVE('',#7965,#7967,#711,.T.);
#10025=EDGE_CURVE('',#7968,#7969,#4688,.T.);
#10026=EDGE_CURVE('',#7968,#7966,#712,.T.);
#10027=EDGE_CURVE('',#7967,#7969,#713,.T.);
#10028=EDGE_CURVE('',#7970,#7971,#4689,.T.);
#10029=EDGE_CURVE('',#7970,#7972,#714,.T.);
#10030=EDGE_CURVE('',#7973,#7972,#6801,.T.);
#10031=EDGE_CURVE('',#7971,#7973,#715,.T.);
#10032=EDGE_CURVE('',#7974,#7975,#4690,.T.);
#10033=EDGE_CURVE('',#7974,#7970,#716,.T.);
#10034=EDGE_CURVE('',#7975,#7971,#717,.T.);
#10035=EDGE_CURVE('',#7976,#7977,#4691,.T.);
#10036=EDGE_CURVE('',#7976,#7974,#718,.T.);
#10037=EDGE_CURVE('',#7977,#7975,#719,.T.);
#10038=EDGE_CURVE('',#7978,#7979,#4692,.T.);
#10039=EDGE_CURVE('',#7978,#7976,#720,.T.);
#10040=EDGE_CURVE('',#7979,#7977,#721,.T.);
#10041=EDGE_CURVE('',#7980,#7981,#4693,.T.);
#10042=EDGE_CURVE('',#7980,#7978,#722,.T.);
#10043=EDGE_CURVE('',#7981,#7979,#723,.T.);
#10044=EDGE_CURVE('',#7982,#7983,#4694,.T.);
#10045=EDGE_CURVE('',#7982,#7980,#724,.T.);
#10046=EDGE_CURVE('',#7983,#7981,#725,.T.);
#10047=EDGE_CURVE('',#7984,#7985,#4695,.T.);
#10048=EDGE_CURVE('',#7984,#7982,#726,.T.);
#10049=EDGE_CURVE('',#7985,#7983,#727,.T.);
#10050=EDGE_CURVE('',#7986,#7987,#4696,.T.);
#10051=EDGE_CURVE('',#7986,#7984,#728,.T.);
#10052=EDGE_CURVE('',#7987,#7985,#729,.T.);
#10053=EDGE_CURVE('',#7988,#7989,#4697,.T.);
#10054=EDGE_CURVE('',#7988,#7986,#730,.T.);
#10055=EDGE_CURVE('',#7989,#7987,#731,.T.);
#10056=EDGE_CURVE('',#7990,#7991,#4698,.T.);
#10057=EDGE_CURVE('',#7990,#7988,#732,.T.);
#10058=EDGE_CURVE('',#7991,#7989,#733,.T.);
#10059=EDGE_CURVE('',#7992,#7993,#4699,.T.);
#10060=EDGE_CURVE('',#7992,#7990,#734,.T.);
#10061=EDGE_CURVE('',#7993,#7991,#735,.T.);
#10062=EDGE_CURVE('',#7994,#7995,#4700,.T.);
#10063=EDGE_CURVE('',#7994,#7992,#736,.T.);
#10064=EDGE_CURVE('',#7995,#7993,#737,.T.);
#10065=EDGE_CURVE('',#7996,#7973,#738,.T.);
#10066=EDGE_CURVE('',#7969,#7996,#739,.T.);
#10067=EDGE_CURVE('',#7997,#7945,#740,.T.);
#10068=EDGE_CURVE('',#7997,#7995,#741,.T.);
#10069=EDGE_CURVE('',#7945,#7998,#6802,.T.);
#10070=EDGE_CURVE('',#7998,#7944,#6803,.T.);
#10071=EDGE_CURVE('',#7944,#7999,#742,.T.);
#10072=EDGE_CURVE('',#7999,#7997,#6804,.T.);
#10073=EDGE_CURVE('',#7999,#7994,#743,.T.);
#10074=EDGE_CURVE('',#7972,#8000,#744,.T.);
#10075=EDGE_CURVE('',#8000,#7968,#745,.T.);
#10076=EDGE_CURVE('',#8000,#7996,#6805,.F.);
#10077=EDGE_CURVE('',#8001,#8001,#6806,.T.);
#10078=EDGE_CURVE('',#8002,#8003,#746,.T.);
#10079=EDGE_CURVE('',#8002,#8004,#4701,.T.);
#10080=EDGE_CURVE('',#8004,#8005,#747,.T.);
#10081=EDGE_CURVE('',#8003,#8005,#4702,.T.);
#10082=EDGE_CURVE('',#8006,#8002,#748,.T.);
#10083=EDGE_CURVE('',#8006,#8007,#4703,.T.);
#10084=EDGE_CURVE('',#8007,#8004,#749,.T.);
#10085=EDGE_CURVE('',#8008,#8006,#750,.T.);
#10086=EDGE_CURVE('',#8008,#8009,#4704,.T.);
#10087=EDGE_CURVE('',#8009,#8007,#751,.T.);
#10088=EDGE_CURVE('',#8010,#8008,#752,.T.);
#10089=EDGE_CURVE('',#8010,#8011,#4705,.T.);
#10090=EDGE_CURVE('',#8011,#8009,#753,.T.);
#10091=EDGE_CURVE('',#8012,#8010,#754,.T.);
#10092=EDGE_CURVE('',#8012,#8013,#4706,.T.);
#10093=EDGE_CURVE('',#8013,#8011,#755,.T.);
#10094=EDGE_CURVE('',#8014,#8012,#756,.T.);
#10095=EDGE_CURVE('',#8014,#8015,#4707,.T.);
#10096=EDGE_CURVE('',#8015,#8013,#757,.T.);
#10097=EDGE_CURVE('',#8016,#8014,#758,.T.);
#10098=EDGE_CURVE('',#8016,#8017,#4708,.T.);
#10099=EDGE_CURVE('',#8017,#8015,#759,.T.);
#10100=EDGE_CURVE('',#8018,#8016,#760,.T.);
#10101=EDGE_CURVE('',#8018,#8019,#4709,.T.);
#10102=EDGE_CURVE('',#8019,#8017,#761,.T.);
#10103=EDGE_CURVE('',#8020,#8018,#762,.T.);
#10104=EDGE_CURVE('',#8020,#8021,#4710,.T.);
#10105=EDGE_CURVE('',#8021,#8019,#763,.T.);
#10106=EDGE_CURVE('',#8022,#8020,#764,.T.);
#10107=EDGE_CURVE('',#8022,#8023,#4711,.T.);
#10108=EDGE_CURVE('',#8023,#8021,#765,.T.);
#10109=EDGE_CURVE('',#8003,#8022,#766,.T.);
#10110=EDGE_CURVE('',#8005,#8023,#767,.T.);
#10111=EDGE_CURVE('',#8024,#8025,#4712,.T.);
#10112=EDGE_CURVE('',#8024,#8026,#4713,.T.);
#10113=EDGE_CURVE('',#8026,#8027,#4714,.T.);
#10114=EDGE_CURVE('',#8025,#8027,#4715,.T.);
#10115=EDGE_CURVE('',#8028,#8024,#4716,.T.);
#10116=EDGE_CURVE('',#8028,#8029,#4717,.T.);
#10117=EDGE_CURVE('',#8029,#8026,#4718,.T.);
#10118=EDGE_CURVE('',#8030,#8028,#4719,.T.);
#10119=EDGE_CURVE('',#8030,#8031,#4720,.T.);
#10120=EDGE_CURVE('',#8031,#8029,#4721,.T.);
#10121=EDGE_CURVE('',#8032,#8030,#4722,.T.);
#10122=EDGE_CURVE('',#8032,#8033,#4723,.T.);
#10123=EDGE_CURVE('',#8033,#8031,#4724,.T.);
#10124=EDGE_CURVE('',#8034,#8032,#4725,.T.);
#10125=EDGE_CURVE('',#8034,#8035,#4726,.T.);
#10126=EDGE_CURVE('',#8035,#8033,#4727,.T.);
#10127=EDGE_CURVE('',#8036,#8034,#4728,.T.);
#10128=EDGE_CURVE('',#8036,#8037,#4729,.T.);
#10129=EDGE_CURVE('',#8037,#8035,#4730,.T.);
#10130=EDGE_CURVE('',#8038,#8036,#4731,.T.);
#10131=EDGE_CURVE('',#8038,#8039,#4732,.T.);
#10132=EDGE_CURVE('',#8039,#8037,#4733,.T.);
#10133=EDGE_CURVE('',#8040,#8038,#4734,.T.);
#10134=EDGE_CURVE('',#8040,#8041,#4735,.T.);
#10135=EDGE_CURVE('',#8041,#8039,#4736,.T.);
#10136=EDGE_CURVE('',#8042,#8040,#4737,.T.);
#10137=EDGE_CURVE('',#8042,#8043,#4738,.T.);
#10138=EDGE_CURVE('',#8043,#8041,#4739,.T.);
#10139=EDGE_CURVE('',#8025,#8042,#4740,.T.);
#10140=EDGE_CURVE('',#8027,#8043,#4741,.T.);
#10141=EDGE_CURVE('',#8044,#8045,#768,.T.);
#10142=EDGE_CURVE('',#8044,#8046,#4742,.T.);
#10143=EDGE_CURVE('',#8046,#8047,#769,.T.);
#10144=EDGE_CURVE('',#8045,#8047,#4743,.T.);
#10145=EDGE_CURVE('',#8048,#8044,#770,.T.);
#10146=EDGE_CURVE('',#8048,#8049,#4744,.T.);
#10147=EDGE_CURVE('',#8049,#8046,#771,.T.);
#10148=EDGE_CURVE('',#8050,#8048,#772,.T.);
#10149=EDGE_CURVE('',#8050,#8051,#4745,.T.);
#10150=EDGE_CURVE('',#8051,#8049,#773,.T.);
#10151=EDGE_CURVE('',#8052,#8050,#774,.T.);
#10152=EDGE_CURVE('',#8052,#8053,#4746,.T.);
#10153=EDGE_CURVE('',#8053,#8051,#775,.T.);
#10154=EDGE_CURVE('',#8054,#8052,#776,.T.);
#10155=EDGE_CURVE('',#8054,#8055,#4747,.T.);
#10156=EDGE_CURVE('',#8055,#8053,#777,.T.);
#10157=EDGE_CURVE('',#8056,#8054,#778,.T.);
#10158=EDGE_CURVE('',#8056,#8057,#4748,.T.);
#10159=EDGE_CURVE('',#8057,#8055,#779,.T.);
#10160=EDGE_CURVE('',#8058,#8056,#780,.T.);
#10161=EDGE_CURVE('',#8058,#8059,#4749,.T.);
#10162=EDGE_CURVE('',#8059,#8057,#781,.T.);
#10163=EDGE_CURVE('',#8060,#8058,#782,.T.);
#10164=EDGE_CURVE('',#8060,#8061,#4750,.T.);
#10165=EDGE_CURVE('',#8061,#8059,#783,.T.);
#10166=EDGE_CURVE('',#8062,#8060,#784,.T.);
#10167=EDGE_CURVE('',#8062,#8063,#4751,.T.);
#10168=EDGE_CURVE('',#8063,#8061,#785,.T.);
#10169=EDGE_CURVE('',#8064,#8062,#786,.T.);
#10170=EDGE_CURVE('',#8064,#8065,#4752,.T.);
#10171=EDGE_CURVE('',#8065,#8063,#787,.T.);
#10172=EDGE_CURVE('',#8045,#8064,#788,.T.);
#10173=EDGE_CURVE('',#8047,#8065,#789,.T.);
#10174=EDGE_CURVE('',#8066,#8067,#4753,.T.);
#10175=EDGE_CURVE('',#8066,#8068,#4754,.T.);
#10176=EDGE_CURVE('',#8068,#8069,#4755,.T.);
#10177=EDGE_CURVE('',#8067,#8069,#4756,.T.);
#10178=EDGE_CURVE('',#8070,#8066,#4757,.T.);
#10179=EDGE_CURVE('',#8070,#8071,#4758,.T.);
#10180=EDGE_CURVE('',#8071,#8068,#4759,.T.);
#10181=EDGE_CURVE('',#8072,#8070,#4760,.T.);
#10182=EDGE_CURVE('',#8072,#8073,#4761,.T.);
#10183=EDGE_CURVE('',#8073,#8071,#4762,.T.);
#10184=EDGE_CURVE('',#8074,#8072,#4763,.T.);
#10185=EDGE_CURVE('',#8074,#8075,#4764,.T.);
#10186=EDGE_CURVE('',#8075,#8073,#4765,.T.);
#10187=EDGE_CURVE('',#8076,#8074,#4766,.T.);
#10188=EDGE_CURVE('',#8076,#8077,#4767,.T.);
#10189=EDGE_CURVE('',#8077,#8075,#4768,.T.);
#10190=EDGE_CURVE('',#8078,#8076,#4769,.T.);
#10191=EDGE_CURVE('',#8078,#8079,#4770,.T.);
#10192=EDGE_CURVE('',#8079,#8077,#4771,.T.);
#10193=EDGE_CURVE('',#8080,#8078,#4772,.T.);
#10194=EDGE_CURVE('',#8080,#8081,#4773,.T.);
#10195=EDGE_CURVE('',#8081,#8079,#4774,.T.);
#10196=EDGE_CURVE('',#8082,#8080,#4775,.T.);
#10197=EDGE_CURVE('',#8082,#8083,#4776,.T.);
#10198=EDGE_CURVE('',#8083,#8081,#4777,.T.);
#10199=EDGE_CURVE('',#8084,#8082,#4778,.T.);
#10200=EDGE_CURVE('',#8084,#8085,#4779,.T.);
#10201=EDGE_CURVE('',#8085,#8083,#4780,.T.);
#10202=EDGE_CURVE('',#8067,#8084,#4781,.T.);
#10203=EDGE_CURVE('',#8069,#8085,#4782,.T.);
#10204=EDGE_CURVE('',#8086,#8087,#4783,.T.);
#10205=EDGE_CURVE('',#8086,#8088,#4784,.T.);
#10206=EDGE_CURVE('',#8088,#8089,#4785,.T.);
#10207=EDGE_CURVE('',#8087,#8089,#4786,.T.);
#10208=EDGE_CURVE('',#8090,#8086,#4787,.T.);
#10209=EDGE_CURVE('',#8090,#8091,#4788,.T.);
#10210=EDGE_CURVE('',#8091,#8088,#4789,.T.);
#10211=EDGE_CURVE('',#8092,#8090,#4790,.T.);
#10212=EDGE_CURVE('',#8092,#8093,#4791,.T.);
#10213=EDGE_CURVE('',#8093,#8091,#4792,.T.);
#10214=EDGE_CURVE('',#8094,#8092,#4793,.T.);
#10215=EDGE_CURVE('',#8094,#8095,#4794,.T.);
#10216=EDGE_CURVE('',#8095,#8093,#4795,.T.);
#10217=EDGE_CURVE('',#8096,#8094,#4796,.T.);
#10218=EDGE_CURVE('',#8096,#8097,#4797,.T.);
#10219=EDGE_CURVE('',#8097,#8095,#4798,.T.);
#10220=EDGE_CURVE('',#8098,#8096,#4799,.T.);
#10221=EDGE_CURVE('',#8098,#8099,#4800,.T.);
#10222=EDGE_CURVE('',#8099,#8097,#4801,.T.);
#10223=EDGE_CURVE('',#8100,#8098,#4802,.T.);
#10224=EDGE_CURVE('',#8100,#8101,#4803,.T.);
#10225=EDGE_CURVE('',#8101,#8099,#4804,.T.);
#10226=EDGE_CURVE('',#8102,#8100,#4805,.T.);
#10227=EDGE_CURVE('',#8102,#8103,#4806,.T.);
#10228=EDGE_CURVE('',#8103,#8101,#4807,.T.);
#10229=EDGE_CURVE('',#8104,#8102,#4808,.T.);
#10230=EDGE_CURVE('',#8104,#8105,#4809,.T.);
#10231=EDGE_CURVE('',#8105,#8103,#4810,.T.);
#10232=EDGE_CURVE('',#8087,#8104,#4811,.T.);
#10233=EDGE_CURVE('',#8089,#8105,#4812,.T.);
#10234=EDGE_CURVE('',#8106,#8106,#6807,.T.);
#10235=EDGE_CURVE('',#8107,#8107,#6808,.T.);
#10236=EDGE_CURVE('',#8106,#8108,#4813,.T.);
#10237=EDGE_CURVE('',#8108,#8108,#6809,.T.);
#10238=EDGE_CURVE('',#8107,#8109,#4814,.T.);
#10239=EDGE_CURVE('',#8109,#8109,#6810,.T.);
#10240=EDGE_CURVE('',#8110,#8111,#4815,.T.);
#10241=EDGE_CURVE('',#8110,#8112,#4816,.T.);
#10242=EDGE_CURVE('',#8113,#8112,#4817,.T.);
#10243=EDGE_CURVE('',#8111,#8113,#4818,.T.);
#10244=EDGE_CURVE('',#8111,#8114,#6811,.T.);
#10245=EDGE_CURVE('',#8113,#8114,#4819,.T.);
#10246=EDGE_CURVE('',#8114,#8115,#4820,.T.);
#10247=EDGE_CURVE('',#8112,#8115,#4821,.T.);
#10248=EDGE_CURVE('',#8115,#8110,#6812,.T.);
#10249=EDGE_CURVE('',#8116,#8117,#4822,.T.);
#10250=EDGE_CURVE('',#8116,#8118,#4823,.T.);
#10251=EDGE_CURVE('',#8119,#8118,#4824,.T.);
#10252=EDGE_CURVE('',#8117,#8119,#4825,.T.);
#10253=EDGE_CURVE('',#8117,#8120,#6813,.T.);
#10254=EDGE_CURVE('',#8119,#8120,#4826,.T.);
#10255=EDGE_CURVE('',#8120,#8121,#4827,.T.);
#10256=EDGE_CURVE('',#8118,#8121,#4828,.T.);
#10257=EDGE_CURVE('',#8121,#8116,#6814,.T.);
#10258=EDGE_CURVE('',#8122,#8123,#4829,.T.);
#10259=EDGE_CURVE('',#8122,#8124,#4830,.T.);
#10260=EDGE_CURVE('',#8125,#8124,#4831,.T.);
#10261=EDGE_CURVE('',#8123,#8125,#4832,.T.);
#10262=EDGE_CURVE('',#8123,#8126,#6815,.T.);
#10263=EDGE_CURVE('',#8125,#8126,#4833,.T.);
#10264=EDGE_CURVE('',#8126,#8127,#4834,.T.);
#10265=EDGE_CURVE('',#8124,#8127,#4835,.T.);
#10266=EDGE_CURVE('',#8127,#8122,#6816,.T.);
#10267=EDGE_CURVE('',#8128,#8129,#4836,.T.);
#10268=EDGE_CURVE('',#8128,#8130,#4837,.T.);
#10269=EDGE_CURVE('',#8131,#8130,#4838,.T.);
#10270=EDGE_CURVE('',#8129,#8131,#4839,.T.);
#10271=EDGE_CURVE('',#8129,#8132,#6817,.T.);
#10272=EDGE_CURVE('',#8131,#8132,#4840,.T.);
#10273=EDGE_CURVE('',#8132,#8133,#4841,.T.);
#10274=EDGE_CURVE('',#8130,#8133,#4842,.T.);
#10275=EDGE_CURVE('',#8133,#8128,#6818,.T.);
#10276=EDGE_CURVE('',#8134,#8135,#4843,.T.);
#10277=EDGE_CURVE('',#8134,#8136,#4844,.T.);
#10278=EDGE_CURVE('',#8137,#8136,#4845,.T.);
#10279=EDGE_CURVE('',#8135,#8137,#4846,.T.);
#10280=EDGE_CURVE('',#8135,#8138,#6819,.T.);
#10281=EDGE_CURVE('',#8137,#8138,#4847,.T.);
#10282=EDGE_CURVE('',#8138,#8139,#4848,.T.);
#10283=EDGE_CURVE('',#8136,#8139,#4849,.T.);
#10284=EDGE_CURVE('',#8139,#8134,#6820,.T.);
#10285=EDGE_CURVE('',#8140,#8141,#4850,.T.);
#10286=EDGE_CURVE('',#8140,#8142,#4851,.T.);
#10287=EDGE_CURVE('',#8143,#8142,#4852,.T.);
#10288=EDGE_CURVE('',#8141,#8143,#4853,.T.);
#10289=EDGE_CURVE('',#8141,#8144,#6821,.T.);
#10290=EDGE_CURVE('',#8143,#8144,#4854,.T.);
#10291=EDGE_CURVE('',#8144,#8145,#4855,.T.);
#10292=EDGE_CURVE('',#8142,#8145,#4856,.T.);
#10293=EDGE_CURVE('',#8145,#8140,#6822,.T.);
#10294=EDGE_CURVE('',#8146,#8147,#4857,.T.);
#10295=EDGE_CURVE('',#8146,#8148,#4858,.T.);
#10296=EDGE_CURVE('',#8149,#8148,#4859,.T.);
#10297=EDGE_CURVE('',#8147,#8149,#4860,.T.);
#10298=EDGE_CURVE('',#8147,#8150,#6823,.T.);
#10299=EDGE_CURVE('',#8149,#8150,#4861,.T.);
#10300=EDGE_CURVE('',#8150,#8151,#4862,.T.);
#10301=EDGE_CURVE('',#8148,#8151,#4863,.T.);
#10302=EDGE_CURVE('',#8151,#8146,#6824,.T.);
#10303=EDGE_CURVE('',#8152,#8153,#4864,.T.);
#10304=EDGE_CURVE('',#8152,#8154,#4865,.T.);
#10305=EDGE_CURVE('',#8155,#8154,#4866,.T.);
#10306=EDGE_CURVE('',#8153,#8155,#4867,.T.);
#10307=EDGE_CURVE('',#8153,#8156,#6825,.T.);
#10308=EDGE_CURVE('',#8155,#8156,#4868,.T.);
#10309=EDGE_CURVE('',#8156,#8157,#4869,.T.);
#10310=EDGE_CURVE('',#8154,#8157,#4870,.T.);
#10311=EDGE_CURVE('',#8157,#8152,#6826,.T.);
#10312=EDGE_CURVE('',#8158,#8159,#4871,.T.);
#10313=EDGE_CURVE('',#8158,#8160,#4872,.T.);
#10314=EDGE_CURVE('',#8161,#8160,#4873,.T.);
#10315=EDGE_CURVE('',#8159,#8161,#4874,.T.);
#10316=EDGE_CURVE('',#8159,#8162,#6827,.T.);
#10317=EDGE_CURVE('',#8161,#8162,#4875,.T.);
#10318=EDGE_CURVE('',#8162,#8163,#4876,.T.);
#10319=EDGE_CURVE('',#8160,#8163,#4877,.T.);
#10320=EDGE_CURVE('',#8163,#8158,#6828,.T.);
#10321=EDGE_CURVE('',#8164,#8165,#4878,.T.);
#10322=EDGE_CURVE('',#8164,#8166,#4879,.T.);
#10323=EDGE_CURVE('',#8167,#8166,#4880,.T.);
#10324=EDGE_CURVE('',#8165,#8167,#4881,.T.);
#10325=EDGE_CURVE('',#8165,#8168,#6829,.T.);
#10326=EDGE_CURVE('',#8167,#8168,#4882,.T.);
#10327=EDGE_CURVE('',#8168,#8169,#4883,.T.);
#10328=EDGE_CURVE('',#8166,#8169,#4884,.T.);
#10329=EDGE_CURVE('',#8169,#8164,#6830,.T.);
#10330=EDGE_CURVE('',#8170,#8171,#4885,.T.);
#10331=EDGE_CURVE('',#8170,#8172,#4886,.T.);
#10332=EDGE_CURVE('',#8173,#8172,#4887,.T.);
#10333=EDGE_CURVE('',#8171,#8173,#4888,.T.);
#10334=EDGE_CURVE('',#8171,#8174,#6831,.T.);
#10335=EDGE_CURVE('',#8173,#8174,#4889,.T.);
#10336=EDGE_CURVE('',#8174,#8175,#4890,.T.);
#10337=EDGE_CURVE('',#8172,#8175,#4891,.T.);
#10338=EDGE_CURVE('',#8175,#8170,#6832,.T.);
#10339=EDGE_CURVE('',#8176,#8177,#4892,.T.);
#10340=EDGE_CURVE('',#8176,#8178,#4893,.T.);
#10341=EDGE_CURVE('',#8179,#8178,#4894,.T.);
#10342=EDGE_CURVE('',#8177,#8179,#4895,.T.);
#10343=EDGE_CURVE('',#8177,#8180,#6833,.T.);
#10344=EDGE_CURVE('',#8179,#8180,#4896,.T.);
#10345=EDGE_CURVE('',#8180,#8181,#4897,.T.);
#10346=EDGE_CURVE('',#8178,#8181,#4898,.T.);
#10347=EDGE_CURVE('',#8181,#8176,#6834,.T.);
#10348=EDGE_CURVE('',#8182,#8183,#4899,.T.);
#10349=EDGE_CURVE('',#8182,#8184,#4900,.T.);
#10350=EDGE_CURVE('',#8185,#8184,#4901,.T.);
#10351=EDGE_CURVE('',#8183,#8185,#4902,.T.);
#10352=EDGE_CURVE('',#8183,#8186,#6835,.T.);
#10353=EDGE_CURVE('',#8185,#8186,#4903,.T.);
#10354=EDGE_CURVE('',#8186,#8187,#4904,.T.);
#10355=EDGE_CURVE('',#8184,#8187,#4905,.T.);
#10356=EDGE_CURVE('',#8187,#8182,#6836,.T.);
#10357=EDGE_CURVE('',#8188,#8189,#4906,.T.);
#10358=EDGE_CURVE('',#8188,#8190,#4907,.T.);
#10359=EDGE_CURVE('',#8191,#8190,#4908,.T.);
#10360=EDGE_CURVE('',#8189,#8191,#4909,.T.);
#10361=EDGE_CURVE('',#8189,#8192,#6837,.T.);
#10362=EDGE_CURVE('',#8191,#8192,#4910,.T.);
#10363=EDGE_CURVE('',#8192,#8193,#4911,.T.);
#10364=EDGE_CURVE('',#8190,#8193,#4912,.T.);
#10365=EDGE_CURVE('',#8193,#8188,#6838,.T.);
#10366=EDGE_CURVE('',#8194,#8195,#4913,.T.);
#10367=EDGE_CURVE('',#8194,#8196,#4914,.T.);
#10368=EDGE_CURVE('',#8197,#8196,#4915,.T.);
#10369=EDGE_CURVE('',#8195,#8197,#4916,.T.);
#10370=EDGE_CURVE('',#8195,#8198,#6839,.T.);
#10371=EDGE_CURVE('',#8197,#8199,#4917,.T.);
#10372=EDGE_CURVE('',#8198,#8199,#6840,.T.);
#10373=EDGE_CURVE('',#8199,#8200,#4918,.T.);
#10374=EDGE_CURVE('',#8196,#8200,#4919,.T.);
#10375=EDGE_CURVE('',#8200,#8201,#6841,.T.);
#10376=EDGE_CURVE('',#8201,#8194,#6842,.T.);
#10377=EDGE_CURVE('',#8202,#8203,#4920,.T.);
#10378=EDGE_CURVE('',#8202,#8204,#4921,.T.);
#10379=EDGE_CURVE('',#8205,#8204,#4922,.T.);
#10380=EDGE_CURVE('',#8203,#8205,#4923,.T.);
#10381=EDGE_CURVE('',#8203,#8206,#6843,.T.);
#10382=EDGE_CURVE('',#8205,#8206,#4924,.T.);
#10383=EDGE_CURVE('',#8206,#8207,#4925,.T.);
#10384=EDGE_CURVE('',#8204,#8207,#4926,.T.);
#10385=EDGE_CURVE('',#8207,#8202,#6844,.T.);
#10386=EDGE_CURVE('',#8208,#8209,#4927,.T.);
#10387=EDGE_CURVE('',#8208,#8210,#4928,.T.);
#10388=EDGE_CURVE('',#8211,#8210,#4929,.T.);
#10389=EDGE_CURVE('',#8209,#8211,#4930,.T.);
#10390=EDGE_CURVE('',#8209,#8212,#6845,.T.);
#10391=EDGE_CURVE('',#8211,#8212,#4931,.T.);
#10392=EDGE_CURVE('',#8212,#8213,#4932,.T.);
#10393=EDGE_CURVE('',#8210,#8213,#4933,.T.);
#10394=EDGE_CURVE('',#8213,#8208,#6846,.T.);
#10395=EDGE_CURVE('',#8214,#8215,#4934,.T.);
#10396=EDGE_CURVE('',#8214,#8216,#4935,.T.);
#10397=EDGE_CURVE('',#8217,#8216,#4936,.T.);
#10398=EDGE_CURVE('',#8215,#8217,#4937,.T.);
#10399=EDGE_CURVE('',#8215,#8218,#6847,.T.);
#10400=EDGE_CURVE('',#8217,#8218,#4938,.T.);
#10401=EDGE_CURVE('',#8218,#8219,#4939,.T.);
#10402=EDGE_CURVE('',#8216,#8219,#4940,.T.);
#10403=EDGE_CURVE('',#8219,#8214,#6848,.T.);
#10404=EDGE_CURVE('',#8220,#8221,#4941,.T.);
#10405=EDGE_CURVE('',#8220,#8222,#4942,.T.);
#10406=EDGE_CURVE('',#8223,#8222,#4943,.T.);
#10407=EDGE_CURVE('',#8221,#8223,#4944,.T.);
#10408=EDGE_CURVE('',#8221,#8224,#6849,.T.);
#10409=EDGE_CURVE('',#8223,#8224,#4945,.T.);
#10410=EDGE_CURVE('',#8224,#8225,#4946,.T.);
#10411=EDGE_CURVE('',#8222,#8225,#4947,.T.);
#10412=EDGE_CURVE('',#8225,#8220,#6850,.T.);
#10413=EDGE_CURVE('',#8226,#8227,#4948,.T.);
#10414=EDGE_CURVE('',#8226,#8228,#4949,.T.);
#10415=EDGE_CURVE('',#8229,#8228,#4950,.T.);
#10416=EDGE_CURVE('',#8227,#8229,#4951,.T.);
#10417=EDGE_CURVE('',#8227,#8230,#6851,.T.);
#10418=EDGE_CURVE('',#8229,#8230,#4952,.T.);
#10419=EDGE_CURVE('',#8230,#8231,#4953,.T.);
#10420=EDGE_CURVE('',#8228,#8231,#4954,.T.);
#10421=EDGE_CURVE('',#8231,#8226,#6852,.T.);
#10422=EDGE_CURVE('',#8232,#8233,#4955,.T.);
#10423=EDGE_CURVE('',#8232,#8234,#4956,.T.);
#10424=EDGE_CURVE('',#8235,#8234,#4957,.T.);
#10425=EDGE_CURVE('',#8233,#8235,#4958,.T.);
#10426=EDGE_CURVE('',#8233,#8236,#6853,.T.);
#10427=EDGE_CURVE('',#8235,#8236,#4959,.T.);
#10428=EDGE_CURVE('',#8236,#8237,#4960,.T.);
#10429=EDGE_CURVE('',#8234,#8237,#4961,.T.);
#10430=EDGE_CURVE('',#8237,#8232,#6854,.T.);
#10431=EDGE_CURVE('',#8238,#8239,#4962,.T.);
#10432=EDGE_CURVE('',#8238,#8240,#4963,.T.);
#10433=EDGE_CURVE('',#8241,#8240,#4964,.T.);
#10434=EDGE_CURVE('',#8239,#8241,#4965,.T.);
#10435=EDGE_CURVE('',#8239,#8242,#6855,.T.);
#10436=EDGE_CURVE('',#8241,#8242,#4966,.T.);
#10437=EDGE_CURVE('',#8242,#8243,#4967,.T.);
#10438=EDGE_CURVE('',#8240,#8243,#4968,.T.);
#10439=EDGE_CURVE('',#8243,#8238,#6856,.T.);
#10440=EDGE_CURVE('',#8244,#8245,#4969,.T.);
#10441=EDGE_CURVE('',#8244,#8246,#4970,.T.);
#10442=EDGE_CURVE('',#8247,#8246,#4971,.T.);
#10443=EDGE_CURVE('',#8245,#8247,#4972,.T.);
#10444=EDGE_CURVE('',#8245,#8248,#6857,.T.);
#10445=EDGE_CURVE('',#8247,#8248,#4973,.T.);
#10446=EDGE_CURVE('',#8248,#8249,#4974,.T.);
#10447=EDGE_CURVE('',#8246,#8249,#4975,.T.);
#10448=EDGE_CURVE('',#8249,#8244,#6858,.T.);
#10449=EDGE_CURVE('',#8250,#8251,#4976,.T.);
#10450=EDGE_CURVE('',#8250,#8252,#4977,.T.);
#10451=EDGE_CURVE('',#8253,#8252,#4978,.T.);
#10452=EDGE_CURVE('',#8251,#8253,#4979,.T.);
#10453=EDGE_CURVE('',#8251,#8254,#6859,.T.);
#10454=EDGE_CURVE('',#8253,#8254,#4980,.T.);
#10455=EDGE_CURVE('',#8254,#8255,#4981,.T.);
#10456=EDGE_CURVE('',#8252,#8255,#4982,.T.);
#10457=EDGE_CURVE('',#8255,#8250,#6860,.T.);
#10458=EDGE_CURVE('',#8256,#8257,#4983,.T.);
#10459=EDGE_CURVE('',#8256,#8258,#4984,.T.);
#10460=EDGE_CURVE('',#8259,#8258,#4985,.T.);
#10461=EDGE_CURVE('',#8257,#8259,#4986,.T.);
#10462=EDGE_CURVE('',#8257,#8260,#6861,.T.);
#10463=EDGE_CURVE('',#8259,#8260,#4987,.T.);
#10464=EDGE_CURVE('',#8260,#8261,#4988,.T.);
#10465=EDGE_CURVE('',#8258,#8261,#4989,.T.);
#10466=EDGE_CURVE('',#8261,#8256,#6862,.T.);
#10467=EDGE_CURVE('',#8262,#8263,#4990,.T.);
#10468=EDGE_CURVE('',#8262,#8264,#4991,.T.);
#10469=EDGE_CURVE('',#8265,#8264,#4992,.T.);
#10470=EDGE_CURVE('',#8263,#8265,#4993,.T.);
#10471=EDGE_CURVE('',#8263,#8266,#6863,.T.);
#10472=EDGE_CURVE('',#8265,#8266,#4994,.T.);
#10473=EDGE_CURVE('',#8266,#8267,#4995,.T.);
#10474=EDGE_CURVE('',#8264,#8267,#4996,.T.);
#10475=EDGE_CURVE('',#8267,#8262,#6864,.T.);
#10476=EDGE_CURVE('',#8268,#8269,#4997,.T.);
#10477=EDGE_CURVE('',#8268,#8270,#4998,.T.);
#10478=EDGE_CURVE('',#8271,#8270,#4999,.T.);
#10479=EDGE_CURVE('',#8269,#8271,#5000,.T.);
#10480=EDGE_CURVE('',#8269,#8272,#6865,.T.);
#10481=EDGE_CURVE('',#8271,#8272,#5001,.T.);
#10482=EDGE_CURVE('',#8272,#8273,#5002,.T.);
#10483=EDGE_CURVE('',#8270,#8273,#5003,.T.);
#10484=EDGE_CURVE('',#8273,#8268,#6866,.T.);
#10485=EDGE_CURVE('',#8274,#8275,#5004,.T.);
#10486=EDGE_CURVE('',#8274,#8276,#5005,.T.);
#10487=EDGE_CURVE('',#8277,#8276,#5006,.T.);
#10488=EDGE_CURVE('',#8275,#8277,#5007,.T.);
#10489=EDGE_CURVE('',#8275,#8278,#6867,.T.);
#10490=EDGE_CURVE('',#8277,#8278,#5008,.T.);
#10491=EDGE_CURVE('',#8278,#8279,#5009,.T.);
#10492=EDGE_CURVE('',#8276,#8279,#5010,.T.);
#10493=EDGE_CURVE('',#8279,#8274,#6868,.T.);
#10494=EDGE_CURVE('',#8280,#8281,#5011,.T.);
#10495=EDGE_CURVE('',#8280,#8282,#5012,.T.);
#10496=EDGE_CURVE('',#8283,#8282,#5013,.T.);
#10497=EDGE_CURVE('',#8281,#8283,#5014,.T.);
#10498=EDGE_CURVE('',#8281,#8284,#6869,.T.);
#10499=EDGE_CURVE('',#8283,#8284,#5015,.T.);
#10500=EDGE_CURVE('',#8284,#8285,#5016,.T.);
#10501=EDGE_CURVE('',#8282,#8285,#5017,.T.);
#10502=EDGE_CURVE('',#8285,#8280,#6870,.T.);
#10503=EDGE_CURVE('',#8286,#8287,#5018,.T.);
#10504=EDGE_CURVE('',#8286,#8288,#5019,.T.);
#10505=EDGE_CURVE('',#8289,#8288,#5020,.T.);
#10506=EDGE_CURVE('',#8287,#8289,#5021,.T.);
#10507=EDGE_CURVE('',#8287,#8290,#6871,.T.);
#10508=EDGE_CURVE('',#8289,#8290,#5022,.T.);
#10509=EDGE_CURVE('',#8290,#8291,#5023,.T.);
#10510=EDGE_CURVE('',#8288,#8291,#5024,.T.);
#10511=EDGE_CURVE('',#8291,#8286,#6872,.T.);
#10512=EDGE_CURVE('',#8292,#8292,#6873,.T.);
#10513=EDGE_CURVE('',#8293,#8293,#6874,.T.);
#10514=EDGE_CURVE('',#8293,#8292,#5025,.T.);
#10515=EDGE_CURVE('',#7998,#8293,#5026,.T.);
#10516=EDGE_CURVE('',#8294,#8294,#6875,.T.);
#10517=EDGE_CURVE('',#8294,#8001,#5027,.T.);
#10518=EDGE_CURVE('',#8295,#8295,#6876,.T.);
#10519=EDGE_CURVE('',#8296,#8296,#6877,.T.);
#10520=EDGE_CURVE('',#8296,#8295,#5028,.T.);
#10521=EDGE_CURVE('',#8297,#8297,#6878,.T.);
#10522=EDGE_CURVE('',#8297,#8201,#5029,.T.);
#10523=EDGE_CURVE('',#8198,#8296,#5030,.T.);
#10524=EDGE_CURVE('',#8298,#8298,#6879,.T.);
#10525=EDGE_CURVE('',#8298,#8297,#5031,.T.);
#13850=ORIENTED_EDGE('',*,*,#9988,.F.);
#13851=ORIENTED_EDGE('',*,*,#9989,.T.);
#13852=ORIENTED_EDGE('',*,*,#9990,.T.);
#13853=ORIENTED_EDGE('',*,*,#9991,.T.);
#13854=ORIENTED_EDGE('',*,*,#9992,.F.);
#13855=ORIENTED_EDGE('',*,*,#9993,.T.);
#13856=ORIENTED_EDGE('',*,*,#9988,.T.);
#13857=ORIENTED_EDGE('',*,*,#9994,.T.);
#13858=ORIENTED_EDGE('',*,*,#9995,.F.);
#13859=ORIENTED_EDGE('',*,*,#9996,.T.);
#13860=ORIENTED_EDGE('',*,*,#9992,.T.);
#13861=ORIENTED_EDGE('',*,*,#9997,.T.);
#13862=ORIENTED_EDGE('',*,*,#9998,.F.);
#13863=ORIENTED_EDGE('',*,*,#9999,.T.);
#13864=ORIENTED_EDGE('',*,*,#9995,.T.);
#13865=ORIENTED_EDGE('',*,*,#10000,.T.);
#13866=ORIENTED_EDGE('',*,*,#10001,.F.);
#13867=ORIENTED_EDGE('',*,*,#10002,.T.);
#13868=ORIENTED_EDGE('',*,*,#9998,.T.);
#13869=ORIENTED_EDGE('',*,*,#10003,.T.);
#13870=ORIENTED_EDGE('',*,*,#10004,.F.);
#13871=ORIENTED_EDGE('',*,*,#10005,.T.);
#13872=ORIENTED_EDGE('',*,*,#10001,.T.);
#13873=ORIENTED_EDGE('',*,*,#10006,.T.);
#13874=ORIENTED_EDGE('',*,*,#10007,.F.);
#13875=ORIENTED_EDGE('',*,*,#10008,.T.);
#13876=ORIENTED_EDGE('',*,*,#10004,.T.);
#13877=ORIENTED_EDGE('',*,*,#10009,.T.);
#13878=ORIENTED_EDGE('',*,*,#10010,.F.);
#13879=ORIENTED_EDGE('',*,*,#10011,.T.);
#13880=ORIENTED_EDGE('',*,*,#10007,.T.);
#13881=ORIENTED_EDGE('',*,*,#10012,.T.);
#13882=ORIENTED_EDGE('',*,*,#10013,.F.);
#13883=ORIENTED_EDGE('',*,*,#10014,.T.);
#13884=ORIENTED_EDGE('',*,*,#10010,.T.);
#13885=ORIENTED_EDGE('',*,*,#10015,.T.);
#13886=ORIENTED_EDGE('',*,*,#10016,.F.);
#13887=ORIENTED_EDGE('',*,*,#10017,.T.);
#13888=ORIENTED_EDGE('',*,*,#10013,.T.);
#13889=ORIENTED_EDGE('',*,*,#10018,.T.);
#13890=ORIENTED_EDGE('',*,*,#10019,.F.);
#13891=ORIENTED_EDGE('',*,*,#10020,.T.);
#13892=ORIENTED_EDGE('',*,*,#10016,.T.);
#13893=ORIENTED_EDGE('',*,*,#10021,.T.);
#13894=ORIENTED_EDGE('',*,*,#10022,.F.);
#13895=ORIENTED_EDGE('',*,*,#10023,.T.);
#13896=ORIENTED_EDGE('',*,*,#10019,.T.);
#13897=ORIENTED_EDGE('',*,*,#10024,.T.);
#13898=ORIENTED_EDGE('',*,*,#10025,.F.);
#13899=ORIENTED_EDGE('',*,*,#10026,.T.);
#13900=ORIENTED_EDGE('',*,*,#10022,.T.);
#13901=ORIENTED_EDGE('',*,*,#10027,.T.);
#13902=ORIENTED_EDGE('',*,*,#10028,.F.);
#13903=ORIENTED_EDGE('',*,*,#10029,.T.);
#13904=ORIENTED_EDGE('',*,*,#10030,.F.);
#13905=ORIENTED_EDGE('',*,*,#10031,.F.);
#13906=ORIENTED_EDGE('',*,*,#10032,.F.);
#13907=ORIENTED_EDGE('',*,*,#10033,.T.);
#13908=ORIENTED_EDGE('',*,*,#10028,.T.);
#13909=ORIENTED_EDGE('',*,*,#10034,.F.);
#13910=ORIENTED_EDGE('',*,*,#10035,.F.);
#13911=ORIENTED_EDGE('',*,*,#10036,.T.);
#13912=ORIENTED_EDGE('',*,*,#10032,.T.);
#13913=ORIENTED_EDGE('',*,*,#10037,.F.);
#13914=ORIENTED_EDGE('',*,*,#10038,.F.);
#13915=ORIENTED_EDGE('',*,*,#10039,.T.);
#13916=ORIENTED_EDGE('',*,*,#10035,.T.);
#13917=ORIENTED_EDGE('',*,*,#10040,.F.);
#13918=ORIENTED_EDGE('',*,*,#10041,.F.);
#13919=ORIENTED_EDGE('',*,*,#10042,.T.);
#13920=ORIENTED_EDGE('',*,*,#10038,.T.);
#13921=ORIENTED_EDGE('',*,*,#10043,.F.);
#13922=ORIENTED_EDGE('',*,*,#10044,.F.);
#13923=ORIENTED_EDGE('',*,*,#10045,.T.);
#13924=ORIENTED_EDGE('',*,*,#10041,.T.);
#13925=ORIENTED_EDGE('',*,*,#10046,.F.);
#13926=ORIENTED_EDGE('',*,*,#10047,.F.);
#13927=ORIENTED_EDGE('',*,*,#10048,.T.);
#13928=ORIENTED_EDGE('',*,*,#10044,.T.);
#13929=ORIENTED_EDGE('',*,*,#10049,.F.);
#13930=ORIENTED_EDGE('',*,*,#10050,.F.);
#13931=ORIENTED_EDGE('',*,*,#10051,.T.);
#13932=ORIENTED_EDGE('',*,*,#10047,.T.);
#13933=ORIENTED_EDGE('',*,*,#10052,.F.);
#13934=ORIENTED_EDGE('',*,*,#10053,.F.);
#13935=ORIENTED_EDGE('',*,*,#10054,.T.);
#13936=ORIENTED_EDGE('',*,*,#10050,.T.);
#13937=ORIENTED_EDGE('',*,*,#10055,.F.);
#13938=ORIENTED_EDGE('',*,*,#10056,.F.);
#13939=ORIENTED_EDGE('',*,*,#10057,.T.);
#13940=ORIENTED_EDGE('',*,*,#10053,.T.);
#13941=ORIENTED_EDGE('',*,*,#10058,.F.);
#13942=ORIENTED_EDGE('',*,*,#10059,.F.);
#13943=ORIENTED_EDGE('',*,*,#10060,.T.);
#13944=ORIENTED_EDGE('',*,*,#10056,.T.);
#13945=ORIENTED_EDGE('',*,*,#10061,.F.);
#13946=ORIENTED_EDGE('',*,*,#10062,.F.);
#13947=ORIENTED_EDGE('',*,*,#10063,.T.);
#13948=ORIENTED_EDGE('',*,*,#10059,.T.);
#13949=ORIENTED_EDGE('',*,*,#10064,.F.);
#13950=ORIENTED_EDGE('',*,*,#10065,.F.);
#13951=ORIENTED_EDGE('',*,*,#10066,.F.);
#13952=ORIENTED_EDGE('',*,*,#10027,.F.);
#13953=ORIENTED_EDGE('',*,*,#10024,.F.);
#13954=ORIENTED_EDGE('',*,*,#10021,.F.);
#13955=ORIENTED_EDGE('',*,*,#10018,.F.);
#13956=ORIENTED_EDGE('',*,*,#10015,.F.);
#13957=ORIENTED_EDGE('',*,*,#10012,.F.);
#13958=ORIENTED_EDGE('',*,*,#10009,.F.);
#13959=ORIENTED_EDGE('',*,*,#10006,.F.);
#13960=ORIENTED_EDGE('',*,*,#10003,.F.);
#13961=ORIENTED_EDGE('',*,*,#10000,.F.);
#13962=ORIENTED_EDGE('',*,*,#9997,.F.);
#13963=ORIENTED_EDGE('',*,*,#9994,.F.);
#13964=ORIENTED_EDGE('',*,*,#9991,.F.);
#13965=ORIENTED_EDGE('',*,*,#10067,.F.);
#13966=ORIENTED_EDGE('',*,*,#10068,.T.);
#13967=ORIENTED_EDGE('',*,*,#10064,.T.);
#13968=ORIENTED_EDGE('',*,*,#10061,.T.);
#13969=ORIENTED_EDGE('',*,*,#10058,.T.);
#13970=ORIENTED_EDGE('',*,*,#10055,.T.);
#13971=ORIENTED_EDGE('',*,*,#10052,.T.);
#13972=ORIENTED_EDGE('',*,*,#10049,.T.);
#13973=ORIENTED_EDGE('',*,*,#10046,.T.);
#13974=ORIENTED_EDGE('',*,*,#10043,.T.);
#13975=ORIENTED_EDGE('',*,*,#10040,.T.);
#13976=ORIENTED_EDGE('',*,*,#10037,.T.);
#13977=ORIENTED_EDGE('',*,*,#10034,.T.);
#13978=ORIENTED_EDGE('',*,*,#10031,.T.);
#13979=ORIENTED_EDGE('',*,*,#10069,.T.);
#13980=ORIENTED_EDGE('',*,*,#10070,.T.);
#13981=ORIENTED_EDGE('',*,*,#10071,.T.);
#13982=ORIENTED_EDGE('',*,*,#10072,.T.);
#13983=ORIENTED_EDGE('',*,*,#10067,.T.);
#13984=ORIENTED_EDGE('',*,*,#10062,.T.);
#13985=ORIENTED_EDGE('',*,*,#10068,.F.);
#13986=ORIENTED_EDGE('',*,*,#10072,.F.);
#13987=ORIENTED_EDGE('',*,*,#10073,.T.);
#13988=ORIENTED_EDGE('',*,*,#10074,.F.);
#13989=ORIENTED_EDGE('',*,*,#10029,.F.);
#13990=ORIENTED_EDGE('',*,*,#10033,.F.);
#13991=ORIENTED_EDGE('',*,*,#10036,.F.);
#13992=ORIENTED_EDGE('',*,*,#10039,.F.);
#13993=ORIENTED_EDGE('',*,*,#10042,.F.);
#13994=ORIENTED_EDGE('',*,*,#10045,.F.);
#13995=ORIENTED_EDGE('',*,*,#10048,.F.);
#13996=ORIENTED_EDGE('',*,*,#10051,.F.);
#13997=ORIENTED_EDGE('',*,*,#10054,.F.);
#13998=ORIENTED_EDGE('',*,*,#10057,.F.);
#13999=ORIENTED_EDGE('',*,*,#10060,.F.);
#14000=ORIENTED_EDGE('',*,*,#10063,.F.);
#14001=ORIENTED_EDGE('',*,*,#10073,.F.);
#14002=ORIENTED_EDGE('',*,*,#10071,.F.);
#14003=ORIENTED_EDGE('',*,*,#9989,.F.);
#14004=ORIENTED_EDGE('',*,*,#9993,.F.);
#14005=ORIENTED_EDGE('',*,*,#9996,.F.);
#14006=ORIENTED_EDGE('',*,*,#9999,.F.);
#14007=ORIENTED_EDGE('',*,*,#10002,.F.);
#14008=ORIENTED_EDGE('',*,*,#10005,.F.);
#14009=ORIENTED_EDGE('',*,*,#10008,.F.);
#14010=ORIENTED_EDGE('',*,*,#10011,.F.);
#14011=ORIENTED_EDGE('',*,*,#10014,.F.);
#14012=ORIENTED_EDGE('',*,*,#10017,.F.);
#14013=ORIENTED_EDGE('',*,*,#10020,.F.);
#14014=ORIENTED_EDGE('',*,*,#10023,.F.);
#14015=ORIENTED_EDGE('',*,*,#10026,.F.);
#14016=ORIENTED_EDGE('',*,*,#10075,.F.);
#14017=ORIENTED_EDGE('',*,*,#10065,.T.);
#14018=ORIENTED_EDGE('',*,*,#10030,.T.);
#14019=ORIENTED_EDGE('',*,*,#10074,.T.);
#14020=ORIENTED_EDGE('',*,*,#10076,.T.);
#14021=ORIENTED_EDGE('',*,*,#10077,.F.);
#14022=ORIENTED_EDGE('',*,*,#10078,.F.);
#14023=ORIENTED_EDGE('',*,*,#10079,.T.);
#14024=ORIENTED_EDGE('',*,*,#10080,.T.);
#14025=ORIENTED_EDGE('',*,*,#10081,.F.);
#14026=ORIENTED_EDGE('',*,*,#10082,.F.);
#14027=ORIENTED_EDGE('',*,*,#10083,.T.);
#14028=ORIENTED_EDGE('',*,*,#10084,.T.);
#14029=ORIENTED_EDGE('',*,*,#10079,.F.);
#14030=ORIENTED_EDGE('',*,*,#10085,.F.);
#14031=ORIENTED_EDGE('',*,*,#10086,.T.);
#14032=ORIENTED_EDGE('',*,*,#10087,.T.);
#14033=ORIENTED_EDGE('',*,*,#10083,.F.);
#14034=ORIENTED_EDGE('',*,*,#10088,.F.);
#14035=ORIENTED_EDGE('',*,*,#10089,.T.);
#14036=ORIENTED_EDGE('',*,*,#10090,.T.);
#14037=ORIENTED_EDGE('',*,*,#10086,.F.);
#14038=ORIENTED_EDGE('',*,*,#10091,.F.);
#14039=ORIENTED_EDGE('',*,*,#10092,.T.);
#14040=ORIENTED_EDGE('',*,*,#10093,.T.);
#14041=ORIENTED_EDGE('',*,*,#10089,.F.);
#14042=ORIENTED_EDGE('',*,*,#10094,.F.);
#14043=ORIENTED_EDGE('',*,*,#10095,.T.);
#14044=ORIENTED_EDGE('',*,*,#10096,.T.);
#14045=ORIENTED_EDGE('',*,*,#10092,.F.);
#14046=ORIENTED_EDGE('',*,*,#10097,.F.);
#14047=ORIENTED_EDGE('',*,*,#10098,.T.);
#14048=ORIENTED_EDGE('',*,*,#10099,.T.);
#14049=ORIENTED_EDGE('',*,*,#10095,.F.);
#14050=ORIENTED_EDGE('',*,*,#10100,.F.);
#14051=ORIENTED_EDGE('',*,*,#10101,.T.);
#14052=ORIENTED_EDGE('',*,*,#10102,.T.);
#14053=ORIENTED_EDGE('',*,*,#10098,.F.);
#14054=ORIENTED_EDGE('',*,*,#10103,.F.);
#14055=ORIENTED_EDGE('',*,*,#10104,.T.);
#14056=ORIENTED_EDGE('',*,*,#10105,.T.);
#14057=ORIENTED_EDGE('',*,*,#10101,.F.);
#14058=ORIENTED_EDGE('',*,*,#10106,.F.);
#14059=ORIENTED_EDGE('',*,*,#10107,.T.);
#14060=ORIENTED_EDGE('',*,*,#10108,.T.);
#14061=ORIENTED_EDGE('',*,*,#10104,.F.);
#14062=ORIENTED_EDGE('',*,*,#10109,.F.);
#14063=ORIENTED_EDGE('',*,*,#10081,.T.);
#14064=ORIENTED_EDGE('',*,*,#10110,.T.);
#14065=ORIENTED_EDGE('',*,*,#10107,.F.);
#14066=ORIENTED_EDGE('',*,*,#10110,.F.);
#14067=ORIENTED_EDGE('',*,*,#10080,.F.);
#14068=ORIENTED_EDGE('',*,*,#10084,.F.);
#14069=ORIENTED_EDGE('',*,*,#10087,.F.);
#14070=ORIENTED_EDGE('',*,*,#10090,.F.);
#14071=ORIENTED_EDGE('',*,*,#10093,.F.);
#14072=ORIENTED_EDGE('',*,*,#10096,.F.);
#14073=ORIENTED_EDGE('',*,*,#10099,.F.);
#14074=ORIENTED_EDGE('',*,*,#10102,.F.);
#14075=ORIENTED_EDGE('',*,*,#10105,.F.);
#14076=ORIENTED_EDGE('',*,*,#10108,.F.);
#14077=ORIENTED_EDGE('',*,*,#10111,.F.);
#14078=ORIENTED_EDGE('',*,*,#10112,.T.);
#14079=ORIENTED_EDGE('',*,*,#10113,.T.);
#14080=ORIENTED_EDGE('',*,*,#10114,.F.);
#14081=ORIENTED_EDGE('',*,*,#10115,.F.);
#14082=ORIENTED_EDGE('',*,*,#10116,.T.);
#14083=ORIENTED_EDGE('',*,*,#10117,.T.);
#14084=ORIENTED_EDGE('',*,*,#10112,.F.);
#14085=ORIENTED_EDGE('',*,*,#10118,.F.);
#14086=ORIENTED_EDGE('',*,*,#10119,.T.);
#14087=ORIENTED_EDGE('',*,*,#10120,.T.);
#14088=ORIENTED_EDGE('',*,*,#10116,.F.);
#14089=ORIENTED_EDGE('',*,*,#10121,.F.);
#14090=ORIENTED_EDGE('',*,*,#10122,.T.);
#14091=ORIENTED_EDGE('',*,*,#10123,.T.);
#14092=ORIENTED_EDGE('',*,*,#10119,.F.);
#14093=ORIENTED_EDGE('',*,*,#10124,.F.);
#14094=ORIENTED_EDGE('',*,*,#10125,.T.);
#14095=ORIENTED_EDGE('',*,*,#10126,.T.);
#14096=ORIENTED_EDGE('',*,*,#10122,.F.);
#14097=ORIENTED_EDGE('',*,*,#10127,.F.);
#14098=ORIENTED_EDGE('',*,*,#10128,.T.);
#14099=ORIENTED_EDGE('',*,*,#10129,.T.);
#14100=ORIENTED_EDGE('',*,*,#10125,.F.);
#14101=ORIENTED_EDGE('',*,*,#10130,.F.);
#14102=ORIENTED_EDGE('',*,*,#10131,.T.);
#14103=ORIENTED_EDGE('',*,*,#10132,.T.);
#14104=ORIENTED_EDGE('',*,*,#10128,.F.);
#14105=ORIENTED_EDGE('',*,*,#10133,.F.);
#14106=ORIENTED_EDGE('',*,*,#10134,.T.);
#14107=ORIENTED_EDGE('',*,*,#10135,.T.);
#14108=ORIENTED_EDGE('',*,*,#10131,.F.);
#14109=ORIENTED_EDGE('',*,*,#10136,.F.);
#14110=ORIENTED_EDGE('',*,*,#10137,.T.);
#14111=ORIENTED_EDGE('',*,*,#10138,.T.);
#14112=ORIENTED_EDGE('',*,*,#10134,.F.);
#14113=ORIENTED_EDGE('',*,*,#10139,.F.);
#14114=ORIENTED_EDGE('',*,*,#10114,.T.);
#14115=ORIENTED_EDGE('',*,*,#10140,.T.);
#14116=ORIENTED_EDGE('',*,*,#10137,.F.);
#14117=ORIENTED_EDGE('',*,*,#10140,.F.);
#14118=ORIENTED_EDGE('',*,*,#10113,.F.);
#14119=ORIENTED_EDGE('',*,*,#10117,.F.);
#14120=ORIENTED_EDGE('',*,*,#10120,.F.);
#14121=ORIENTED_EDGE('',*,*,#10123,.F.);
#14122=ORIENTED_EDGE('',*,*,#10126,.F.);
#14123=ORIENTED_EDGE('',*,*,#10129,.F.);
#14124=ORIENTED_EDGE('',*,*,#10132,.F.);
#14125=ORIENTED_EDGE('',*,*,#10135,.F.);
#14126=ORIENTED_EDGE('',*,*,#10138,.F.);
#14127=ORIENTED_EDGE('',*,*,#10141,.F.);
#14128=ORIENTED_EDGE('',*,*,#10142,.T.);
#14129=ORIENTED_EDGE('',*,*,#10143,.T.);
#14130=ORIENTED_EDGE('',*,*,#10144,.F.);
#14131=ORIENTED_EDGE('',*,*,#10145,.F.);
#14132=ORIENTED_EDGE('',*,*,#10146,.T.);
#14133=ORIENTED_EDGE('',*,*,#10147,.T.);
#14134=ORIENTED_EDGE('',*,*,#10142,.F.);
#14135=ORIENTED_EDGE('',*,*,#10148,.F.);
#14136=ORIENTED_EDGE('',*,*,#10149,.T.);
#14137=ORIENTED_EDGE('',*,*,#10150,.T.);
#14138=ORIENTED_EDGE('',*,*,#10146,.F.);
#14139=ORIENTED_EDGE('',*,*,#10151,.F.);
#14140=ORIENTED_EDGE('',*,*,#10152,.T.);
#14141=ORIENTED_EDGE('',*,*,#10153,.T.);
#14142=ORIENTED_EDGE('',*,*,#10149,.F.);
#14143=ORIENTED_EDGE('',*,*,#10154,.F.);
#14144=ORIENTED_EDGE('',*,*,#10155,.T.);
#14145=ORIENTED_EDGE('',*,*,#10156,.T.);
#14146=ORIENTED_EDGE('',*,*,#10152,.F.);
#14147=ORIENTED_EDGE('',*,*,#10157,.F.);
#14148=ORIENTED_EDGE('',*,*,#10158,.T.);
#14149=ORIENTED_EDGE('',*,*,#10159,.T.);
#14150=ORIENTED_EDGE('',*,*,#10155,.F.);
#14151=ORIENTED_EDGE('',*,*,#10160,.F.);
#14152=ORIENTED_EDGE('',*,*,#10161,.T.);
#14153=ORIENTED_EDGE('',*,*,#10162,.T.);
#14154=ORIENTED_EDGE('',*,*,#10158,.F.);
#14155=ORIENTED_EDGE('',*,*,#10163,.F.);
#14156=ORIENTED_EDGE('',*,*,#10164,.T.);
#14157=ORIENTED_EDGE('',*,*,#10165,.T.);
#14158=ORIENTED_EDGE('',*,*,#10161,.F.);
#14159=ORIENTED_EDGE('',*,*,#10166,.F.);
#14160=ORIENTED_EDGE('',*,*,#10167,.T.);
#14161=ORIENTED_EDGE('',*,*,#10168,.T.);
#14162=ORIENTED_EDGE('',*,*,#10164,.F.);
#14163=ORIENTED_EDGE('',*,*,#10169,.F.);
#14164=ORIENTED_EDGE('',*,*,#10170,.T.);
#14165=ORIENTED_EDGE('',*,*,#10171,.T.);
#14166=ORIENTED_EDGE('',*,*,#10167,.F.);
#14167=ORIENTED_EDGE('',*,*,#10172,.F.);
#14168=ORIENTED_EDGE('',*,*,#10144,.T.);
#14169=ORIENTED_EDGE('',*,*,#10173,.T.);
#14170=ORIENTED_EDGE('',*,*,#10170,.F.);
#14171=ORIENTED_EDGE('',*,*,#10173,.F.);
#14172=ORIENTED_EDGE('',*,*,#10143,.F.);
#14173=ORIENTED_EDGE('',*,*,#10147,.F.);
#14174=ORIENTED_EDGE('',*,*,#10150,.F.);
#14175=ORIENTED_EDGE('',*,*,#10153,.F.);
#14176=ORIENTED_EDGE('',*,*,#10156,.F.);
#14177=ORIENTED_EDGE('',*,*,#10159,.F.);
#14178=ORIENTED_EDGE('',*,*,#10162,.F.);
#14179=ORIENTED_EDGE('',*,*,#10165,.F.);
#14180=ORIENTED_EDGE('',*,*,#10168,.F.);
#14181=ORIENTED_EDGE('',*,*,#10171,.F.);
#14182=ORIENTED_EDGE('',*,*,#10174,.F.);
#14183=ORIENTED_EDGE('',*,*,#10175,.T.);
#14184=ORIENTED_EDGE('',*,*,#10176,.T.);
#14185=ORIENTED_EDGE('',*,*,#10177,.F.);
#14186=ORIENTED_EDGE('',*,*,#10178,.F.);
#14187=ORIENTED_EDGE('',*,*,#10179,.T.);
#14188=ORIENTED_EDGE('',*,*,#10180,.T.);
#14189=ORIENTED_EDGE('',*,*,#10175,.F.);
#14190=ORIENTED_EDGE('',*,*,#10181,.F.);
#14191=ORIENTED_EDGE('',*,*,#10182,.T.);
#14192=ORIENTED_EDGE('',*,*,#10183,.T.);
#14193=ORIENTED_EDGE('',*,*,#10179,.F.);
#14194=ORIENTED_EDGE('',*,*,#10184,.F.);
#14195=ORIENTED_EDGE('',*,*,#10185,.T.);
#14196=ORIENTED_EDGE('',*,*,#10186,.T.);
#14197=ORIENTED_EDGE('',*,*,#10182,.F.);
#14198=ORIENTED_EDGE('',*,*,#10187,.F.);
#14199=ORIENTED_EDGE('',*,*,#10188,.T.);
#14200=ORIENTED_EDGE('',*,*,#10189,.T.);
#14201=ORIENTED_EDGE('',*,*,#10185,.F.);
#14202=ORIENTED_EDGE('',*,*,#10190,.F.);
#14203=ORIENTED_EDGE('',*,*,#10191,.T.);
#14204=ORIENTED_EDGE('',*,*,#10192,.T.);
#14205=ORIENTED_EDGE('',*,*,#10188,.F.);
#14206=ORIENTED_EDGE('',*,*,#10193,.F.);
#14207=ORIENTED_EDGE('',*,*,#10194,.T.);
#14208=ORIENTED_EDGE('',*,*,#10195,.T.);
#14209=ORIENTED_EDGE('',*,*,#10191,.F.);
#14210=ORIENTED_EDGE('',*,*,#10196,.F.);
#14211=ORIENTED_EDGE('',*,*,#10197,.T.);
#14212=ORIENTED_EDGE('',*,*,#10198,.T.);
#14213=ORIENTED_EDGE('',*,*,#10194,.F.);
#14214=ORIENTED_EDGE('',*,*,#10199,.F.);
#14215=ORIENTED_EDGE('',*,*,#10200,.T.);
#14216=ORIENTED_EDGE('',*,*,#10201,.T.);
#14217=ORIENTED_EDGE('',*,*,#10197,.F.);
#14218=ORIENTED_EDGE('',*,*,#10202,.F.);
#14219=ORIENTED_EDGE('',*,*,#10177,.T.);
#14220=ORIENTED_EDGE('',*,*,#10203,.T.);
#14221=ORIENTED_EDGE('',*,*,#10200,.F.);
#14222=ORIENTED_EDGE('',*,*,#10203,.F.);
#14223=ORIENTED_EDGE('',*,*,#10176,.F.);
#14224=ORIENTED_EDGE('',*,*,#10180,.F.);
#14225=ORIENTED_EDGE('',*,*,#10183,.F.);
#14226=ORIENTED_EDGE('',*,*,#10186,.F.);
#14227=ORIENTED_EDGE('',*,*,#10189,.F.);
#14228=ORIENTED_EDGE('',*,*,#10192,.F.);
#14229=ORIENTED_EDGE('',*,*,#10195,.F.);
#14230=ORIENTED_EDGE('',*,*,#10198,.F.);
#14231=ORIENTED_EDGE('',*,*,#10201,.F.);
#14232=ORIENTED_EDGE('',*,*,#10204,.F.);
#14233=ORIENTED_EDGE('',*,*,#10205,.T.);
#14234=ORIENTED_EDGE('',*,*,#10206,.T.);
#14235=ORIENTED_EDGE('',*,*,#10207,.F.);
#14236=ORIENTED_EDGE('',*,*,#10208,.F.);
#14237=ORIENTED_EDGE('',*,*,#10209,.T.);
#14238=ORIENTED_EDGE('',*,*,#10210,.T.);
#14239=ORIENTED_EDGE('',*,*,#10205,.F.);
#14240=ORIENTED_EDGE('',*,*,#10211,.F.);
#14241=ORIENTED_EDGE('',*,*,#10212,.T.);
#14242=ORIENTED_EDGE('',*,*,#10213,.T.);
#14243=ORIENTED_EDGE('',*,*,#10209,.F.);
#14244=ORIENTED_EDGE('',*,*,#10214,.F.);
#14245=ORIENTED_EDGE('',*,*,#10215,.T.);
#14246=ORIENTED_EDGE('',*,*,#10216,.T.);
#14247=ORIENTED_EDGE('',*,*,#10212,.F.);
#14248=ORIENTED_EDGE('',*,*,#10217,.F.);
#14249=ORIENTED_EDGE('',*,*,#10218,.T.);
#14250=ORIENTED_EDGE('',*,*,#10219,.T.);
#14251=ORIENTED_EDGE('',*,*,#10215,.F.);
#14252=ORIENTED_EDGE('',*,*,#10220,.F.);
#14253=ORIENTED_EDGE('',*,*,#10221,.T.);
#14254=ORIENTED_EDGE('',*,*,#10222,.T.);
#14255=ORIENTED_EDGE('',*,*,#10218,.F.);
#14256=ORIENTED_EDGE('',*,*,#10223,.F.);
#14257=ORIENTED_EDGE('',*,*,#10224,.T.);
#14258=ORIENTED_EDGE('',*,*,#10225,.T.);
#14259=ORIENTED_EDGE('',*,*,#10221,.F.);
#14260=ORIENTED_EDGE('',*,*,#10226,.F.);
#14261=ORIENTED_EDGE('',*,*,#10227,.T.);
#14262=ORIENTED_EDGE('',*,*,#10228,.T.);
#14263=ORIENTED_EDGE('',*,*,#10224,.F.);
#14264=ORIENTED_EDGE('',*,*,#10229,.F.);
#14265=ORIENTED_EDGE('',*,*,#10230,.T.);
#14266=ORIENTED_EDGE('',*,*,#10231,.T.);
#14267=ORIENTED_EDGE('',*,*,#10227,.F.);
#14268=ORIENTED_EDGE('',*,*,#10232,.F.);
#14269=ORIENTED_EDGE('',*,*,#10207,.T.);
#14270=ORIENTED_EDGE('',*,*,#10233,.T.);
#14271=ORIENTED_EDGE('',*,*,#10230,.F.);
#14272=ORIENTED_EDGE('',*,*,#10233,.F.);
#14273=ORIENTED_EDGE('',*,*,#10206,.F.);
#14274=ORIENTED_EDGE('',*,*,#10210,.F.);
#14275=ORIENTED_EDGE('',*,*,#10213,.F.);
#14276=ORIENTED_EDGE('',*,*,#10216,.F.);
#14277=ORIENTED_EDGE('',*,*,#10219,.F.);
#14278=ORIENTED_EDGE('',*,*,#10222,.F.);
#14279=ORIENTED_EDGE('',*,*,#10225,.F.);
#14280=ORIENTED_EDGE('',*,*,#10228,.F.);
#14281=ORIENTED_EDGE('',*,*,#10231,.F.);
#14282=ORIENTED_EDGE('',*,*,#10234,.T.);
#14283=ORIENTED_EDGE('',*,*,#10235,.F.);
#14284=ORIENTED_EDGE('',*,*,#10234,.F.);
#14285=ORIENTED_EDGE('',*,*,#10236,.T.);
#14286=ORIENTED_EDGE('',*,*,#10237,.F.);
#14287=ORIENTED_EDGE('',*,*,#10236,.F.);
#14288=ORIENTED_EDGE('',*,*,#10235,.T.);
#14289=ORIENTED_EDGE('',*,*,#10238,.T.);
#14290=ORIENTED_EDGE('',*,*,#10239,.F.);
#14291=ORIENTED_EDGE('',*,*,#10238,.F.);
#14292=ORIENTED_EDGE('',*,*,#10239,.T.);
#14293=ORIENTED_EDGE('',*,*,#10240,.F.);
#14294=ORIENTED_EDGE('',*,*,#10241,.T.);
#14295=ORIENTED_EDGE('',*,*,#10242,.F.);
#14296=ORIENTED_EDGE('',*,*,#10243,.F.);
#14297=ORIENTED_EDGE('',*,*,#10244,.F.);
#14298=ORIENTED_EDGE('',*,*,#10243,.T.);
#14299=ORIENTED_EDGE('',*,*,#10245,.T.);
#14300=ORIENTED_EDGE('',*,*,#10246,.F.);
#14301=ORIENTED_EDGE('',*,*,#10245,.F.);
#14302=ORIENTED_EDGE('',*,*,#10242,.T.);
#14303=ORIENTED_EDGE('',*,*,#10247,.T.);
#14304=ORIENTED_EDGE('',*,*,#10248,.F.);
#14305=ORIENTED_EDGE('',*,*,#10247,.F.);
#14306=ORIENTED_EDGE('',*,*,#10241,.F.);
#14307=ORIENTED_EDGE('',*,*,#10249,.F.);
#14308=ORIENTED_EDGE('',*,*,#10250,.T.);
#14309=ORIENTED_EDGE('',*,*,#10251,.F.);
#14310=ORIENTED_EDGE('',*,*,#10252,.F.);
#14311=ORIENTED_EDGE('',*,*,#10253,.F.);
#14312=ORIENTED_EDGE('',*,*,#10252,.T.);
#14313=ORIENTED_EDGE('',*,*,#10254,.T.);
#14314=ORIENTED_EDGE('',*,*,#10255,.F.);
#14315=ORIENTED_EDGE('',*,*,#10254,.F.);
#14316=ORIENTED_EDGE('',*,*,#10251,.T.);
#14317=ORIENTED_EDGE('',*,*,#10256,.T.);
#14318=ORIENTED_EDGE('',*,*,#10257,.F.);
#14319=ORIENTED_EDGE('',*,*,#10256,.F.);
#14320=ORIENTED_EDGE('',*,*,#10250,.F.);
#14321=ORIENTED_EDGE('',*,*,#10258,.F.);
#14322=ORIENTED_EDGE('',*,*,#10259,.T.);
#14323=ORIENTED_EDGE('',*,*,#10260,.F.);
#14324=ORIENTED_EDGE('',*,*,#10261,.F.);
#14325=ORIENTED_EDGE('',*,*,#10262,.F.);
#14326=ORIENTED_EDGE('',*,*,#10261,.T.);
#14327=ORIENTED_EDGE('',*,*,#10263,.T.);
#14328=ORIENTED_EDGE('',*,*,#10264,.F.);
#14329=ORIENTED_EDGE('',*,*,#10263,.F.);
#14330=ORIENTED_EDGE('',*,*,#10260,.T.);
#14331=ORIENTED_EDGE('',*,*,#10265,.T.);
#14332=ORIENTED_EDGE('',*,*,#10266,.F.);
#14333=ORIENTED_EDGE('',*,*,#10265,.F.);
#14334=ORIENTED_EDGE('',*,*,#10259,.F.);
#14335=ORIENTED_EDGE('',*,*,#10267,.F.);
#14336=ORIENTED_EDGE('',*,*,#10268,.T.);
#14337=ORIENTED_EDGE('',*,*,#10269,.F.);
#14338=ORIENTED_EDGE('',*,*,#10270,.F.);
#14339=ORIENTED_EDGE('',*,*,#10271,.F.);
#14340=ORIENTED_EDGE('',*,*,#10270,.T.);
#14341=ORIENTED_EDGE('',*,*,#10272,.T.);
#14342=ORIENTED_EDGE('',*,*,#10273,.F.);
#14343=ORIENTED_EDGE('',*,*,#10272,.F.);
#14344=ORIENTED_EDGE('',*,*,#10269,.T.);
#14345=ORIENTED_EDGE('',*,*,#10274,.T.);
#14346=ORIENTED_EDGE('',*,*,#10275,.F.);
#14347=ORIENTED_EDGE('',*,*,#10274,.F.);
#14348=ORIENTED_EDGE('',*,*,#10268,.F.);
#14349=ORIENTED_EDGE('',*,*,#10276,.F.);
#14350=ORIENTED_EDGE('',*,*,#10277,.T.);
#14351=ORIENTED_EDGE('',*,*,#10278,.F.);
#14352=ORIENTED_EDGE('',*,*,#10279,.F.);
#14353=ORIENTED_EDGE('',*,*,#10280,.F.);
#14354=ORIENTED_EDGE('',*,*,#10279,.T.);
#14355=ORIENTED_EDGE('',*,*,#10281,.T.);
#14356=ORIENTED_EDGE('',*,*,#10282,.F.);
#14357=ORIENTED_EDGE('',*,*,#10281,.F.);
#14358=ORIENTED_EDGE('',*,*,#10278,.T.);
#14359=ORIENTED_EDGE('',*,*,#10283,.T.);
#14360=ORIENTED_EDGE('',*,*,#10284,.F.);
#14361=ORIENTED_EDGE('',*,*,#10283,.F.);
#14362=ORIENTED_EDGE('',*,*,#10277,.F.);
#14363=ORIENTED_EDGE('',*,*,#10285,.F.);
#14364=ORIENTED_EDGE('',*,*,#10286,.T.);
#14365=ORIENTED_EDGE('',*,*,#10287,.F.);
#14366=ORIENTED_EDGE('',*,*,#10288,.F.);
#14367=ORIENTED_EDGE('',*,*,#10289,.F.);
#14368=ORIENTED_EDGE('',*,*,#10288,.T.);
#14369=ORIENTED_EDGE('',*,*,#10290,.T.);
#14370=ORIENTED_EDGE('',*,*,#10291,.F.);
#14371=ORIENTED_EDGE('',*,*,#10290,.F.);
#14372=ORIENTED_EDGE('',*,*,#10287,.T.);
#14373=ORIENTED_EDGE('',*,*,#10292,.T.);
#14374=ORIENTED_EDGE('',*,*,#10293,.F.);
#14375=ORIENTED_EDGE('',*,*,#10292,.F.);
#14376=ORIENTED_EDGE('',*,*,#10286,.F.);
#14377=ORIENTED_EDGE('',*,*,#10294,.F.);
#14378=ORIENTED_EDGE('',*,*,#10295,.T.);
#14379=ORIENTED_EDGE('',*,*,#10296,.F.);
#14380=ORIENTED_EDGE('',*,*,#10297,.F.);
#14381=ORIENTED_EDGE('',*,*,#10298,.F.);
#14382=ORIENTED_EDGE('',*,*,#10297,.T.);
#14383=ORIENTED_EDGE('',*,*,#10299,.T.);
#14384=ORIENTED_EDGE('',*,*,#10300,.F.);
#14385=ORIENTED_EDGE('',*,*,#10299,.F.);
#14386=ORIENTED_EDGE('',*,*,#10296,.T.);
#14387=ORIENTED_EDGE('',*,*,#10301,.T.);
#14388=ORIENTED_EDGE('',*,*,#10302,.F.);
#14389=ORIENTED_EDGE('',*,*,#10301,.F.);
#14390=ORIENTED_EDGE('',*,*,#10295,.F.);
#14391=ORIENTED_EDGE('',*,*,#10303,.F.);
#14392=ORIENTED_EDGE('',*,*,#10304,.T.);
#14393=ORIENTED_EDGE('',*,*,#10305,.F.);
#14394=ORIENTED_EDGE('',*,*,#10306,.F.);
#14395=ORIENTED_EDGE('',*,*,#10307,.F.);
#14396=ORIENTED_EDGE('',*,*,#10306,.T.);
#14397=ORIENTED_EDGE('',*,*,#10308,.T.);
#14398=ORIENTED_EDGE('',*,*,#10309,.F.);
#14399=ORIENTED_EDGE('',*,*,#10308,.F.);
#14400=ORIENTED_EDGE('',*,*,#10305,.T.);
#14401=ORIENTED_EDGE('',*,*,#10310,.T.);
#14402=ORIENTED_EDGE('',*,*,#10311,.F.);
#14403=ORIENTED_EDGE('',*,*,#10310,.F.);
#14404=ORIENTED_EDGE('',*,*,#10304,.F.);
#14405=ORIENTED_EDGE('',*,*,#10312,.F.);
#14406=ORIENTED_EDGE('',*,*,#10313,.T.);
#14407=ORIENTED_EDGE('',*,*,#10314,.F.);
#14408=ORIENTED_EDGE('',*,*,#10315,.F.);
#14409=ORIENTED_EDGE('',*,*,#10316,.F.);
#14410=ORIENTED_EDGE('',*,*,#10315,.T.);
#14411=ORIENTED_EDGE('',*,*,#10317,.T.);
#14412=ORIENTED_EDGE('',*,*,#10318,.F.);
#14413=ORIENTED_EDGE('',*,*,#10317,.F.);
#14414=ORIENTED_EDGE('',*,*,#10314,.T.);
#14415=ORIENTED_EDGE('',*,*,#10319,.T.);
#14416=ORIENTED_EDGE('',*,*,#10320,.F.);
#14417=ORIENTED_EDGE('',*,*,#10319,.F.);
#14418=ORIENTED_EDGE('',*,*,#10313,.F.);
#14419=ORIENTED_EDGE('',*,*,#10321,.F.);
#14420=ORIENTED_EDGE('',*,*,#10322,.T.);
#14421=ORIENTED_EDGE('',*,*,#10323,.F.);
#14422=ORIENTED_EDGE('',*,*,#10324,.F.);
#14423=ORIENTED_EDGE('',*,*,#10325,.F.);
#14424=ORIENTED_EDGE('',*,*,#10324,.T.);
#14425=ORIENTED_EDGE('',*,*,#10326,.T.);
#14426=ORIENTED_EDGE('',*,*,#10327,.F.);
#14427=ORIENTED_EDGE('',*,*,#10326,.F.);
#14428=ORIENTED_EDGE('',*,*,#10323,.T.);
#14429=ORIENTED_EDGE('',*,*,#10328,.T.);
#14430=ORIENTED_EDGE('',*,*,#10329,.F.);
#14431=ORIENTED_EDGE('',*,*,#10328,.F.);
#14432=ORIENTED_EDGE('',*,*,#10322,.F.);
#14433=ORIENTED_EDGE('',*,*,#10330,.F.);
#14434=ORIENTED_EDGE('',*,*,#10331,.T.);
#14435=ORIENTED_EDGE('',*,*,#10332,.F.);
#14436=ORIENTED_EDGE('',*,*,#10333,.F.);
#14437=ORIENTED_EDGE('',*,*,#10334,.F.);
#14438=ORIENTED_EDGE('',*,*,#10333,.T.);
#14439=ORIENTED_EDGE('',*,*,#10335,.T.);
#14440=ORIENTED_EDGE('',*,*,#10336,.F.);
#14441=ORIENTED_EDGE('',*,*,#10335,.F.);
#14442=ORIENTED_EDGE('',*,*,#10332,.T.);
#14443=ORIENTED_EDGE('',*,*,#10337,.T.);
#14444=ORIENTED_EDGE('',*,*,#10338,.F.);
#14445=ORIENTED_EDGE('',*,*,#10337,.F.);
#14446=ORIENTED_EDGE('',*,*,#10331,.F.);
#14447=ORIENTED_EDGE('',*,*,#10339,.F.);
#14448=ORIENTED_EDGE('',*,*,#10340,.T.);
#14449=ORIENTED_EDGE('',*,*,#10341,.F.);
#14450=ORIENTED_EDGE('',*,*,#10342,.F.);
#14451=ORIENTED_EDGE('',*,*,#10343,.F.);
#14452=ORIENTED_EDGE('',*,*,#10342,.T.);
#14453=ORIENTED_EDGE('',*,*,#10344,.T.);
#14454=ORIENTED_EDGE('',*,*,#10345,.F.);
#14455=ORIENTED_EDGE('',*,*,#10344,.F.);
#14456=ORIENTED_EDGE('',*,*,#10341,.T.);
#14457=ORIENTED_EDGE('',*,*,#10346,.T.);
#14458=ORIENTED_EDGE('',*,*,#10347,.F.);
#14459=ORIENTED_EDGE('',*,*,#10346,.F.);
#14460=ORIENTED_EDGE('',*,*,#10340,.F.);
#14461=ORIENTED_EDGE('',*,*,#10348,.F.);
#14462=ORIENTED_EDGE('',*,*,#10349,.T.);
#14463=ORIENTED_EDGE('',*,*,#10350,.F.);
#14464=ORIENTED_EDGE('',*,*,#10351,.F.);
#14465=ORIENTED_EDGE('',*,*,#10352,.F.);
#14466=ORIENTED_EDGE('',*,*,#10351,.T.);
#14467=ORIENTED_EDGE('',*,*,#10353,.T.);
#14468=ORIENTED_EDGE('',*,*,#10354,.F.);
#14469=ORIENTED_EDGE('',*,*,#10353,.F.);
#14470=ORIENTED_EDGE('',*,*,#10350,.T.);
#14471=ORIENTED_EDGE('',*,*,#10355,.T.);
#14472=ORIENTED_EDGE('',*,*,#10356,.F.);
#14473=ORIENTED_EDGE('',*,*,#10355,.F.);
#14474=ORIENTED_EDGE('',*,*,#10349,.F.);
#14475=ORIENTED_EDGE('',*,*,#10357,.F.);
#14476=ORIENTED_EDGE('',*,*,#10358,.T.);
#14477=ORIENTED_EDGE('',*,*,#10359,.F.);
#14478=ORIENTED_EDGE('',*,*,#10360,.F.);
#14479=ORIENTED_EDGE('',*,*,#10361,.F.);
#14480=ORIENTED_EDGE('',*,*,#10360,.T.);
#14481=ORIENTED_EDGE('',*,*,#10362,.T.);
#14482=ORIENTED_EDGE('',*,*,#10363,.F.);
#14483=ORIENTED_EDGE('',*,*,#10362,.F.);
#14484=ORIENTED_EDGE('',*,*,#10359,.T.);
#14485=ORIENTED_EDGE('',*,*,#10364,.T.);
#14486=ORIENTED_EDGE('',*,*,#10365,.F.);
#14487=ORIENTED_EDGE('',*,*,#10364,.F.);
#14488=ORIENTED_EDGE('',*,*,#10358,.F.);
#14489=ORIENTED_EDGE('',*,*,#10366,.F.);
#14490=ORIENTED_EDGE('',*,*,#10367,.T.);
#14491=ORIENTED_EDGE('',*,*,#10368,.F.);
#14492=ORIENTED_EDGE('',*,*,#10369,.F.);
#14493=ORIENTED_EDGE('',*,*,#10370,.F.);
#14494=ORIENTED_EDGE('',*,*,#10369,.T.);
#14495=ORIENTED_EDGE('',*,*,#10371,.T.);
#14496=ORIENTED_EDGE('',*,*,#10372,.F.);
#14497=ORIENTED_EDGE('',*,*,#10373,.F.);
#14498=ORIENTED_EDGE('',*,*,#10371,.F.);
#14499=ORIENTED_EDGE('',*,*,#10368,.T.);
#14500=ORIENTED_EDGE('',*,*,#10374,.T.);
#14501=ORIENTED_EDGE('',*,*,#10375,.F.);
#14502=ORIENTED_EDGE('',*,*,#10374,.F.);
#14503=ORIENTED_EDGE('',*,*,#10367,.F.);
#14504=ORIENTED_EDGE('',*,*,#10376,.F.);
#14505=ORIENTED_EDGE('',*,*,#10377,.F.);
#14506=ORIENTED_EDGE('',*,*,#10378,.T.);
#14507=ORIENTED_EDGE('',*,*,#10379,.F.);
#14508=ORIENTED_EDGE('',*,*,#10380,.F.);
#14509=ORIENTED_EDGE('',*,*,#10381,.F.);
#14510=ORIENTED_EDGE('',*,*,#10380,.T.);
#14511=ORIENTED_EDGE('',*,*,#10382,.T.);
#14512=ORIENTED_EDGE('',*,*,#10383,.F.);
#14513=ORIENTED_EDGE('',*,*,#10382,.F.);
#14514=ORIENTED_EDGE('',*,*,#10379,.T.);
#14515=ORIENTED_EDGE('',*,*,#10384,.T.);
#14516=ORIENTED_EDGE('',*,*,#10385,.F.);
#14517=ORIENTED_EDGE('',*,*,#10384,.F.);
#14518=ORIENTED_EDGE('',*,*,#10378,.F.);
#14519=ORIENTED_EDGE('',*,*,#10386,.F.);
#14520=ORIENTED_EDGE('',*,*,#10387,.T.);
#14521=ORIENTED_EDGE('',*,*,#10388,.F.);
#14522=ORIENTED_EDGE('',*,*,#10389,.F.);
#14523=ORIENTED_EDGE('',*,*,#10390,.F.);
#14524=ORIENTED_EDGE('',*,*,#10389,.T.);
#14525=ORIENTED_EDGE('',*,*,#10391,.T.);
#14526=ORIENTED_EDGE('',*,*,#10392,.F.);
#14527=ORIENTED_EDGE('',*,*,#10391,.F.);
#14528=ORIENTED_EDGE('',*,*,#10388,.T.);
#14529=ORIENTED_EDGE('',*,*,#10393,.T.);
#14530=ORIENTED_EDGE('',*,*,#10394,.F.);
#14531=ORIENTED_EDGE('',*,*,#10393,.F.);
#14532=ORIENTED_EDGE('',*,*,#10387,.F.);
#14533=ORIENTED_EDGE('',*,*,#10395,.F.);
#14534=ORIENTED_EDGE('',*,*,#10396,.T.);
#14535=ORIENTED_EDGE('',*,*,#10397,.F.);
#14536=ORIENTED_EDGE('',*,*,#10398,.F.);
#14537=ORIENTED_EDGE('',*,*,#10399,.F.);
#14538=ORIENTED_EDGE('',*,*,#10398,.T.);
#14539=ORIENTED_EDGE('',*,*,#10400,.T.);
#14540=ORIENTED_EDGE('',*,*,#10401,.F.);
#14541=ORIENTED_EDGE('',*,*,#10400,.F.);
#14542=ORIENTED_EDGE('',*,*,#10397,.T.);
#14543=ORIENTED_EDGE('',*,*,#10402,.T.);
#14544=ORIENTED_EDGE('',*,*,#10403,.F.);
#14545=ORIENTED_EDGE('',*,*,#10402,.F.);
#14546=ORIENTED_EDGE('',*,*,#10396,.F.);
#14547=ORIENTED_EDGE('',*,*,#10404,.F.);
#14548=ORIENTED_EDGE('',*,*,#10405,.T.);
#14549=ORIENTED_EDGE('',*,*,#10406,.F.);
#14550=ORIENTED_EDGE('',*,*,#10407,.F.);
#14551=ORIENTED_EDGE('',*,*,#10408,.F.);
#14552=ORIENTED_EDGE('',*,*,#10407,.T.);
#14553=ORIENTED_EDGE('',*,*,#10409,.T.);
#14554=ORIENTED_EDGE('',*,*,#10410,.F.);
#14555=ORIENTED_EDGE('',*,*,#10409,.F.);
#14556=ORIENTED_EDGE('',*,*,#10406,.T.);
#14557=ORIENTED_EDGE('',*,*,#10411,.T.);
#14558=ORIENTED_EDGE('',*,*,#10412,.F.);
#14559=ORIENTED_EDGE('',*,*,#10411,.F.);
#14560=ORIENTED_EDGE('',*,*,#10405,.F.);
#14561=ORIENTED_EDGE('',*,*,#10413,.F.);
#14562=ORIENTED_EDGE('',*,*,#10414,.T.);
#14563=ORIENTED_EDGE('',*,*,#10415,.F.);
#14564=ORIENTED_EDGE('',*,*,#10416,.F.);
#14565=ORIENTED_EDGE('',*,*,#10417,.F.);
#14566=ORIENTED_EDGE('',*,*,#10416,.T.);
#14567=ORIENTED_EDGE('',*,*,#10418,.T.);
#14568=ORIENTED_EDGE('',*,*,#10419,.F.);
#14569=ORIENTED_EDGE('',*,*,#10418,.F.);
#14570=ORIENTED_EDGE('',*,*,#10415,.T.);
#14571=ORIENTED_EDGE('',*,*,#10420,.T.);
#14572=ORIENTED_EDGE('',*,*,#10421,.F.);
#14573=ORIENTED_EDGE('',*,*,#10420,.F.);
#14574=ORIENTED_EDGE('',*,*,#10414,.F.);
#14575=ORIENTED_EDGE('',*,*,#10422,.F.);
#14576=ORIENTED_EDGE('',*,*,#10423,.T.);
#14577=ORIENTED_EDGE('',*,*,#10424,.F.);
#14578=ORIENTED_EDGE('',*,*,#10425,.F.);
#14579=ORIENTED_EDGE('',*,*,#10426,.F.);
#14580=ORIENTED_EDGE('',*,*,#10425,.T.);
#14581=ORIENTED_EDGE('',*,*,#10427,.T.);
#14582=ORIENTED_EDGE('',*,*,#10428,.F.);
#14583=ORIENTED_EDGE('',*,*,#10427,.F.);
#14584=ORIENTED_EDGE('',*,*,#10424,.T.);
#14585=ORIENTED_EDGE('',*,*,#10429,.T.);
#14586=ORIENTED_EDGE('',*,*,#10430,.F.);
#14587=ORIENTED_EDGE('',*,*,#10429,.F.);
#14588=ORIENTED_EDGE('',*,*,#10423,.F.);
#14589=ORIENTED_EDGE('',*,*,#10431,.F.);
#14590=ORIENTED_EDGE('',*,*,#10432,.T.);
#14591=ORIENTED_EDGE('',*,*,#10433,.F.);
#14592=ORIENTED_EDGE('',*,*,#10434,.F.);
#14593=ORIENTED_EDGE('',*,*,#10435,.F.);
#14594=ORIENTED_EDGE('',*,*,#10434,.T.);
#14595=ORIENTED_EDGE('',*,*,#10436,.T.);
#14596=ORIENTED_EDGE('',*,*,#10437,.F.);
#14597=ORIENTED_EDGE('',*,*,#10436,.F.);
#14598=ORIENTED_EDGE('',*,*,#10433,.T.);
#14599=ORIENTED_EDGE('',*,*,#10438,.T.);
#14600=ORIENTED_EDGE('',*,*,#10439,.F.);
#14601=ORIENTED_EDGE('',*,*,#10438,.F.);
#14602=ORIENTED_EDGE('',*,*,#10432,.F.);
#14603=ORIENTED_EDGE('',*,*,#10440,.F.);
#14604=ORIENTED_EDGE('',*,*,#10441,.T.);
#14605=ORIENTED_EDGE('',*,*,#10442,.F.);
#14606=ORIENTED_EDGE('',*,*,#10443,.F.);
#14607=ORIENTED_EDGE('',*,*,#10444,.F.);
#14608=ORIENTED_EDGE('',*,*,#10443,.T.);
#14609=ORIENTED_EDGE('',*,*,#10445,.T.);
#14610=ORIENTED_EDGE('',*,*,#10446,.F.);
#14611=ORIENTED_EDGE('',*,*,#10445,.F.);
#14612=ORIENTED_EDGE('',*,*,#10442,.T.);
#14613=ORIENTED_EDGE('',*,*,#10447,.T.);
#14614=ORIENTED_EDGE('',*,*,#10448,.F.);
#14615=ORIENTED_EDGE('',*,*,#10447,.F.);
#14616=ORIENTED_EDGE('',*,*,#10441,.F.);
#14617=ORIENTED_EDGE('',*,*,#10449,.F.);
#14618=ORIENTED_EDGE('',*,*,#10450,.T.);
#14619=ORIENTED_EDGE('',*,*,#10451,.F.);
#14620=ORIENTED_EDGE('',*,*,#10452,.F.);
#14621=ORIENTED_EDGE('',*,*,#10453,.F.);
#14622=ORIENTED_EDGE('',*,*,#10452,.T.);
#14623=ORIENTED_EDGE('',*,*,#10454,.T.);
#14624=ORIENTED_EDGE('',*,*,#10455,.F.);
#14625=ORIENTED_EDGE('',*,*,#10454,.F.);
#14626=ORIENTED_EDGE('',*,*,#10451,.T.);
#14627=ORIENTED_EDGE('',*,*,#10456,.T.);
#14628=ORIENTED_EDGE('',*,*,#10457,.F.);
#14629=ORIENTED_EDGE('',*,*,#10456,.F.);
#14630=ORIENTED_EDGE('',*,*,#10450,.F.);
#14631=ORIENTED_EDGE('',*,*,#10458,.F.);
#14632=ORIENTED_EDGE('',*,*,#10459,.T.);
#14633=ORIENTED_EDGE('',*,*,#10460,.F.);
#14634=ORIENTED_EDGE('',*,*,#10461,.F.);
#14635=ORIENTED_EDGE('',*,*,#10462,.F.);
#14636=ORIENTED_EDGE('',*,*,#10461,.T.);
#14637=ORIENTED_EDGE('',*,*,#10463,.T.);
#14638=ORIENTED_EDGE('',*,*,#10464,.F.);
#14639=ORIENTED_EDGE('',*,*,#10463,.F.);
#14640=ORIENTED_EDGE('',*,*,#10460,.T.);
#14641=ORIENTED_EDGE('',*,*,#10465,.T.);
#14642=ORIENTED_EDGE('',*,*,#10466,.F.);
#14643=ORIENTED_EDGE('',*,*,#10465,.F.);
#14644=ORIENTED_EDGE('',*,*,#10459,.F.);
#14645=ORIENTED_EDGE('',*,*,#10467,.F.);
#14646=ORIENTED_EDGE('',*,*,#10468,.T.);
#14647=ORIENTED_EDGE('',*,*,#10469,.F.);
#14648=ORIENTED_EDGE('',*,*,#10470,.F.);
#14649=ORIENTED_EDGE('',*,*,#10471,.F.);
#14650=ORIENTED_EDGE('',*,*,#10470,.T.);
#14651=ORIENTED_EDGE('',*,*,#10472,.T.);
#14652=ORIENTED_EDGE('',*,*,#10473,.F.);
#14653=ORIENTED_EDGE('',*,*,#10472,.F.);
#14654=ORIENTED_EDGE('',*,*,#10469,.T.);
#14655=ORIENTED_EDGE('',*,*,#10474,.T.);
#14656=ORIENTED_EDGE('',*,*,#10475,.F.);
#14657=ORIENTED_EDGE('',*,*,#10474,.F.);
#14658=ORIENTED_EDGE('',*,*,#10468,.F.);
#14659=ORIENTED_EDGE('',*,*,#10476,.F.);
#14660=ORIENTED_EDGE('',*,*,#10477,.T.);
#14661=ORIENTED_EDGE('',*,*,#10478,.F.);
#14662=ORIENTED_EDGE('',*,*,#10479,.F.);
#14663=ORIENTED_EDGE('',*,*,#10480,.F.);
#14664=ORIENTED_EDGE('',*,*,#10479,.T.);
#14665=ORIENTED_EDGE('',*,*,#10481,.T.);
#14666=ORIENTED_EDGE('',*,*,#10482,.F.);
#14667=ORIENTED_EDGE('',*,*,#10481,.F.);
#14668=ORIENTED_EDGE('',*,*,#10478,.T.);
#14669=ORIENTED_EDGE('',*,*,#10483,.T.);
#14670=ORIENTED_EDGE('',*,*,#10484,.F.);
#14671=ORIENTED_EDGE('',*,*,#10483,.F.);
#14672=ORIENTED_EDGE('',*,*,#10477,.F.);
#14673=ORIENTED_EDGE('',*,*,#10485,.F.);
#14674=ORIENTED_EDGE('',*,*,#10486,.T.);
#14675=ORIENTED_EDGE('',*,*,#10487,.F.);
#14676=ORIENTED_EDGE('',*,*,#10488,.F.);
#14677=ORIENTED_EDGE('',*,*,#10489,.F.);
#14678=ORIENTED_EDGE('',*,*,#10488,.T.);
#14679=ORIENTED_EDGE('',*,*,#10490,.T.);
#14680=ORIENTED_EDGE('',*,*,#10491,.F.);
#14681=ORIENTED_EDGE('',*,*,#10490,.F.);
#14682=ORIENTED_EDGE('',*,*,#10487,.T.);
#14683=ORIENTED_EDGE('',*,*,#10492,.T.);
#14684=ORIENTED_EDGE('',*,*,#10493,.F.);
#14685=ORIENTED_EDGE('',*,*,#10492,.F.);
#14686=ORIENTED_EDGE('',*,*,#10486,.F.);
#14687=ORIENTED_EDGE('',*,*,#10494,.F.);
#14688=ORIENTED_EDGE('',*,*,#10495,.T.);
#14689=ORIENTED_EDGE('',*,*,#10496,.F.);
#14690=ORIENTED_EDGE('',*,*,#10497,.F.);
#14691=ORIENTED_EDGE('',*,*,#10498,.F.);
#14692=ORIENTED_EDGE('',*,*,#10497,.T.);
#14693=ORIENTED_EDGE('',*,*,#10499,.T.);
#14694=ORIENTED_EDGE('',*,*,#10500,.F.);
#14695=ORIENTED_EDGE('',*,*,#10499,.F.);
#14696=ORIENTED_EDGE('',*,*,#10496,.T.);
#14697=ORIENTED_EDGE('',*,*,#10501,.T.);
#14698=ORIENTED_EDGE('',*,*,#10502,.F.);
#14699=ORIENTED_EDGE('',*,*,#10501,.F.);
#14700=ORIENTED_EDGE('',*,*,#10495,.F.);
#14701=ORIENTED_EDGE('',*,*,#10503,.F.);
#14702=ORIENTED_EDGE('',*,*,#10504,.T.);
#14703=ORIENTED_EDGE('',*,*,#10505,.F.);
#14704=ORIENTED_EDGE('',*,*,#10506,.F.);
#14705=ORIENTED_EDGE('',*,*,#10507,.F.);
#14706=ORIENTED_EDGE('',*,*,#10506,.T.);
#14707=ORIENTED_EDGE('',*,*,#10508,.T.);
#14708=ORIENTED_EDGE('',*,*,#10509,.F.);
#14709=ORIENTED_EDGE('',*,*,#10508,.F.);
#14710=ORIENTED_EDGE('',*,*,#10505,.T.);
#14711=ORIENTED_EDGE('',*,*,#10510,.T.);
#14712=ORIENTED_EDGE('',*,*,#10511,.F.);
#14713=ORIENTED_EDGE('',*,*,#10510,.F.);
#14714=ORIENTED_EDGE('',*,*,#10504,.F.);
#14715=ORIENTED_EDGE('',*,*,#10512,.F.);
#14716=ORIENTED_EDGE('',*,*,#10513,.F.);
#14717=ORIENTED_EDGE('',*,*,#10514,.T.);
#14718=ORIENTED_EDGE('',*,*,#10512,.T.);
#14719=ORIENTED_EDGE('',*,*,#10514,.F.);
#14720=ORIENTED_EDGE('',*,*,#10069,.F.);
#14721=ORIENTED_EDGE('',*,*,#9990,.F.);
#14722=ORIENTED_EDGE('',*,*,#10070,.F.);
#14723=ORIENTED_EDGE('',*,*,#10515,.T.);
#14724=ORIENTED_EDGE('',*,*,#10513,.T.);
#14725=ORIENTED_EDGE('',*,*,#10515,.F.);
#14726=ORIENTED_EDGE('',*,*,#10025,.T.);
#14727=ORIENTED_EDGE('',*,*,#10066,.T.);
#14728=ORIENTED_EDGE('',*,*,#10076,.F.);
#14729=ORIENTED_EDGE('',*,*,#10075,.T.);
#14730=ORIENTED_EDGE('',*,*,#10516,.F.);
#14731=ORIENTED_EDGE('',*,*,#10517,.T.);
#14732=ORIENTED_EDGE('',*,*,#10077,.T.);
#14733=ORIENTED_EDGE('',*,*,#10517,.F.);
#14734=ORIENTED_EDGE('',*,*,#10518,.F.);
#14735=ORIENTED_EDGE('',*,*,#10516,.T.);
#14736=ORIENTED_EDGE('',*,*,#10519,.F.);
#14737=ORIENTED_EDGE('',*,*,#10520,.T.);
#14738=ORIENTED_EDGE('',*,*,#10518,.T.);
#14739=ORIENTED_EDGE('',*,*,#10520,.F.);
#14740=ORIENTED_EDGE('',*,*,#10521,.F.);
#14741=ORIENTED_EDGE('',*,*,#10522,.T.);
#14742=ORIENTED_EDGE('',*,*,#10376,.T.);
#14743=ORIENTED_EDGE('',*,*,#10366,.T.);
#14744=ORIENTED_EDGE('',*,*,#10370,.T.);
#14745=ORIENTED_EDGE('',*,*,#10523,.T.);
#14746=ORIENTED_EDGE('',*,*,#10519,.T.);
#14747=ORIENTED_EDGE('',*,*,#10523,.F.);
#14748=ORIENTED_EDGE('',*,*,#10372,.T.);
#14749=ORIENTED_EDGE('',*,*,#10373,.T.);
#14750=ORIENTED_EDGE('',*,*,#10375,.T.);
#14751=ORIENTED_EDGE('',*,*,#10522,.F.);
#14752=ORIENTED_EDGE('',*,*,#10246,.T.);
#14753=ORIENTED_EDGE('',*,*,#10248,.T.);
#14754=ORIENTED_EDGE('',*,*,#10240,.T.);
#14755=ORIENTED_EDGE('',*,*,#10244,.T.);
#14756=ORIENTED_EDGE('',*,*,#10255,.T.);
#14757=ORIENTED_EDGE('',*,*,#10257,.T.);
#14758=ORIENTED_EDGE('',*,*,#10249,.T.);
#14759=ORIENTED_EDGE('',*,*,#10253,.T.);
#14760=ORIENTED_EDGE('',*,*,#10264,.T.);
#14761=ORIENTED_EDGE('',*,*,#10266,.T.);
#14762=ORIENTED_EDGE('',*,*,#10258,.T.);
#14763=ORIENTED_EDGE('',*,*,#10262,.T.);
#14764=ORIENTED_EDGE('',*,*,#10273,.T.);
#14765=ORIENTED_EDGE('',*,*,#10275,.T.);
#14766=ORIENTED_EDGE('',*,*,#10267,.T.);
#14767=ORIENTED_EDGE('',*,*,#10271,.T.);
#14768=ORIENTED_EDGE('',*,*,#10282,.T.);
#14769=ORIENTED_EDGE('',*,*,#10284,.T.);
#14770=ORIENTED_EDGE('',*,*,#10276,.T.);
#14771=ORIENTED_EDGE('',*,*,#10280,.T.);
#14772=ORIENTED_EDGE('',*,*,#10291,.T.);
#14773=ORIENTED_EDGE('',*,*,#10293,.T.);
#14774=ORIENTED_EDGE('',*,*,#10285,.T.);
#14775=ORIENTED_EDGE('',*,*,#10289,.T.);
#14776=ORIENTED_EDGE('',*,*,#10300,.T.);
#14777=ORIENTED_EDGE('',*,*,#10302,.T.);
#14778=ORIENTED_EDGE('',*,*,#10294,.T.);
#14779=ORIENTED_EDGE('',*,*,#10298,.T.);
#14780=ORIENTED_EDGE('',*,*,#10309,.T.);
#14781=ORIENTED_EDGE('',*,*,#10311,.T.);
#14782=ORIENTED_EDGE('',*,*,#10303,.T.);
#14783=ORIENTED_EDGE('',*,*,#10307,.T.);
#14784=ORIENTED_EDGE('',*,*,#10318,.T.);
#14785=ORIENTED_EDGE('',*,*,#10320,.T.);
#14786=ORIENTED_EDGE('',*,*,#10312,.T.);
#14787=ORIENTED_EDGE('',*,*,#10316,.T.);
#14788=ORIENTED_EDGE('',*,*,#10327,.T.);
#14789=ORIENTED_EDGE('',*,*,#10329,.T.);
#14790=ORIENTED_EDGE('',*,*,#10321,.T.);
#14791=ORIENTED_EDGE('',*,*,#10325,.T.);
#14792=ORIENTED_EDGE('',*,*,#10336,.T.);
#14793=ORIENTED_EDGE('',*,*,#10338,.T.);
#14794=ORIENTED_EDGE('',*,*,#10330,.T.);
#14795=ORIENTED_EDGE('',*,*,#10334,.T.);
#14796=ORIENTED_EDGE('',*,*,#10345,.T.);
#14797=ORIENTED_EDGE('',*,*,#10347,.T.);
#14798=ORIENTED_EDGE('',*,*,#10339,.T.);
#14799=ORIENTED_EDGE('',*,*,#10343,.T.);
#14800=ORIENTED_EDGE('',*,*,#10354,.T.);
#14801=ORIENTED_EDGE('',*,*,#10356,.T.);
#14802=ORIENTED_EDGE('',*,*,#10348,.T.);
#14803=ORIENTED_EDGE('',*,*,#10352,.T.);
#14804=ORIENTED_EDGE('',*,*,#10363,.T.);
#14805=ORIENTED_EDGE('',*,*,#10365,.T.);
#14806=ORIENTED_EDGE('',*,*,#10357,.T.);
#14807=ORIENTED_EDGE('',*,*,#10361,.T.);
#14808=ORIENTED_EDGE('',*,*,#10383,.T.);
#14809=ORIENTED_EDGE('',*,*,#10385,.T.);
#14810=ORIENTED_EDGE('',*,*,#10377,.T.);
#14811=ORIENTED_EDGE('',*,*,#10381,.T.);
#14812=ORIENTED_EDGE('',*,*,#10392,.T.);
#14813=ORIENTED_EDGE('',*,*,#10394,.T.);
#14814=ORIENTED_EDGE('',*,*,#10386,.T.);
#14815=ORIENTED_EDGE('',*,*,#10390,.T.);
#14816=ORIENTED_EDGE('',*,*,#10401,.T.);
#14817=ORIENTED_EDGE('',*,*,#10403,.T.);
#14818=ORIENTED_EDGE('',*,*,#10395,.T.);
#14819=ORIENTED_EDGE('',*,*,#10399,.T.);
#14820=ORIENTED_EDGE('',*,*,#10410,.T.);
#14821=ORIENTED_EDGE('',*,*,#10412,.T.);
#14822=ORIENTED_EDGE('',*,*,#10404,.T.);
#14823=ORIENTED_EDGE('',*,*,#10408,.T.);
#14824=ORIENTED_EDGE('',*,*,#10419,.T.);
#14825=ORIENTED_EDGE('',*,*,#10421,.T.);
#14826=ORIENTED_EDGE('',*,*,#10413,.T.);
#14827=ORIENTED_EDGE('',*,*,#10417,.T.);
#14828=ORIENTED_EDGE('',*,*,#10428,.T.);
#14829=ORIENTED_EDGE('',*,*,#10430,.T.);
#14830=ORIENTED_EDGE('',*,*,#10422,.T.);
#14831=ORIENTED_EDGE('',*,*,#10426,.T.);
#14832=ORIENTED_EDGE('',*,*,#10437,.T.);
#14833=ORIENTED_EDGE('',*,*,#10439,.T.);
#14834=ORIENTED_EDGE('',*,*,#10431,.T.);
#14835=ORIENTED_EDGE('',*,*,#10435,.T.);
#14836=ORIENTED_EDGE('',*,*,#10446,.T.);
#14837=ORIENTED_EDGE('',*,*,#10448,.T.);
#14838=ORIENTED_EDGE('',*,*,#10440,.T.);
#14839=ORIENTED_EDGE('',*,*,#10444,.T.);
#14840=ORIENTED_EDGE('',*,*,#10455,.T.);
#14841=ORIENTED_EDGE('',*,*,#10457,.T.);
#14842=ORIENTED_EDGE('',*,*,#10449,.T.);
#14843=ORIENTED_EDGE('',*,*,#10453,.T.);
#14844=ORIENTED_EDGE('',*,*,#10464,.T.);
#14845=ORIENTED_EDGE('',*,*,#10466,.T.);
#14846=ORIENTED_EDGE('',*,*,#10458,.T.);
#14847=ORIENTED_EDGE('',*,*,#10462,.T.);
#14848=ORIENTED_EDGE('',*,*,#10473,.T.);
#14849=ORIENTED_EDGE('',*,*,#10475,.T.);
#14850=ORIENTED_EDGE('',*,*,#10467,.T.);
#14851=ORIENTED_EDGE('',*,*,#10471,.T.);
#14852=ORIENTED_EDGE('',*,*,#10482,.T.);
#14853=ORIENTED_EDGE('',*,*,#10484,.T.);
#14854=ORIENTED_EDGE('',*,*,#10476,.T.);
#14855=ORIENTED_EDGE('',*,*,#10480,.T.);
#14856=ORIENTED_EDGE('',*,*,#10491,.T.);
#14857=ORIENTED_EDGE('',*,*,#10493,.T.);
#14858=ORIENTED_EDGE('',*,*,#10485,.T.);
#14859=ORIENTED_EDGE('',*,*,#10489,.T.);
#14860=ORIENTED_EDGE('',*,*,#10500,.T.);
#14861=ORIENTED_EDGE('',*,*,#10502,.T.);
#14862=ORIENTED_EDGE('',*,*,#10494,.T.);
#14863=ORIENTED_EDGE('',*,*,#10498,.T.);
#14864=ORIENTED_EDGE('',*,*,#10509,.T.);
#14865=ORIENTED_EDGE('',*,*,#10511,.T.);
#14866=ORIENTED_EDGE('',*,*,#10503,.T.);
#14867=ORIENTED_EDGE('',*,*,#10507,.T.);
#14868=ORIENTED_EDGE('',*,*,#10524,.F.);
#14869=ORIENTED_EDGE('',*,*,#10525,.T.);
#14870=ORIENTED_EDGE('',*,*,#10521,.T.);
#14871=ORIENTED_EDGE('',*,*,#10525,.F.);
#14872=ORIENTED_EDGE('',*,*,#10524,.T.);
#14873=ORIENTED_EDGE('',*,*,#10078,.T.);
#14874=ORIENTED_EDGE('',*,*,#10109,.T.);
#14875=ORIENTED_EDGE('',*,*,#10106,.T.);
#14876=ORIENTED_EDGE('',*,*,#10103,.T.);
#14877=ORIENTED_EDGE('',*,*,#10100,.T.);
#14878=ORIENTED_EDGE('',*,*,#10097,.T.);
#14879=ORIENTED_EDGE('',*,*,#10094,.T.);
#14880=ORIENTED_EDGE('',*,*,#10091,.T.);
#14881=ORIENTED_EDGE('',*,*,#10088,.T.);
#14882=ORIENTED_EDGE('',*,*,#10085,.T.);
#14883=ORIENTED_EDGE('',*,*,#10082,.T.);
#14884=ORIENTED_EDGE('',*,*,#10111,.T.);
#14885=ORIENTED_EDGE('',*,*,#10139,.T.);
#14886=ORIENTED_EDGE('',*,*,#10136,.T.);
#14887=ORIENTED_EDGE('',*,*,#10133,.T.);
#14888=ORIENTED_EDGE('',*,*,#10130,.T.);
#14889=ORIENTED_EDGE('',*,*,#10127,.T.);
#14890=ORIENTED_EDGE('',*,*,#10124,.T.);
#14891=ORIENTED_EDGE('',*,*,#10121,.T.);
#14892=ORIENTED_EDGE('',*,*,#10118,.T.);
#14893=ORIENTED_EDGE('',*,*,#10115,.T.);
#14894=ORIENTED_EDGE('',*,*,#10141,.T.);
#14895=ORIENTED_EDGE('',*,*,#10172,.T.);
#14896=ORIENTED_EDGE('',*,*,#10169,.T.);
#14897=ORIENTED_EDGE('',*,*,#10166,.T.);
#14898=ORIENTED_EDGE('',*,*,#10163,.T.);
#14899=ORIENTED_EDGE('',*,*,#10160,.T.);
#14900=ORIENTED_EDGE('',*,*,#10157,.T.);
#14901=ORIENTED_EDGE('',*,*,#10154,.T.);
#14902=ORIENTED_EDGE('',*,*,#10151,.T.);
#14903=ORIENTED_EDGE('',*,*,#10148,.T.);
#14904=ORIENTED_EDGE('',*,*,#10145,.T.);
#14905=ORIENTED_EDGE('',*,*,#10174,.T.);
#14906=ORIENTED_EDGE('',*,*,#10202,.T.);
#14907=ORIENTED_EDGE('',*,*,#10199,.T.);
#14908=ORIENTED_EDGE('',*,*,#10196,.T.);
#14909=ORIENTED_EDGE('',*,*,#10193,.T.);
#14910=ORIENTED_EDGE('',*,*,#10190,.T.);
#14911=ORIENTED_EDGE('',*,*,#10187,.T.);
#14912=ORIENTED_EDGE('',*,*,#10184,.T.);
#14913=ORIENTED_EDGE('',*,*,#10181,.T.);
#14914=ORIENTED_EDGE('',*,*,#10178,.T.);
#14915=ORIENTED_EDGE('',*,*,#10204,.T.);
#14916=ORIENTED_EDGE('',*,*,#10232,.T.);
#14917=ORIENTED_EDGE('',*,*,#10229,.T.);
#14918=ORIENTED_EDGE('',*,*,#10226,.T.);
#14919=ORIENTED_EDGE('',*,*,#10223,.T.);
#14920=ORIENTED_EDGE('',*,*,#10220,.T.);
#14921=ORIENTED_EDGE('',*,*,#10217,.T.);
#14922=ORIENTED_EDGE('',*,*,#10214,.T.);
#14923=ORIENTED_EDGE('',*,*,#10211,.T.);
#14924=ORIENTED_EDGE('',*,*,#10208,.T.);
#14925=ORIENTED_EDGE('',*,*,#10237,.T.);
#15521=CONICAL_SURFACE('',#17864,3.,0.982793723247329);
#15522=CONICAL_SURFACE('',#17866,4.75,0.785398163397448);
#15523=CONICAL_SURFACE('',#17872,12.7,0.785398163397447);
#15524=CONICAL_SURFACE('',#17876,12.7,0.785398163397448);
#16167=ADVANCED_FACE('',(#2439),#1752,.T.);
#16168=ADVANCED_FACE('',(#2440),#1753,.T.);
#16169=ADVANCED_FACE('',(#2441),#1754,.T.);
#16170=ADVANCED_FACE('',(#2442),#1755,.T.);
#16171=ADVANCED_FACE('',(#2443),#1756,.T.);
#16172=ADVANCED_FACE('',(#2444),#1757,.T.);
#16173=ADVANCED_FACE('',(#2445),#1758,.T.);
#16174=ADVANCED_FACE('',(#2446),#1759,.T.);
#16175=ADVANCED_FACE('',(#2447),#1760,.T.);
#16176=ADVANCED_FACE('',(#2448),#1761,.T.);
#16177=ADVANCED_FACE('',(#2449),#1762,.T.);
#16178=ADVANCED_FACE('',(#2450),#1763,.T.);
#16179=ADVANCED_FACE('',(#2451),#1764,.T.);
#16180=ADVANCED_FACE('',(#2452),#1765,.T.);
#16181=ADVANCED_FACE('',(#2453),#1766,.T.);
#16182=ADVANCED_FACE('',(#2454),#1767,.T.);
#16183=ADVANCED_FACE('',(#2455),#1768,.T.);
#16184=ADVANCED_FACE('',(#2456),#1769,.T.);
#16185=ADVANCED_FACE('',(#2457),#1770,.T.);
#16186=ADVANCED_FACE('',(#2458),#1771,.T.);
#16187=ADVANCED_FACE('',(#2459),#1772,.T.);
#16188=ADVANCED_FACE('',(#2460),#1773,.T.);
#16189=ADVANCED_FACE('',(#2461),#1774,.T.);
#16190=ADVANCED_FACE('',(#2462),#1775,.T.);
#16191=ADVANCED_FACE('',(#2463),#1776,.T.);
#16192=ADVANCED_FACE('',(#2464),#907,.F.);
#16193=ADVANCED_FACE('',(#2465),#1336,.T.);
#16194=ADVANCED_FACE('',(#2466),#1777,.T.);
#16195=ADVANCED_FACE('',(#2467),#908,.F.);
#16196=ADVANCED_FACE('',(#2468,#1004),#1337,.T.);
#16197=ADVANCED_FACE('',(#2469),#909,.F.);
#16198=ADVANCED_FACE('',(#2470),#910,.F.);
#16199=ADVANCED_FACE('',(#2471),#911,.F.);
#16200=ADVANCED_FACE('',(#2472),#912,.F.);
#16201=ADVANCED_FACE('',(#2473),#913,.F.);
#16202=ADVANCED_FACE('',(#2474),#914,.F.);
#16203=ADVANCED_FACE('',(#2475),#915,.F.);
#16204=ADVANCED_FACE('',(#2476),#916,.F.);
#16205=ADVANCED_FACE('',(#2477),#917,.F.);
#16206=ADVANCED_FACE('',(#2478),#918,.F.);
#16207=ADVANCED_FACE('',(#2479),#919,.F.);
#16208=ADVANCED_FACE('',(#2480),#1338,.T.);
#16209=ADVANCED_FACE('',(#2481),#1339,.F.);
#16210=ADVANCED_FACE('',(#2482),#1340,.F.);
#16211=ADVANCED_FACE('',(#2483),#1341,.F.);
#16212=ADVANCED_FACE('',(#2484),#1342,.F.);
#16213=ADVANCED_FACE('',(#2485),#1343,.F.);
#16214=ADVANCED_FACE('',(#2486),#1344,.F.);
#16215=ADVANCED_FACE('',(#2487),#1345,.F.);
#16216=ADVANCED_FACE('',(#2488),#1346,.F.);
#16217=ADVANCED_FACE('',(#2489),#1347,.F.);
#16218=ADVANCED_FACE('',(#2490),#1348,.F.);
#16219=ADVANCED_FACE('',(#2491),#1349,.F.);
#16220=ADVANCED_FACE('',(#2492),#920,.F.);
#16221=ADVANCED_FACE('',(#2493),#921,.F.);
#16222=ADVANCED_FACE('',(#2494),#922,.F.);
#16223=ADVANCED_FACE('',(#2495),#923,.F.);
#16224=ADVANCED_FACE('',(#2496),#924,.F.);
#16225=ADVANCED_FACE('',(#2497),#925,.F.);
#16226=ADVANCED_FACE('',(#2498),#926,.F.);
#16227=ADVANCED_FACE('',(#2499),#927,.F.);
#16228=ADVANCED_FACE('',(#2500),#928,.F.);
#16229=ADVANCED_FACE('',(#2501),#929,.F.);
#16230=ADVANCED_FACE('',(#2502),#930,.F.);
#16231=ADVANCED_FACE('',(#2503),#1350,.T.);
#16232=ADVANCED_FACE('',(#2504),#1351,.F.);
#16233=ADVANCED_FACE('',(#2505),#1352,.F.);
#16234=ADVANCED_FACE('',(#2506),#1353,.F.);
#16235=ADVANCED_FACE('',(#2507),#1354,.F.);
#16236=ADVANCED_FACE('',(#2508),#1355,.F.);
#16237=ADVANCED_FACE('',(#2509),#1356,.F.);
#16238=ADVANCED_FACE('',(#2510),#1357,.F.);
#16239=ADVANCED_FACE('',(#2511),#1358,.F.);
#16240=ADVANCED_FACE('',(#2512),#1359,.F.);
#16241=ADVANCED_FACE('',(#2513),#1360,.F.);
#16242=ADVANCED_FACE('',(#2514),#1361,.F.);
#16243=ADVANCED_FACE('',(#2515),#1362,.F.);
#16244=ADVANCED_FACE('',(#2516),#1363,.F.);
#16245=ADVANCED_FACE('',(#2517),#1364,.F.);
#16246=ADVANCED_FACE('',(#2518),#1365,.F.);
#16247=ADVANCED_FACE('',(#2519),#1366,.F.);
#16248=ADVANCED_FACE('',(#2520),#1367,.F.);
#16249=ADVANCED_FACE('',(#2521),#1368,.F.);
#16250=ADVANCED_FACE('',(#2522),#1369,.F.);
#16251=ADVANCED_FACE('',(#2523),#1370,.F.);
#16252=ADVANCED_FACE('',(#2524),#1371,.F.);
#16253=ADVANCED_FACE('',(#2525),#1372,.F.);
#16254=ADVANCED_FACE('',(#2526,#1005),#1373,.F.);
#16255=ADVANCED_FACE('',(#2527),#1778,.F.);
#16256=ADVANCED_FACE('',(#2528),#1779,.T.);
#16257=ADVANCED_FACE('',(#2529),#1374,.T.);
#16258=ADVANCED_FACE('',(#2530),#1375,.F.);
#16259=ADVANCED_FACE('',(#2531),#1376,.T.);
#16260=ADVANCED_FACE('',(#2532),#1377,.F.);
#16261=ADVANCED_FACE('',(#2533),#1378,.F.);
#16262=ADVANCED_FACE('',(#2534),#1379,.F.);
#16263=ADVANCED_FACE('',(#2535),#1380,.T.);
#16264=ADVANCED_FACE('',(#2536),#1381,.F.);
#16265=ADVANCED_FACE('',(#2537),#1382,.F.);
#16266=ADVANCED_FACE('',(#2538),#1383,.F.);
#16267=ADVANCED_FACE('',(#2539),#1384,.T.);
#16268=ADVANCED_FACE('',(#2540),#1385,.F.);
#16269=ADVANCED_FACE('',(#2541),#1386,.F.);
#16270=ADVANCED_FACE('',(#2542),#1387,.F.);
#16271=ADVANCED_FACE('',(#2543),#1388,.T.);
#16272=ADVANCED_FACE('',(#2544),#1389,.F.);
#16273=ADVANCED_FACE('',(#2545),#1390,.F.);
#16274=ADVANCED_FACE('',(#2546),#1391,.F.);
#16275=ADVANCED_FACE('',(#2547),#1392,.T.);
#16276=ADVANCED_FACE('',(#2548),#1393,.F.);
#16277=ADVANCED_FACE('',(#2549),#1394,.F.);
#16278=ADVANCED_FACE('',(#2550),#1395,.F.);
#16279=ADVANCED_FACE('',(#2551),#1396,.T.);
#16280=ADVANCED_FACE('',(#2552),#1397,.F.);
#16281=ADVANCED_FACE('',(#2553),#1398,.F.);
#16282=ADVANCED_FACE('',(#2554),#1399,.F.);
#16283=ADVANCED_FACE('',(#2555),#1400,.T.);
#16284=ADVANCED_FACE('',(#2556),#1401,.F.);
#16285=ADVANCED_FACE('',(#2557),#1402,.F.);
#16286=ADVANCED_FACE('',(#2558),#1403,.F.);
#16287=ADVANCED_FACE('',(#2559),#1404,.T.);
#16288=ADVANCED_FACE('',(#2560),#1405,.F.);
#16289=ADVANCED_FACE('',(#2561),#1406,.F.);
#16290=ADVANCED_FACE('',(#2562),#1407,.F.);
#16291=ADVANCED_FACE('',(#2563),#1408,.T.);
#16292=ADVANCED_FACE('',(#2564),#1409,.F.);
#16293=ADVANCED_FACE('',(#2565),#1410,.F.);
#16294=ADVANCED_FACE('',(#2566),#1411,.F.);
#16295=ADVANCED_FACE('',(#2567),#1412,.T.);
#16296=ADVANCED_FACE('',(#2568),#1413,.F.);
#16297=ADVANCED_FACE('',(#2569),#1414,.F.);
#16298=ADVANCED_FACE('',(#2570),#1415,.F.);
#16299=ADVANCED_FACE('',(#2571),#1416,.T.);
#16300=ADVANCED_FACE('',(#2572),#1417,.F.);
#16301=ADVANCED_FACE('',(#2573),#1418,.F.);
#16302=ADVANCED_FACE('',(#2574),#1419,.F.);
#16303=ADVANCED_FACE('',(#2575),#1420,.T.);
#16304=ADVANCED_FACE('',(#2576),#1421,.F.);
#16305=ADVANCED_FACE('',(#2577),#1422,.F.);
#16306=ADVANCED_FACE('',(#2578),#1423,.F.);
#16307=ADVANCED_FACE('',(#2579),#1424,.T.);
#16308=ADVANCED_FACE('',(#2580),#1425,.F.);
#16309=ADVANCED_FACE('',(#2581),#1426,.F.);
#16310=ADVANCED_FACE('',(#2582),#1427,.F.);
#16311=ADVANCED_FACE('',(#2583),#1428,.T.);
#16312=ADVANCED_FACE('',(#2584),#1429,.F.);
#16313=ADVANCED_FACE('',(#2585),#1430,.F.);
#16314=ADVANCED_FACE('',(#2586),#1431,.F.);
#16315=ADVANCED_FACE('',(#2587),#1432,.T.);
#16316=ADVANCED_FACE('',(#2588),#1433,.F.);
#16317=ADVANCED_FACE('',(#2589),#1434,.F.);
#16318=ADVANCED_FACE('',(#2590),#1435,.F.);
#16319=ADVANCED_FACE('',(#2591),#1436,.T.);
#16320=ADVANCED_FACE('',(#2592),#1437,.F.);
#16321=ADVANCED_FACE('',(#2593),#1438,.F.);
#16322=ADVANCED_FACE('',(#2594),#1439,.F.);
#16323=ADVANCED_FACE('',(#2595),#1440,.T.);
#16324=ADVANCED_FACE('',(#2596),#1441,.F.);
#16325=ADVANCED_FACE('',(#2597),#1442,.F.);
#16326=ADVANCED_FACE('',(#2598),#1443,.F.);
#16327=ADVANCED_FACE('',(#2599),#1444,.T.);
#16328=ADVANCED_FACE('',(#2600),#1445,.F.);
#16329=ADVANCED_FACE('',(#2601),#1446,.F.);
#16330=ADVANCED_FACE('',(#2602),#1447,.F.);
#16331=ADVANCED_FACE('',(#2603),#1448,.T.);
#16332=ADVANCED_FACE('',(#2604),#1449,.F.);
#16333=ADVANCED_FACE('',(#2605),#1450,.F.);
#16334=ADVANCED_FACE('',(#2606),#1451,.F.);
#16335=ADVANCED_FACE('',(#2607),#1452,.T.);
#16336=ADVANCED_FACE('',(#2608),#1453,.F.);
#16337=ADVANCED_FACE('',(#2609),#1454,.F.);
#16338=ADVANCED_FACE('',(#2610),#1455,.F.);
#16339=ADVANCED_FACE('',(#2611),#1456,.T.);
#16340=ADVANCED_FACE('',(#2612),#1457,.F.);
#16341=ADVANCED_FACE('',(#2613),#1458,.F.);
#16342=ADVANCED_FACE('',(#2614),#1459,.F.);
#16343=ADVANCED_FACE('',(#2615),#1460,.T.);
#16344=ADVANCED_FACE('',(#2616),#1461,.F.);
#16345=ADVANCED_FACE('',(#2617),#1462,.F.);
#16346=ADVANCED_FACE('',(#2618),#1463,.F.);
#16347=ADVANCED_FACE('',(#2619),#1464,.T.);
#16348=ADVANCED_FACE('',(#2620),#1465,.F.);
#16349=ADVANCED_FACE('',(#2621),#1466,.F.);
#16350=ADVANCED_FACE('',(#2622),#1467,.F.);
#16351=ADVANCED_FACE('',(#2623),#1468,.T.);
#16352=ADVANCED_FACE('',(#2624),#1469,.F.);
#16353=ADVANCED_FACE('',(#2625),#1470,.F.);
#16354=ADVANCED_FACE('',(#2626),#1471,.F.);
#16355=ADVANCED_FACE('',(#2627),#1472,.T.);
#16356=ADVANCED_FACE('',(#2628),#1473,.F.);
#16357=ADVANCED_FACE('',(#2629),#1474,.F.);
#16358=ADVANCED_FACE('',(#2630),#1475,.F.);
#16359=ADVANCED_FACE('',(#2631),#1476,.T.);
#16360=ADVANCED_FACE('',(#2632),#1477,.F.);
#16361=ADVANCED_FACE('',(#2633),#1478,.F.);
#16362=ADVANCED_FACE('',(#2634),#1479,.F.);
#16363=ADVANCED_FACE('',(#2635),#1480,.T.);
#16364=ADVANCED_FACE('',(#2636),#1481,.F.);
#16365=ADVANCED_FACE('',(#2637),#1482,.F.);
#16366=ADVANCED_FACE('',(#2638),#1483,.F.);
#16367=ADVANCED_FACE('',(#2639),#1484,.T.);
#16368=ADVANCED_FACE('',(#2640),#1485,.F.);
#16369=ADVANCED_FACE('',(#2641),#1486,.F.);
#16370=ADVANCED_FACE('',(#2642),#1487,.F.);
#16371=ADVANCED_FACE('',(#2643),#1488,.T.);
#16372=ADVANCED_FACE('',(#2644),#1489,.F.);
#16373=ADVANCED_FACE('',(#2645),#1490,.F.);
#16374=ADVANCED_FACE('',(#2646),#1491,.F.);
#16375=ADVANCED_FACE('',(#2647),#1492,.T.);
#16376=ADVANCED_FACE('',(#2648),#1493,.F.);
#16377=ADVANCED_FACE('',(#2649),#1494,.F.);
#16378=ADVANCED_FACE('',(#2650),#1495,.T.);
#16379=ADVANCED_FACE('',(#2651),#15521,.T.);
#16380=ADVANCED_FACE('',(#2652),#15522,.T.);
#16381=ADVANCED_FACE('',(#2653),#1780,.T.);
#16382=ADVANCED_FACE('',(#2654),#1781,.T.);
#16383=ADVANCED_FACE('',(#2655,#1006),#1496,.T.);
#16384=ADVANCED_FACE('',(#2656),#15523,.T.);
#16385=ADVANCED_FACE('',(#2657,#1007,#1008,#1009,#1010,#1011,#1012,#1013,
#1014,#1015,#1016,#1017,#1018,#1019,#1020,#1021,#1022,#1023,#1024,#1025,
#1026,#1027,#1028,#1029,#1030,#1031,#1032,#1033,#1034,#1035),#1782,.T.);
#16386=ADVANCED_FACE('',(#2658),#15524,.T.);
#16387=ADVANCED_FACE('',(#2659,#1036,#1037,#1038,#1039,#1040,#1041),#1497,
 .T.);
#16530=CLOSED_SHELL('',(#16167,#16168,#16169,#16170,#16171,#16172,#16173,
#16174,#16175,#16176,#16177,#16178,#16179,#16180,#16181,#16182,#16183,#16184,
#16185,#16186,#16187,#16188,#16189,#16190,#16191,#16192,#16193,#16194,#16195,
#16196,#16197,#16198,#16199,#16200,#16201,#16202,#16203,#16204,#16205,#16206,
#16207,#16208,#16209,#16210,#16211,#16212,#16213,#16214,#16215,#16216,#16217,
#16218,#16219,#16220,#16221,#16222,#16223,#16224,#16225,#16226,#16227,#16228,
#16229,#16230,#16231,#16232,#16233,#16234,#16235,#16236,#16237,#16238,#16239,
#16240,#16241,#16242,#16243,#16244,#16245,#16246,#16247,#16248,#16249,#16250,
#16251,#16252,#16253,#16254,#16255,#16256,#16257,#16258,#16259,#16260,#16261,
#16262,#16263,#16264,#16265,#16266,#16267,#16268,#16269,#16270,#16271,#16272,
#16273,#16274,#16275,#16276,#16277,#16278,#16279,#16280,#16281,#16282,#16283,
#16284,#16285,#16286,#16287,#16288,#16289,#16290,#16291,#16292,#16293,#16294,
#16295,#16296,#16297,#16298,#16299,#16300,#16301,#16302,#16303,#16304,#16305,
#16306,#16307,#16308,#16309,#16310,#16311,#16312,#16313,#16314,#16315,#16316,
#16317,#16318,#16319,#16320,#16321,#16322,#16323,#16324,#16325,#16326,#16327,
#16328,#16329,#16330,#16331,#16332,#16333,#16334,#16335,#16336,#16337,#16338,
#16339,#16340,#16341,#16342,#16343,#16344,#16345,#16346,#16347,#16348,#16349,
#16350,#16351,#16352,#16353,#16354,#16355,#16356,#16357,#16358,#16359,#16360,
#16361,#16362,#16363,#16364,#16365,#16366,#16367,#16368,#16369,#16370,#16371,
#16372,#16373,#16374,#16375,#16376,#16377,#16378,#16379,#16380,#16381,#16382,
#16383,#16384,#16385,#16386,#16387));
#17601=AXIS2_PLACEMENT_3D('',#40639,#20599,#20600);
#17602=AXIS2_PLACEMENT_3D('',#40640,#20601,#20602);
#17603=AXIS2_PLACEMENT_3D('',#40656,#20604,#20605);
#17604=AXIS2_PLACEMENT_3D('',#40667,#20606,#20607);
#17605=AXIS2_PLACEMENT_3D('',#40715,#20609,#20610);
#17606=AXIS2_PLACEMENT_3D('',#40763,#20612,#20613);
#17607=AXIS2_PLACEMENT_3D('',#40811,#20615,#20616);
#17608=AXIS2_PLACEMENT_3D('',#40865,#20618,#20619);
#17609=AXIS2_PLACEMENT_3D('',#40913,#20621,#20622);
#17610=AXIS2_PLACEMENT_3D('',#40961,#20624,#20625);
#17611=AXIS2_PLACEMENT_3D('',#41015,#20627,#20628);
#17612=AXIS2_PLACEMENT_3D('',#41063,#20630,#20631);
#17613=AXIS2_PLACEMENT_3D('',#41111,#20633,#20634);
#17614=AXIS2_PLACEMENT_3D('',#41159,#20636,#20637);
#17615=AXIS2_PLACEMENT_3D('',#41213,#20639,#20640);
#17616=AXIS2_PLACEMENT_3D('',#41261,#20642,#20643);
#17617=AXIS2_PLACEMENT_3D('',#41276,#20645,#20646);
#17618=AXIS2_PLACEMENT_3D('',#41286,#20647,#20648);
#17619=AXIS2_PLACEMENT_3D('',#41311,#20650,#20651);
#17620=AXIS2_PLACEMENT_3D('',#41336,#20653,#20654);
#17621=AXIS2_PLACEMENT_3D('',#41360,#20656,#20657);
#17622=AXIS2_PLACEMENT_3D('',#41384,#20659,#20660);
#17623=AXIS2_PLACEMENT_3D('',#41409,#20662,#20663);
#17624=AXIS2_PLACEMENT_3D('',#41434,#20665,#20666);
#17625=AXIS2_PLACEMENT_3D('',#41458,#20668,#20669);
#17626=AXIS2_PLACEMENT_3D('',#41483,#20671,#20672);
#17627=AXIS2_PLACEMENT_3D('',#41508,#20674,#20675);
#17628=AXIS2_PLACEMENT_3D('',#41532,#20677,#20678);
#17629=AXIS2_PLACEMENT_3D('',#42133,#20680,#20681);
#17630=AXIS2_PLACEMENT_3D('',#42135,#20682,#20683);
#17631=AXIS2_PLACEMENT_3D('',#42136,#20684,#20685);
#17632=AXIS2_PLACEMENT_3D('',#42250,#20686,#20687);
#17633=AXIS2_PLACEMENT_3D('',#42251,#20688,#20689);
#17634=AXIS2_PLACEMENT_3D('',#42725,#20690,#20691);
#17635=AXIS2_PLACEMENT_3D('',#42726,#20692,#20693);
#17636=AXIS2_PLACEMENT_3D('',#42728,#20694,#20695);
#17637=AXIS2_PLACEMENT_3D('',#42894,#20707,#20708);
#17638=AXIS2_PLACEMENT_3D('',#42895,#20709,#20710);
#17639=AXIS2_PLACEMENT_3D('',#42904,#20715,#20716);
#17640=AXIS2_PLACEMENT_3D('',#42910,#20720,#20721);
#17641=AXIS2_PLACEMENT_3D('',#42916,#20725,#20726);
#17642=AXIS2_PLACEMENT_3D('',#42922,#20730,#20731);
#17643=AXIS2_PLACEMENT_3D('',#42928,#20735,#20736);
#17644=AXIS2_PLACEMENT_3D('',#42934,#20740,#20741);
#17645=AXIS2_PLACEMENT_3D('',#42940,#20745,#20746);
#17646=AXIS2_PLACEMENT_3D('',#42946,#20750,#20751);
#17647=AXIS2_PLACEMENT_3D('',#42952,#20755,#20756);
#17648=AXIS2_PLACEMENT_3D('',#42955,#20759,#20760);
#17649=AXIS2_PLACEMENT_3D('',#43121,#20772,#20773);
#17650=AXIS2_PLACEMENT_3D('',#43122,#20774,#20775);
#17651=AXIS2_PLACEMENT_3D('',#43131,#20780,#20781);
#17652=AXIS2_PLACEMENT_3D('',#43137,#20785,#20786);
#17653=AXIS2_PLACEMENT_3D('',#43143,#20790,#20791);
#17654=AXIS2_PLACEMENT_3D('',#43149,#20795,#20796);
#17655=AXIS2_PLACEMENT_3D('',#43155,#20800,#20801);
#17656=AXIS2_PLACEMENT_3D('',#43161,#20805,#20806);
#17657=AXIS2_PLACEMENT_3D('',#43167,#20810,#20811);
#17658=AXIS2_PLACEMENT_3D('',#43173,#20815,#20816);
#17659=AXIS2_PLACEMENT_3D('',#43179,#20820,#20821);
#17660=AXIS2_PLACEMENT_3D('',#43182,#20824,#20825);
#17661=AXIS2_PLACEMENT_3D('',#43183,#20826,#20827);
#17662=AXIS2_PLACEMENT_3D('',#43192,#20832,#20833);
#17663=AXIS2_PLACEMENT_3D('',#43198,#20837,#20838);
#17664=AXIS2_PLACEMENT_3D('',#43204,#20842,#20843);
#17665=AXIS2_PLACEMENT_3D('',#43210,#20847,#20848);
#17666=AXIS2_PLACEMENT_3D('',#43216,#20852,#20853);
#17667=AXIS2_PLACEMENT_3D('',#43222,#20857,#20858);
#17668=AXIS2_PLACEMENT_3D('',#43228,#20862,#20863);
#17669=AXIS2_PLACEMENT_3D('',#43234,#20867,#20868);
#17670=AXIS2_PLACEMENT_3D('',#43240,#20872,#20873);
#17671=AXIS2_PLACEMENT_3D('',#43243,#20876,#20877);
#17672=AXIS2_PLACEMENT_3D('',#43244,#20878,#20879);
#17673=AXIS2_PLACEMENT_3D('',#43246,#20880,#20881);
#17674=AXIS2_PLACEMENT_3D('',#43248,#20882,#20883);
#17675=AXIS2_PLACEMENT_3D('',#43249,#20884,#20885);
#17676=AXIS2_PLACEMENT_3D('',#43252,#20887,#20888);
#17677=AXIS2_PLACEMENT_3D('',#43253,#20889,#20890);
#17678=AXIS2_PLACEMENT_3D('',#43256,#20892,#20893);
#17679=AXIS2_PLACEMENT_3D('',#43257,#20894,#20895);
#17680=AXIS2_PLACEMENT_3D('',#43258,#20896,#20897);
#17681=AXIS2_PLACEMENT_3D('',#43267,#20902,#20903);
#17682=AXIS2_PLACEMENT_3D('',#43269,#20904,#20905);
#17683=AXIS2_PLACEMENT_3D('',#43271,#20907,#20908);
#17684=AXIS2_PLACEMENT_3D('',#43275,#20911,#20912);
#17685=AXIS2_PLACEMENT_3D('',#43276,#20913,#20914);
#17686=AXIS2_PLACEMENT_3D('',#43277,#20915,#20916);
#17687=AXIS2_PLACEMENT_3D('',#43286,#20921,#20922);
#17688=AXIS2_PLACEMENT_3D('',#43288,#20923,#20924);
#17689=AXIS2_PLACEMENT_3D('',#43290,#20926,#20927);
#17690=AXIS2_PLACEMENT_3D('',#43294,#20930,#20931);
#17691=AXIS2_PLACEMENT_3D('',#43295,#20932,#20933);
#17692=AXIS2_PLACEMENT_3D('',#43296,#20934,#20935);
#17693=AXIS2_PLACEMENT_3D('',#43305,#20940,#20941);
#17694=AXIS2_PLACEMENT_3D('',#43307,#20942,#20943);
#17695=AXIS2_PLACEMENT_3D('',#43309,#20945,#20946);
#17696=AXIS2_PLACEMENT_3D('',#43313,#20949,#20950);
#17697=AXIS2_PLACEMENT_3D('',#43314,#20951,#20952);
#17698=AXIS2_PLACEMENT_3D('',#43315,#20953,#20954);
#17699=AXIS2_PLACEMENT_3D('',#43324,#20959,#20960);
#17700=AXIS2_PLACEMENT_3D('',#43326,#20961,#20962);
#17701=AXIS2_PLACEMENT_3D('',#43328,#20964,#20965);
#17702=AXIS2_PLACEMENT_3D('',#43332,#20968,#20969);
#17703=AXIS2_PLACEMENT_3D('',#43333,#20970,#20971);
#17704=AXIS2_PLACEMENT_3D('',#43334,#20972,#20973);
#17705=AXIS2_PLACEMENT_3D('',#43343,#20978,#20979);
#17706=AXIS2_PLACEMENT_3D('',#43345,#20980,#20981);
#17707=AXIS2_PLACEMENT_3D('',#43347,#20983,#20984);
#17708=AXIS2_PLACEMENT_3D('',#43351,#20987,#20988);
#17709=AXIS2_PLACEMENT_3D('',#43352,#20989,#20990);
#17710=AXIS2_PLACEMENT_3D('',#43353,#20991,#20992);
#17711=AXIS2_PLACEMENT_3D('',#43362,#20997,#20998);
#17712=AXIS2_PLACEMENT_3D('',#43364,#20999,#21000);
#17713=AXIS2_PLACEMENT_3D('',#43366,#21002,#21003);
#17714=AXIS2_PLACEMENT_3D('',#43370,#21006,#21007);
#17715=AXIS2_PLACEMENT_3D('',#43371,#21008,#21009);
#17716=AXIS2_PLACEMENT_3D('',#43372,#21010,#21011);
#17717=AXIS2_PLACEMENT_3D('',#43381,#21016,#21017);
#17718=AXIS2_PLACEMENT_3D('',#43383,#21018,#21019);
#17719=AXIS2_PLACEMENT_3D('',#43385,#21021,#21022);
#17720=AXIS2_PLACEMENT_3D('',#43389,#21025,#21026);
#17721=AXIS2_PLACEMENT_3D('',#43390,#21027,#21028);
#17722=AXIS2_PLACEMENT_3D('',#43391,#21029,#21030);
#17723=AXIS2_PLACEMENT_3D('',#43400,#21035,#21036);
#17724=AXIS2_PLACEMENT_3D('',#43402,#21037,#21038);
#17725=AXIS2_PLACEMENT_3D('',#43404,#21040,#21041);
#17726=AXIS2_PLACEMENT_3D('',#43408,#21044,#21045);
#17727=AXIS2_PLACEMENT_3D('',#43409,#21046,#21047);
#17728=AXIS2_PLACEMENT_3D('',#43410,#21048,#21049);
#17729=AXIS2_PLACEMENT_3D('',#43419,#21054,#21055);
#17730=AXIS2_PLACEMENT_3D('',#43421,#21056,#21057);
#17731=AXIS2_PLACEMENT_3D('',#43423,#21059,#21060);
#17732=AXIS2_PLACEMENT_3D('',#43427,#21063,#21064);
#17733=AXIS2_PLACEMENT_3D('',#43428,#21065,#21066);
#17734=AXIS2_PLACEMENT_3D('',#43429,#21067,#21068);
#17735=AXIS2_PLACEMENT_3D('',#43438,#21073,#21074);
#17736=AXIS2_PLACEMENT_3D('',#43440,#21075,#21076);
#17737=AXIS2_PLACEMENT_3D('',#43442,#21078,#21079);
#17738=AXIS2_PLACEMENT_3D('',#43446,#21082,#21083);
#17739=AXIS2_PLACEMENT_3D('',#43447,#21084,#21085);
#17740=AXIS2_PLACEMENT_3D('',#43448,#21086,#21087);
#17741=AXIS2_PLACEMENT_3D('',#43457,#21092,#21093);
#17742=AXIS2_PLACEMENT_3D('',#43459,#21094,#21095);
#17743=AXIS2_PLACEMENT_3D('',#43461,#21097,#21098);
#17744=AXIS2_PLACEMENT_3D('',#43465,#21101,#21102);
#17745=AXIS2_PLACEMENT_3D('',#43466,#21103,#21104);
#17746=AXIS2_PLACEMENT_3D('',#43467,#21105,#21106);
#17747=AXIS2_PLACEMENT_3D('',#43476,#21111,#21112);
#17748=AXIS2_PLACEMENT_3D('',#43478,#21113,#21114);
#17749=AXIS2_PLACEMENT_3D('',#43480,#21116,#21117);
#17750=AXIS2_PLACEMENT_3D('',#43484,#21120,#21121);
#17751=AXIS2_PLACEMENT_3D('',#43485,#21122,#21123);
#17752=AXIS2_PLACEMENT_3D('',#43486,#21124,#21125);
#17753=AXIS2_PLACEMENT_3D('',#43495,#21130,#21131);
#17754=AXIS2_PLACEMENT_3D('',#43497,#21132,#21133);
#17755=AXIS2_PLACEMENT_3D('',#43499,#21135,#21136);
#17756=AXIS2_PLACEMENT_3D('',#43503,#21139,#21140);
#17757=AXIS2_PLACEMENT_3D('',#43504,#21141,#21142);
#17758=AXIS2_PLACEMENT_3D('',#43505,#21143,#21144);
#17759=AXIS2_PLACEMENT_3D('',#43514,#21149,#21150);
#17760=AXIS2_PLACEMENT_3D('',#43516,#21151,#21152);
#17761=AXIS2_PLACEMENT_3D('',#43518,#21154,#21155);
#17762=AXIS2_PLACEMENT_3D('',#43522,#21158,#21159);
#17763=AXIS2_PLACEMENT_3D('',#43523,#21160,#21161);
#17764=AXIS2_PLACEMENT_3D('',#43524,#21162,#21163);
#17765=AXIS2_PLACEMENT_3D('',#43533,#21168,#21169);
#17766=AXIS2_PLACEMENT_3D('',#43535,#21170,#21171);
#17767=AXIS2_PLACEMENT_3D('',#43538,#21173,#21174);
#17768=AXIS2_PLACEMENT_3D('',#43539,#21175,#21176);
#17769=AXIS2_PLACEMENT_3D('',#43543,#21179,#21180);
#17770=AXIS2_PLACEMENT_3D('',#43545,#21181,#21182);
#17771=AXIS2_PLACEMENT_3D('',#43546,#21183,#21184);
#17772=AXIS2_PLACEMENT_3D('',#43547,#21185,#21186);
#17773=AXIS2_PLACEMENT_3D('',#43556,#21191,#21192);
#17774=AXIS2_PLACEMENT_3D('',#43558,#21193,#21194);
#17775=AXIS2_PLACEMENT_3D('',#43560,#21196,#21197);
#17776=AXIS2_PLACEMENT_3D('',#43564,#21200,#21201);
#17777=AXIS2_PLACEMENT_3D('',#43565,#21202,#21203);
#17778=AXIS2_PLACEMENT_3D('',#43566,#21204,#21205);
#17779=AXIS2_PLACEMENT_3D('',#43575,#21210,#21211);
#17780=AXIS2_PLACEMENT_3D('',#43577,#21212,#21213);
#17781=AXIS2_PLACEMENT_3D('',#43579,#21215,#21216);
#17782=AXIS2_PLACEMENT_3D('',#43583,#21219,#21220);
#17783=AXIS2_PLACEMENT_3D('',#43584,#21221,#21222);
#17784=AXIS2_PLACEMENT_3D('',#43585,#21223,#21224);
#17785=AXIS2_PLACEMENT_3D('',#43594,#21229,#21230);
#17786=AXIS2_PLACEMENT_3D('',#43596,#21231,#21232);
#17787=AXIS2_PLACEMENT_3D('',#43598,#21234,#21235);
#17788=AXIS2_PLACEMENT_3D('',#43602,#21238,#21239);
#17789=AXIS2_PLACEMENT_3D('',#43603,#21240,#21241);
#17790=AXIS2_PLACEMENT_3D('',#43604,#21242,#21243);
#17791=AXIS2_PLACEMENT_3D('',#43613,#21248,#21249);
#17792=AXIS2_PLACEMENT_3D('',#43615,#21250,#21251);
#17793=AXIS2_PLACEMENT_3D('',#43617,#21253,#21254);
#17794=AXIS2_PLACEMENT_3D('',#43621,#21257,#21258);
#17795=AXIS2_PLACEMENT_3D('',#43622,#21259,#21260);
#17796=AXIS2_PLACEMENT_3D('',#43623,#21261,#21262);
#17797=AXIS2_PLACEMENT_3D('',#43632,#21267,#21268);
#17798=AXIS2_PLACEMENT_3D('',#43634,#21269,#21270);
#17799=AXIS2_PLACEMENT_3D('',#43636,#21272,#21273);
#17800=AXIS2_PLACEMENT_3D('',#43640,#21276,#21277);
#17801=AXIS2_PLACEMENT_3D('',#43641,#21278,#21279);
#17802=AXIS2_PLACEMENT_3D('',#43642,#21280,#21281);
#17803=AXIS2_PLACEMENT_3D('',#43651,#21286,#21287);
#17804=AXIS2_PLACEMENT_3D('',#43653,#21288,#21289);
#17805=AXIS2_PLACEMENT_3D('',#43655,#21291,#21292);
#17806=AXIS2_PLACEMENT_3D('',#43659,#21295,#21296);
#17807=AXIS2_PLACEMENT_3D('',#43660,#21297,#21298);
#17808=AXIS2_PLACEMENT_3D('',#43661,#21299,#21300);
#17809=AXIS2_PLACEMENT_3D('',#43670,#21305,#21306);
#17810=AXIS2_PLACEMENT_3D('',#43672,#21307,#21308);
#17811=AXIS2_PLACEMENT_3D('',#43674,#21310,#21311);
#17812=AXIS2_PLACEMENT_3D('',#43678,#21314,#21315);
#17813=AXIS2_PLACEMENT_3D('',#43679,#21316,#21317);
#17814=AXIS2_PLACEMENT_3D('',#43680,#21318,#21319);
#17815=AXIS2_PLACEMENT_3D('',#43689,#21324,#21325);
#17816=AXIS2_PLACEMENT_3D('',#43691,#21326,#21327);
#17817=AXIS2_PLACEMENT_3D('',#43693,#21329,#21330);
#17818=AXIS2_PLACEMENT_3D('',#43697,#21333,#21334);
#17819=AXIS2_PLACEMENT_3D('',#43698,#21335,#21336);
#17820=AXIS2_PLACEMENT_3D('',#43699,#21337,#21338);
#17821=AXIS2_PLACEMENT_3D('',#43708,#21343,#21344);
#17822=AXIS2_PLACEMENT_3D('',#43710,#21345,#21346);
#17823=AXIS2_PLACEMENT_3D('',#43712,#21348,#21349);
#17824=AXIS2_PLACEMENT_3D('',#43716,#21352,#21353);
#17825=AXIS2_PLACEMENT_3D('',#43717,#21354,#21355);
#17826=AXIS2_PLACEMENT_3D('',#43718,#21356,#21357);
#17827=AXIS2_PLACEMENT_3D('',#43727,#21362,#21363);
#17828=AXIS2_PLACEMENT_3D('',#43729,#21364,#21365);
#17829=AXIS2_PLACEMENT_3D('',#43731,#21367,#21368);
#17830=AXIS2_PLACEMENT_3D('',#43735,#21371,#21372);
#17831=AXIS2_PLACEMENT_3D('',#43736,#21373,#21374);
#17832=AXIS2_PLACEMENT_3D('',#43737,#21375,#21376);
#17833=AXIS2_PLACEMENT_3D('',#43746,#21381,#21382);
#17834=AXIS2_PLACEMENT_3D('',#43748,#21383,#21384);
#17835=AXIS2_PLACEMENT_3D('',#43750,#21386,#21387);
#17836=AXIS2_PLACEMENT_3D('',#43754,#21390,#21391);
#17837=AXIS2_PLACEMENT_3D('',#43755,#21392,#21393);
#17838=AXIS2_PLACEMENT_3D('',#43756,#21394,#21395);
#17839=AXIS2_PLACEMENT_3D('',#43765,#21400,#21401);
#17840=AXIS2_PLACEMENT_3D('',#43767,#21402,#21403);
#17841=AXIS2_PLACEMENT_3D('',#43769,#21405,#21406);
#17842=AXIS2_PLACEMENT_3D('',#43773,#21409,#21410);
#17843=AXIS2_PLACEMENT_3D('',#43774,#21411,#21412);
#17844=AXIS2_PLACEMENT_3D('',#43775,#21413,#21414);
#17845=AXIS2_PLACEMENT_3D('',#43784,#21419,#21420);
#17846=AXIS2_PLACEMENT_3D('',#43786,#21421,#21422);
#17847=AXIS2_PLACEMENT_3D('',#43788,#21424,#21425);
#17848=AXIS2_PLACEMENT_3D('',#43792,#21428,#21429);
#17849=AXIS2_PLACEMENT_3D('',#43793,#21430,#21431);
#17850=AXIS2_PLACEMENT_3D('',#43794,#21432,#21433);
#17851=AXIS2_PLACEMENT_3D('',#43803,#21438,#21439);
#17852=AXIS2_PLACEMENT_3D('',#43805,#21440,#21441);
#17853=AXIS2_PLACEMENT_3D('',#43807,#21443,#21444);
#17854=AXIS2_PLACEMENT_3D('',#43811,#21447,#21448);
#17855=AXIS2_PLACEMENT_3D('',#43812,#21449,#21450);
#17856=AXIS2_PLACEMENT_3D('',#43813,#21451,#21452);
#17857=AXIS2_PLACEMENT_3D('',#43822,#21457,#21458);
#17858=AXIS2_PLACEMENT_3D('',#43824,#21459,#21460);
#17859=AXIS2_PLACEMENT_3D('',#43826,#21462,#21463);
#17860=AXIS2_PLACEMENT_3D('',#43830,#21466,#21467);
#17861=AXIS2_PLACEMENT_3D('',#43831,#21468,#21469);
#17862=AXIS2_PLACEMENT_3D('',#43832,#21470,#21471);
#17863=AXIS2_PLACEMENT_3D('',#43834,#21472,#21473);
#17864=AXIS2_PLACEMENT_3D('',#43835,#21474,#21475);
#17865=AXIS2_PLACEMENT_3D('',#43837,#21476,#21477);
#17866=AXIS2_PLACEMENT_3D('',#43839,#21479,#21480);
#17867=AXIS2_PLACEMENT_3D('',#43841,#21482,#21483);
#17868=AXIS2_PLACEMENT_3D('',#43842,#21484,#21485);
#17869=AXIS2_PLACEMENT_3D('',#43844,#21486,#21487);
#17870=AXIS2_PLACEMENT_3D('',#43846,#21489,#21490);
#17871=AXIS2_PLACEMENT_3D('',#43848,#21491,#21492);
#17872=AXIS2_PLACEMENT_3D('',#43849,#21493,#21494);
#17873=AXIS2_PLACEMENT_3D('',#43851,#21495,#21496);
#17874=AXIS2_PLACEMENT_3D('',#43853,#21498,#21499);
#17875=AXIS2_PLACEMENT_3D('',#43855,#21500,#21501);
#17876=AXIS2_PLACEMENT_3D('',#43858,#21504,#21505);
#17877=AXIS2_PLACEMENT_3D('',#43860,#21506,#21507);
#17878=AXIS2_PLACEMENT_3D('',#43862,#21509,#21510);
#20599=DIRECTION('axis',(0.,0.,1.));
#20600=DIRECTION('refdir',(1.,0.,0.));
#20601=DIRECTION('center_axis',(1.,0.,0.));
#20602=DIRECTION('ref_axis',(0.,1.,0.));
#20603=DIRECTION('',(-1.,0.,0.));
#20604=DIRECTION('center_axis',(1.,0.,0.));
#20605=DIRECTION('ref_axis',(0.,1.,0.));
#20606=DIRECTION('center_axis',(1.,0.,0.));
#20607=DIRECTION('ref_axis',(0.,1.,0.));
#20608=DIRECTION('',(-1.,0.,0.));
#20609=DIRECTION('center_axis',(1.,0.,0.));
#20610=DIRECTION('ref_axis',(0.,1.,0.));
#20611=DIRECTION('',(-1.,0.,0.));
#20612=DIRECTION('center_axis',(1.,0.,0.));
#20613=DIRECTION('ref_axis',(0.,1.,0.));
#20614=DIRECTION('',(-1.,0.,0.));
#20615=DIRECTION('center_axis',(1.,0.,0.));
#20616=DIRECTION('ref_axis',(0.,1.,0.));
#20617=DIRECTION('',(-1.,0.,0.));
#20618=DIRECTION('center_axis',(1.,0.,0.));
#20619=DIRECTION('ref_axis',(0.,1.,0.));
#20620=DIRECTION('',(-1.,0.,0.));
#20621=DIRECTION('center_axis',(1.,0.,0.));
#20622=DIRECTION('ref_axis',(0.,1.,0.));
#20623=DIRECTION('',(-1.,0.,0.));
#20624=DIRECTION('center_axis',(1.,0.,0.));
#20625=DIRECTION('ref_axis',(0.,1.,0.));
#20626=DIRECTION('',(-1.,0.,0.));
#20627=DIRECTION('center_axis',(1.,0.,0.));
#20628=DIRECTION('ref_axis',(0.,1.,0.));
#20629=DIRECTION('',(-1.,0.,0.));
#20630=DIRECTION('center_axis',(1.,0.,0.));
#20631=DIRECTION('ref_axis',(0.,1.,0.));
#20632=DIRECTION('',(-1.,0.,0.));
#20633=DIRECTION('center_axis',(1.,0.,0.));
#20634=DIRECTION('ref_axis',(0.,1.,0.));
#20635=DIRECTION('',(-1.,0.,0.));
#20636=DIRECTION('center_axis',(1.,0.,0.));
#20637=DIRECTION('ref_axis',(0.,1.,0.));
#20638=DIRECTION('',(-1.,0.,0.));
#20639=DIRECTION('center_axis',(1.,0.,0.));
#20640=DIRECTION('ref_axis',(0.,1.,0.));
#20641=DIRECTION('',(-1.,0.,0.));
#20642=DIRECTION('center_axis',(1.,0.,0.));
#20643=DIRECTION('ref_axis',(0.,0.957230166128618,-0.289327511746427));
#20644=DIRECTION('',(1.,0.,0.));
#20645=DIRECTION('center_axis',(1.,0.,0.));
#20646=DIRECTION('ref_axis',(0.,1.,6.85471472797398E-14));
#20647=DIRECTION('center_axis',(1.,0.,0.));
#20648=DIRECTION('ref_axis',(0.,1.,6.85471472797398E-14));
#20649=DIRECTION('',(1.,0.,0.));
#20650=DIRECTION('center_axis',(1.,0.,0.));
#20651=DIRECTION('ref_axis',(0.,1.,6.85471472797398E-14));
#20652=DIRECTION('',(1.,0.,0.));
#20653=DIRECTION('center_axis',(1.,0.,0.));
#20654=DIRECTION('ref_axis',(0.,1.,6.85471472797398E-14));
#20655=DIRECTION('',(1.,0.,0.));
#20656=DIRECTION('center_axis',(1.,0.,0.));
#20657=DIRECTION('ref_axis',(0.,1.,6.85471472797398E-14));
#20658=DIRECTION('',(1.,0.,0.));
#20659=DIRECTION('center_axis',(1.,0.,0.));
#20660=DIRECTION('ref_axis',(0.,1.,6.85471472797398E-14));
#20661=DIRECTION('',(1.,0.,0.));
#20662=DIRECTION('center_axis',(1.,0.,0.));
#20663=DIRECTION('ref_axis',(0.,1.,6.85471472797398E-14));
#20664=DIRECTION('',(1.,0.,0.));
#20665=DIRECTION('center_axis',(1.,0.,0.));
#20666=DIRECTION('ref_axis',(0.,1.,6.85471472797398E-14));
#20667=DIRECTION('',(1.,0.,0.));
#20668=DIRECTION('center_axis',(1.,0.,0.));
#20669=DIRECTION('ref_axis',(0.,1.,6.85471472797398E-14));
#20670=DIRECTION('',(1.,0.,0.));
#20671=DIRECTION('center_axis',(1.,0.,0.));
#20672=DIRECTION('ref_axis',(0.,1.,6.85471472797398E-14));
#20673=DIRECTION('',(1.,0.,0.));
#20674=DIRECTION('center_axis',(1.,0.,0.));
#20675=DIRECTION('ref_axis',(0.,1.,6.85471472797398E-14));
#20676=DIRECTION('',(1.,0.,0.));
#20677=DIRECTION('center_axis',(1.,0.,0.));
#20678=DIRECTION('ref_axis',(0.,1.,6.85471472797398E-14));
#20679=DIRECTION('',(1.,0.,0.));
#20680=DIRECTION('center_axis',(1.,0.,0.));
#20681=DIRECTION('ref_axis',(0.,0.,-1.));
#20682=DIRECTION('center_axis',(1.,0.,0.));
#20683=DIRECTION('ref_axis',(0.,1.,0.));
#20684=DIRECTION('center_axis',(1.,0.,0.));
#20685=DIRECTION('ref_axis',(0.,1.,0.));
#20686=DIRECTION('center_axis',(-1.,0.,0.));
#20687=DIRECTION('ref_axis',(0.,1.,6.85471472797398E-14));
#20688=DIRECTION('center_axis',(1.,0.,0.));
#20689=DIRECTION('ref_axis',(0.,1.,6.85471472797398E-14));
#20690=DIRECTION('center_axis',(1.,0.,0.));
#20691=DIRECTION('ref_axis',(0.,0.,-1.));
#20692=DIRECTION('center_axis',(-1.,0.,0.));
#20693=DIRECTION('ref_axis',(0.,1.,0.));
#20694=DIRECTION('center_axis',(1.,0.,0.));
#20695=DIRECTION('ref_axis',(0.,0.,-1.));
#20696=DIRECTION('',(-1.,0.,0.));
#20697=DIRECTION('',(-1.,0.,0.));
#20698=DIRECTION('',(-1.,0.,0.));
#20699=DIRECTION('',(-1.,0.,0.));
#20700=DIRECTION('',(-1.,0.,0.));
#20701=DIRECTION('',(-1.,0.,0.));
#20702=DIRECTION('',(-1.,0.,0.));
#20703=DIRECTION('',(-1.,0.,0.));
#20704=DIRECTION('',(-1.,0.,0.));
#20705=DIRECTION('',(-1.,0.,0.));
#20706=DIRECTION('',(-1.,0.,0.));
#20707=DIRECTION('center_axis',(1.,0.,0.));
#20708=DIRECTION('ref_axis',(0.,0.,-1.));
#20709=DIRECTION('center_axis',(0.,0.427000673777987,0.904251306105302));
#20710=DIRECTION('ref_axis',(0.,0.904251306105302,-0.427000673777987));
#20711=DIRECTION('',(0.,0.904251306105302,-0.427000673777987));
#20712=DIRECTION('',(-1.,0.,0.));
#20713=DIRECTION('',(0.,0.904251306105302,-0.427000673777987));
#20714=DIRECTION('',(-1.,0.,0.));
#20715=DIRECTION('center_axis',(0.,-0.514495755427527,0.857492925712544));
#20716=DIRECTION('ref_axis',(0.,0.857492925712544,0.514495755427527));
#20717=DIRECTION('',(0.,0.857492925712544,0.514495755427527));
#20718=DIRECTION('',(-1.,0.,0.));
#20719=DIRECTION('',(0.,0.857492925712544,0.514495755427527));
#20720=DIRECTION('center_axis',(0.,-0.857492925712544,-0.514495755427526));
#20721=DIRECTION('ref_axis',(0.,-0.514495755427526,0.857492925712544));
#20722=DIRECTION('',(0.,-0.514495755427526,0.857492925712544));
#20723=DIRECTION('',(-1.,0.,0.));
#20724=DIRECTION('',(0.,-0.514495755427526,0.857492925712544));
#20725=DIRECTION('center_axis',(0.,0.514495755427526,-0.857492925712544));
#20726=DIRECTION('ref_axis',(0.,-0.857492925712544,-0.514495755427526));
#20727=DIRECTION('',(0.,-0.857492925712544,-0.514495755427526));
#20728=DIRECTION('',(-1.,0.,0.));
#20729=DIRECTION('',(0.,-0.857492925712544,-0.514495755427526));
#20730=DIRECTION('center_axis',(0.,0.857492925712544,0.514495755427527));
#20731=DIRECTION('ref_axis',(0.,0.514495755427527,-0.857492925712544));
#20732=DIRECTION('',(0.,0.514495755427527,-0.857492925712544));
#20733=DIRECTION('',(-1.,0.,0.));
#20734=DIRECTION('',(0.,0.514495755427527,-0.857492925712544));
#20735=DIRECTION('center_axis',(0.,-0.426637779431547,-0.904422581076854));
#20736=DIRECTION('ref_axis',(0.,-0.904422581076854,0.426637779431547));
#20737=DIRECTION('',(0.,-0.904422581076854,0.426637779431547));
#20738=DIRECTION('',(-1.,0.,0.));
#20739=DIRECTION('',(0.,-0.904422581076854,0.426637779431547));
#20740=DIRECTION('center_axis',(0.,0.51449575542753,-0.857492925712542));
#20741=DIRECTION('ref_axis',(0.,-0.857492925712542,-0.51449575542753));
#20742=DIRECTION('',(0.,-0.857492925712542,-0.51449575542753));
#20743=DIRECTION('',(-1.,0.,0.));
#20744=DIRECTION('',(0.,-0.857492925712542,-0.51449575542753));
#20745=DIRECTION('center_axis',(0.,0.857492925712544,0.514495755427527));
#20746=DIRECTION('ref_axis',(0.,0.514495755427527,-0.857492925712544));
#20747=DIRECTION('',(0.,0.514495755427527,-0.857492925712544));
#20748=DIRECTION('',(-1.,0.,0.));
#20749=DIRECTION('',(0.,0.514495755427527,-0.857492925712544));
#20750=DIRECTION('center_axis',(0.,-0.514495755427528,0.857492925712544));
#20751=DIRECTION('ref_axis',(0.,0.857492925712543,0.514495755427528));
#20752=DIRECTION('',(0.,0.857492925712543,0.514495755427528));
#20753=DIRECTION('',(-1.,0.,0.));
#20754=DIRECTION('',(0.,0.857492925712543,0.514495755427528));
#20755=DIRECTION('center_axis',(0.,-0.857492925712544,-0.514495755427527));
#20756=DIRECTION('ref_axis',(0.,-0.514495755427527,0.857492925712544));
#20757=DIRECTION('',(0.,-0.514495755427527,0.857492925712544));
#20758=DIRECTION('',(0.,-0.514495755427527,0.857492925712544));
#20759=DIRECTION('center_axis',(-1.,0.,0.));
#20760=DIRECTION('ref_axis',(0.,0.,1.));
#20761=DIRECTION('',(-1.,0.,0.));
#20762=DIRECTION('',(-1.,0.,0.));
#20763=DIRECTION('',(-1.,0.,0.));
#20764=DIRECTION('',(-1.,0.,0.));
#20765=DIRECTION('',(-1.,0.,0.));
#20766=DIRECTION('',(-1.,0.,0.));
#20767=DIRECTION('',(-1.,0.,0.));
#20768=DIRECTION('',(-1.,0.,0.));
#20769=DIRECTION('',(-1.,0.,0.));
#20770=DIRECTION('',(-1.,0.,0.));
#20771=DIRECTION('',(-1.,0.,0.));
#20772=DIRECTION('center_axis',(1.,0.,0.));
#20773=DIRECTION('ref_axis',(0.,0.,-1.));
#20774=DIRECTION('center_axis',(0.,-0.447213595499958,-0.894427190999916));
#20775=DIRECTION('ref_axis',(0.,-0.894427190999916,0.447213595499958));
#20776=DIRECTION('',(0.,-0.894427190999916,0.447213595499958));
#20777=DIRECTION('',(-1.,0.,0.));
#20778=DIRECTION('',(0.,-0.894427190999916,0.447213595499958));
#20779=DIRECTION('',(-1.,0.,0.));
#20780=DIRECTION('center_axis',(0.,0.894427190999917,-0.447213595499956));
#20781=DIRECTION('ref_axis',(0.,-0.447213595499956,-0.894427190999917));
#20782=DIRECTION('',(0.,-0.447213595499956,-0.894427190999917));
#20783=DIRECTION('',(-1.,0.,0.));
#20784=DIRECTION('',(0.,-0.447213595499956,-0.894427190999917));
#20785=DIRECTION('center_axis',(0.,0.447213595499957,0.894427190999916));
#20786=DIRECTION('ref_axis',(0.,0.894427190999916,-0.447213595499957));
#20787=DIRECTION('',(0.,0.894427190999916,-0.447213595499957));
#20788=DIRECTION('',(-1.,0.,0.));
#20789=DIRECTION('',(0.,0.894427190999916,-0.447213595499957));
#20790=DIRECTION('center_axis',(0.,0.894427190999916,-0.447213595499958));
#20791=DIRECTION('ref_axis',(0.,-0.447213595499958,-0.894427190999916));
#20792=DIRECTION('',(0.,-0.447213595499958,-0.894427190999916));
#20793=DIRECTION('',(-1.,0.,0.));
#20794=DIRECTION('',(0.,-0.447213595499958,-0.894427190999916));
#20795=DIRECTION('center_axis',(0.,-0.447213595499958,-0.894427190999916));
#20796=DIRECTION('ref_axis',(0.,-0.894427190999916,0.447213595499958));
#20797=DIRECTION('',(0.,-0.894427190999916,0.447213595499958));
#20798=DIRECTION('',(-1.,0.,0.));
#20799=DIRECTION('',(0.,-0.894427190999916,0.447213595499958));
#20800=DIRECTION('center_axis',(0.,0.894427190999917,-0.447213595499956));
#20801=DIRECTION('ref_axis',(0.,-0.447213595499956,-0.894427190999917));
#20802=DIRECTION('',(0.,-0.447213595499956,-0.894427190999917));
#20803=DIRECTION('',(-1.,0.,0.));
#20804=DIRECTION('',(0.,-0.447213595499956,-0.894427190999917));
#20805=DIRECTION('center_axis',(0.,0.447213595499958,0.894427190999916));
#20806=DIRECTION('ref_axis',(0.,0.894427190999916,-0.447213595499958));
#20807=DIRECTION('',(0.,0.894427190999916,-0.447213595499958));
#20808=DIRECTION('',(-1.,0.,0.));
#20809=DIRECTION('',(0.,0.894427190999916,-0.447213595499958));
#20810=DIRECTION('center_axis',(0.,-0.894427190999916,0.447213595499958));
#20811=DIRECTION('ref_axis',(0.,0.447213595499958,0.894427190999916));
#20812=DIRECTION('',(0.,0.447213595499958,0.894427190999916));
#20813=DIRECTION('',(-1.,0.,0.));
#20814=DIRECTION('',(0.,0.447213595499958,0.894427190999916));
#20815=DIRECTION('center_axis',(0.,-0.447213595499959,-0.894427190999915));
#20816=DIRECTION('ref_axis',(0.,-0.894427190999915,0.447213595499959));
#20817=DIRECTION('',(0.,-0.894427190999915,0.447213595499959));
#20818=DIRECTION('',(-1.,0.,0.));
#20819=DIRECTION('',(0.,-0.894427190999915,0.447213595499959));
#20820=DIRECTION('center_axis',(0.,0.894427190999916,-0.447213595499958));
#20821=DIRECTION('ref_axis',(0.,-0.447213595499958,-0.894427190999916));
#20822=DIRECTION('',(0.,-0.447213595499958,-0.894427190999916));
#20823=DIRECTION('',(0.,-0.447213595499958,-0.894427190999916));
#20824=DIRECTION('center_axis',(-1.,0.,0.));
#20825=DIRECTION('ref_axis',(0.,0.,1.));
#20826=DIRECTION('center_axis',(0.,-0.447213595499958,-0.894427190999916));
#20827=DIRECTION('ref_axis',(0.,-0.894427190999916,0.447213595499958));
#20828=DIRECTION('',(0.,-0.894427190999916,0.447213595499958));
#20829=DIRECTION('',(-1.,0.,0.));
#20830=DIRECTION('',(0.,-0.894427190999916,0.447213595499958));
#20831=DIRECTION('',(-1.,0.,0.));
#20832=DIRECTION('center_axis',(0.,0.894427190999917,-0.447213595499956));
#20833=DIRECTION('ref_axis',(0.,-0.447213595499956,-0.894427190999917));
#20834=DIRECTION('',(0.,-0.447213595499956,-0.894427190999917));
#20835=DIRECTION('',(-1.,0.,0.));
#20836=DIRECTION('',(0.,-0.447213595499956,-0.894427190999917));
#20837=DIRECTION('center_axis',(0.,0.447213595499957,0.894427190999916));
#20838=DIRECTION('ref_axis',(0.,0.894427190999916,-0.447213595499957));
#20839=DIRECTION('',(0.,0.894427190999917,-0.447213595499957));
#20840=DIRECTION('',(-1.,0.,0.));
#20841=DIRECTION('',(0.,0.894427190999916,-0.447213595499957));
#20842=DIRECTION('center_axis',(0.,0.894427190999916,-0.447213595499958));
#20843=DIRECTION('ref_axis',(0.,-0.447213595499958,-0.894427190999916));
#20844=DIRECTION('',(0.,-0.447213595499958,-0.894427190999916));
#20845=DIRECTION('',(-1.,0.,0.));
#20846=DIRECTION('',(0.,-0.447213595499958,-0.894427190999916));
#20847=DIRECTION('center_axis',(0.,-0.447213595499958,-0.894427190999916));
#20848=DIRECTION('ref_axis',(0.,-0.894427190999916,0.447213595499958));
#20849=DIRECTION('',(0.,-0.894427190999916,0.447213595499958));
#20850=DIRECTION('',(-1.,0.,0.));
#20851=DIRECTION('',(0.,-0.894427190999916,0.447213595499958));
#20852=DIRECTION('center_axis',(0.,0.894427190999916,-0.447213595499958));
#20853=DIRECTION('ref_axis',(0.,-0.447213595499958,-0.894427190999916));
#20854=DIRECTION('',(0.,-0.447213595499958,-0.894427190999916));
#20855=DIRECTION('',(-1.,0.,0.));
#20856=DIRECTION('',(0.,-0.447213595499958,-0.894427190999916));
#20857=DIRECTION('center_axis',(0.,0.447213595499958,0.894427190999916));
#20858=DIRECTION('ref_axis',(0.,0.894427190999916,-0.447213595499958));
#20859=DIRECTION('',(0.,0.894427190999916,-0.447213595499958));
#20860=DIRECTION('',(-1.,0.,0.));
#20861=DIRECTION('',(0.,0.894427190999916,-0.447213595499958));
#20862=DIRECTION('center_axis',(0.,-0.894427190999916,0.447213595499958));
#20863=DIRECTION('ref_axis',(0.,0.447213595499958,0.894427190999916));
#20864=DIRECTION('',(0.,0.447213595499958,0.894427190999916));
#20865=DIRECTION('',(-1.,0.,0.));
#20866=DIRECTION('',(0.,0.447213595499958,0.894427190999916));
#20867=DIRECTION('center_axis',(0.,-0.447213595499957,-0.894427190999916));
#20868=DIRECTION('ref_axis',(0.,-0.894427190999916,0.447213595499957));
#20869=DIRECTION('',(0.,-0.894427190999916,0.447213595499957));
#20870=DIRECTION('',(-1.,0.,0.));
#20871=DIRECTION('',(0.,-0.894427190999916,0.447213595499957));
#20872=DIRECTION('center_axis',(0.,0.894427190999916,-0.447213595499958));
#20873=DIRECTION('ref_axis',(0.,-0.447213595499958,-0.894427190999916));
#20874=DIRECTION('',(0.,-0.447213595499958,-0.894427190999916));
#20875=DIRECTION('',(0.,-0.447213595499958,-0.894427190999916));
#20876=DIRECTION('center_axis',(-1.,0.,0.));
#20877=DIRECTION('ref_axis',(0.,0.,1.));
#20878=DIRECTION('center_axis',(-1.,0.,0.));
#20879=DIRECTION('ref_axis',(0.,0.,1.));
#20880=DIRECTION('center_axis',(1.,0.,0.));
#20881=DIRECTION('ref_axis',(0.,0.,-1.));
#20882=DIRECTION('center_axis',(1.,0.,0.));
#20883=DIRECTION('ref_axis',(0.,0.,-1.));
#20884=DIRECTION('center_axis',(1.,0.,0.));
#20885=DIRECTION('ref_axis',(0.,1.,0.));
#20886=DIRECTION('',(1.,0.,0.));
#20887=DIRECTION('center_axis',(-1.,0.,0.));
#20888=DIRECTION('ref_axis',(0.,1.,0.));
#20889=DIRECTION('center_axis',(1.,0.,0.));
#20890=DIRECTION('ref_axis',(0.,1.,0.));
#20891=DIRECTION('',(1.,0.,0.));
#20892=DIRECTION('center_axis',(1.,0.,0.));
#20893=DIRECTION('ref_axis',(0.,1.,0.));
#20894=DIRECTION('center_axis',(1.,0.,0.));
#20895=DIRECTION('ref_axis',(0.,0.,-1.));
#20896=DIRECTION('center_axis',(0.,-0.599220281862479,0.800584195325296));
#20897=DIRECTION('ref_axis',(0.,-0.800584195325296,-0.599220281862479));
#20898=DIRECTION('',(-1.,0.,0.));
#20899=DIRECTION('',(0.,-0.800584195325296,-0.599220281862479));
#20900=DIRECTION('',(1.,0.,0.));
#20901=DIRECTION('',(0.,-0.800584195325296,-0.599220281862479));
#20902=DIRECTION('center_axis',(1.,0.,0.));
#20903=DIRECTION('ref_axis',(0.,-0.20791169081776,-0.978147600733805));
#20904=DIRECTION('center_axis',(-1.,0.,0.));
#20905=DIRECTION('ref_axis',(0.,1.,0.));
#20906=DIRECTION('',(0.,0.4876452091922,-0.873041894728939));
#20907=DIRECTION('center_axis',(0.,-0.873041894728939,-0.4876452091922));
#20908=DIRECTION('ref_axis',(0.,0.4876452091922,-0.873041894728939));
#20909=DIRECTION('',(1.,0.,0.));
#20910=DIRECTION('',(0.,0.4876452091922,-0.873041894728939));
#20911=DIRECTION('center_axis',(1.,0.,0.));
#20912=DIRECTION('ref_axis',(0.,-0.20791169081776,-0.978147600733805));
#20913=DIRECTION('center_axis',(1.,0.,0.));
#20914=DIRECTION('ref_axis',(0.,1.,0.));
#20915=DIRECTION('center_axis',(0.,-0.419675067322761,0.907674411817165));
#20916=DIRECTION('ref_axis',(0.,-0.907674411817165,-0.419675067322761));
#20917=DIRECTION('',(-1.,0.,0.));
#20918=DIRECTION('',(0.,-0.907674411817165,-0.419675067322761));
#20919=DIRECTION('',(1.,0.,0.));
#20920=DIRECTION('',(0.,-0.907674411817165,-0.419675067322761));
#20921=DIRECTION('center_axis',(1.,0.,0.));
#20922=DIRECTION('ref_axis',(0.,-0.406736643075801,-0.913545457642601));
#20923=DIRECTION('center_axis',(-1.,0.,0.));
#20924=DIRECTION('ref_axis',(0.,1.,0.));
#20925=DIRECTION('',(0.,0.295473374892851,-0.955350974631538));
#20926=DIRECTION('center_axis',(0.,-0.955350974631538,-0.295473374892851));
#20927=DIRECTION('ref_axis',(0.,0.295473374892851,-0.955350974631538));
#20928=DIRECTION('',(1.,0.,0.));
#20929=DIRECTION('',(0.,0.295473374892851,-0.955350974631538));
#20930=DIRECTION('center_axis',(1.,0.,0.));
#20931=DIRECTION('ref_axis',(0.,-0.406736643075801,-0.913545457642601));
#20932=DIRECTION('center_axis',(1.,0.,0.));
#20933=DIRECTION('ref_axis',(0.,1.,0.));
#20934=DIRECTION('center_axis',(0.,-0.221788038516636,0.97509490100756));
#20935=DIRECTION('ref_axis',(0.,-0.97509490100756,-0.221788038516636));
#20936=DIRECTION('',(-1.,0.,0.));
#20937=DIRECTION('',(0.,-0.97509490100756,-0.221788038516636));
#20938=DIRECTION('',(1.,0.,0.));
#20939=DIRECTION('',(0.,-0.97509490100756,-0.221788038516636));
#20940=DIRECTION('center_axis',(1.,0.,0.));
#20941=DIRECTION('ref_axis',(0.,-0.587785252292473,-0.809016994374947));
#20942=DIRECTION('center_axis',(-1.,0.,0.));
#20943=DIRECTION('ref_axis',(0.,1.,0.));
#20944=DIRECTION('',(0.,0.0903879362721259,-0.995906632660144));
#20945=DIRECTION('center_axis',(0.,-0.995906632660144,-0.0903879362721259));
#20946=DIRECTION('ref_axis',(0.,0.0903879362721259,-0.995906632660144));
#20947=DIRECTION('',(1.,0.,0.));
#20948=DIRECTION('',(0.,0.0903879362721259,-0.995906632660144));
#20949=DIRECTION('center_axis',(1.,0.,0.));
#20950=DIRECTION('ref_axis',(0.,-0.587785252292473,-0.809016994374947));
#20951=DIRECTION('center_axis',(1.,0.,0.));
#20952=DIRECTION('ref_axis',(0.,1.,0.));
#20953=DIRECTION('center_axis',(0.,-0.0142078081702462,0.999899063999461));
#20954=DIRECTION('ref_axis',(0.,-0.999899063999461,-0.0142078081702462));
#20955=DIRECTION('',(-1.,0.,0.));
#20956=DIRECTION('',(0.,-0.999899063999461,-0.0142078081702462));
#20957=DIRECTION('',(1.,0.,0.));
#20958=DIRECTION('',(0.,-0.999899063999461,-0.0142078081702462));
#20959=DIRECTION('center_axis',(1.,0.,0.));
#20960=DIRECTION('ref_axis',(0.,-0.743144825477395,-0.669130606358858));
#20961=DIRECTION('center_axis',(-1.,0.,0.));
#20962=DIRECTION('ref_axis',(0.,1.,0.));
#20963=DIRECTION('',(0.,-0.118647888893132,-0.992936391951268));
#20964=DIRECTION('center_axis',(0.,-0.992936391951268,0.118647888893132));
#20965=DIRECTION('ref_axis',(0.,-0.118647888893132,-0.992936391951268));
#20966=DIRECTION('',(1.,0.,0.));
#20967=DIRECTION('',(0.,-0.118647888893132,-0.992936391951268));
#20968=DIRECTION('center_axis',(1.,0.,0.));
#20969=DIRECTION('ref_axis',(0.,-0.743144825477395,-0.669130606358858));
#20970=DIRECTION('center_axis',(1.,0.,0.));
#20971=DIRECTION('ref_axis',(0.,1.,0.));
#20972=DIRECTION('center_axis',(0.,0.193993371569811,0.981002839846541));
#20973=DIRECTION('ref_axis',(0.,-0.981002839846541,0.193993371569811));
#20974=DIRECTION('',(-1.,0.,0.));
#20975=DIRECTION('',(0.,-0.981002839846541,0.193993371569811));
#20976=DIRECTION('',(1.,0.,0.));
#20977=DIRECTION('',(0.,-0.981002839846541,0.193993371569811));
#20978=DIRECTION('center_axis',(1.,0.,0.));
#20979=DIRECTION('ref_axis',(0.,-0.866025403784439,-0.499999999999999));
#20980=DIRECTION('center_axis',(-1.,0.,0.));
#20981=DIRECTION('ref_axis',(0.,1.,0.));
#20982=DIRECTION('',(0.,-0.322498231978022,-0.946570066276686));
#20983=DIRECTION('center_axis',(0.,-0.946570066276686,0.322498231978022));
#20984=DIRECTION('ref_axis',(0.,-0.322498231978022,-0.946570066276686));
#20985=DIRECTION('',(1.,0.,0.));
#20986=DIRECTION('',(0.,-0.322498231978022,-0.946570066276686));
#20987=DIRECTION('center_axis',(1.,0.,0.));
#20988=DIRECTION('ref_axis',(0.,-0.866025403784439,-0.499999999999999));
#20989=DIRECTION('center_axis',(1.,0.,0.));
#20990=DIRECTION('ref_axis',(0.,1.,0.));
#20991=DIRECTION('center_axis',(0.,0.393716110088789,0.919232084218427));
#20992=DIRECTION('ref_axis',(0.,-0.919232084218427,0.393716110088789));
#20993=DIRECTION('',(-1.,0.,0.));
#20994=DIRECTION('',(0.,-0.919232084218427,0.393716110088789));
#20995=DIRECTION('',(1.,0.,0.));
#20996=DIRECTION('',(0.,-0.919232084218427,0.393716110088789));
#20997=DIRECTION('center_axis',(1.,0.,0.));
#20998=DIRECTION('ref_axis',(0.,-0.951056516295154,-0.309016994374947));
#20999=DIRECTION('center_axis',(-1.,0.,0.));
#21000=DIRECTION('ref_axis',(0.,1.,0.));
#21001=DIRECTION('',(0.,-0.51225385480726,-0.858834086558692));
#21002=DIRECTION('center_axis',(0.,-0.858834086558692,0.51225385480726));
#21003=DIRECTION('ref_axis',(0.,-0.51225385480726,-0.858834086558692));
#21004=DIRECTION('',(1.,0.,0.));
#21005=DIRECTION('',(0.,-0.51225385480726,-0.858834086558692));
#21006=DIRECTION('center_axis',(1.,0.,0.));
#21007=DIRECTION('ref_axis',(0.,-0.951056516295154,-0.309016994374947));
#21008=DIRECTION('center_axis',(1.,0.,0.));
#21009=DIRECTION('ref_axis',(0.,1.,0.));
#21010=DIRECTION('center_axis',(0.,0.576231565337382,0.817286475545038));
#21011=DIRECTION('ref_axis',(0.,-0.817286475545038,0.576231565337382));
#21012=DIRECTION('',(-1.,0.,0.));
#21013=DIRECTION('',(0.,-0.817286475545038,0.576231565337382));
#21014=DIRECTION('',(1.,0.,0.));
#21015=DIRECTION('',(0.,-0.817286475545038,0.576231565337382));
#21016=DIRECTION('center_axis',(1.,0.,0.));
#21017=DIRECTION('ref_axis',(0.,-0.994521895368273,-0.104528463267653));
#21018=DIRECTION('center_axis',(-1.,0.,0.));
#21019=DIRECTION('ref_axis',(0.,1.,0.));
#21020=DIRECTION('',(0.,-0.679621526114708,-0.733562936114901));
#21021=DIRECTION('center_axis',(0.,-0.733562936114901,0.679621526114709));
#21022=DIRECTION('ref_axis',(0.,-0.679621526114708,-0.733562936114901));
#21023=DIRECTION('',(1.,0.,0.));
#21024=DIRECTION('',(0.,-0.679621526114708,-0.733562936114901));
#21025=DIRECTION('center_axis',(1.,0.,0.));
#21026=DIRECTION('ref_axis',(0.,-0.994521895368273,-0.104528463267653));
#21027=DIRECTION('center_axis',(1.,0.,0.));
#21028=DIRECTION('ref_axis',(0.,1.,0.));
#21029=DIRECTION('center_axis',(0.,0.733562936114902,0.679621526114708));
#21030=DIRECTION('ref_axis',(0.,-0.679621526114708,0.733562936114902));
#21031=DIRECTION('',(-1.,0.,0.));
#21032=DIRECTION('',(0.,-0.679621526114708,0.733562936114902));
#21033=DIRECTION('',(1.,0.,0.));
#21034=DIRECTION('',(0.,-0.679621526114708,0.733562936114902));
#21035=DIRECTION('center_axis',(1.,0.,0.));
#21036=DIRECTION('ref_axis',(0.,-0.994521895368273,0.104528463267654));
#21037=DIRECTION('center_axis',(-1.,0.,0.));
#21038=DIRECTION('ref_axis',(0.,1.,0.));
#21039=DIRECTION('',(0.,-0.817286475545039,-0.576231565337381));
#21040=DIRECTION('center_axis',(0.,-0.576231565337381,0.817286475545039));
#21041=DIRECTION('ref_axis',(0.,-0.817286475545039,-0.576231565337381));
#21042=DIRECTION('',(1.,0.,0.));
#21043=DIRECTION('',(0.,-0.817286475545039,-0.576231565337381));
#21044=DIRECTION('center_axis',(1.,0.,0.));
#21045=DIRECTION('ref_axis',(0.,-0.994521895368273,0.104528463267654));
#21046=DIRECTION('center_axis',(1.,0.,0.));
#21047=DIRECTION('ref_axis',(0.,1.,0.));
#21048=DIRECTION('center_axis',(0.,0.858834086558692,0.51225385480726));
#21049=DIRECTION('ref_axis',(0.,-0.51225385480726,0.858834086558692));
#21050=DIRECTION('',(-1.,0.,0.));
#21051=DIRECTION('',(0.,-0.51225385480726,0.858834086558692));
#21052=DIRECTION('',(1.,0.,0.));
#21053=DIRECTION('',(0.,-0.51225385480726,0.858834086558692));
#21054=DIRECTION('center_axis',(1.,0.,0.));
#21055=DIRECTION('ref_axis',(0.,-0.951056516295153,0.309016994374948));
#21056=DIRECTION('center_axis',(-1.,0.,0.));
#21057=DIRECTION('ref_axis',(0.,1.,0.));
#21058=DIRECTION('',(0.,-0.919232084218427,-0.393716110088789));
#21059=DIRECTION('center_axis',(0.,-0.393716110088789,0.919232084218427));
#21060=DIRECTION('ref_axis',(0.,-0.919232084218427,-0.393716110088789));
#21061=DIRECTION('',(1.,0.,0.));
#21062=DIRECTION('',(0.,-0.919232084218427,-0.393716110088789));
#21063=DIRECTION('center_axis',(1.,0.,0.));
#21064=DIRECTION('ref_axis',(0.,-0.951056516295153,0.309016994374948));
#21065=DIRECTION('center_axis',(1.,0.,0.));
#21066=DIRECTION('ref_axis',(0.,1.,0.));
#21067=DIRECTION('center_axis',(0.,0.946570066276687,0.322498231978021));
#21068=DIRECTION('ref_axis',(0.,-0.322498231978021,0.946570066276686));
#21069=DIRECTION('',(-1.,0.,0.));
#21070=DIRECTION('',(0.,-0.322498231978021,0.946570066276686));
#21071=DIRECTION('',(1.,0.,0.));
#21072=DIRECTION('',(0.,-0.322498231978021,0.946570066276686));
#21073=DIRECTION('center_axis',(1.,0.,0.));
#21074=DIRECTION('ref_axis',(0.,-0.866025403784438,0.5));
#21075=DIRECTION('center_axis',(-1.,0.,0.));
#21076=DIRECTION('ref_axis',(0.,1.,0.));
#21077=DIRECTION('',(0.,-0.981002839846541,-0.193993371569809));
#21078=DIRECTION('center_axis',(0.,-0.193993371569809,0.981002839846541));
#21079=DIRECTION('ref_axis',(0.,-0.981002839846541,-0.193993371569809));
#21080=DIRECTION('',(1.,0.,0.));
#21081=DIRECTION('',(0.,-0.981002839846541,-0.193993371569809));
#21082=DIRECTION('center_axis',(1.,0.,0.));
#21083=DIRECTION('ref_axis',(0.,-0.866025403784438,0.5));
#21084=DIRECTION('center_axis',(1.,0.,0.));
#21085=DIRECTION('ref_axis',(0.,1.,0.));
#21086=DIRECTION('center_axis',(0.,0.992936391951269,0.118647888893131));
#21087=DIRECTION('ref_axis',(0.,-0.118647888893131,0.992936391951268));
#21088=DIRECTION('',(-1.,0.,0.));
#21089=DIRECTION('',(0.,-0.118647888893131,0.992936391951268));
#21090=DIRECTION('',(1.,0.,0.));
#21091=DIRECTION('',(0.,-0.118647888893131,0.992936391951268));
#21092=DIRECTION('center_axis',(1.,0.,0.));
#21093=DIRECTION('ref_axis',(0.,-0.743144825477394,0.669130606358858));
#21094=DIRECTION('center_axis',(-1.,0.,0.));
#21095=DIRECTION('ref_axis',(0.,1.,0.));
#21096=DIRECTION('',(0.,-0.999899063999461,0.014207808170247));
#21097=DIRECTION('center_axis',(0.,0.014207808170247,0.999899063999461));
#21098=DIRECTION('ref_axis',(0.,-0.999899063999461,0.014207808170247));
#21099=DIRECTION('',(1.,0.,0.));
#21100=DIRECTION('',(0.,-0.999899063999461,0.014207808170247));
#21101=DIRECTION('center_axis',(1.,0.,0.));
#21102=DIRECTION('ref_axis',(0.,-0.743144825477394,0.669130606358858));
#21103=DIRECTION('center_axis',(1.,0.,0.));
#21104=DIRECTION('ref_axis',(0.,1.,0.));
#21105=DIRECTION('center_axis',(0.,0.995906632660144,-0.0903879362721262));
#21106=DIRECTION('ref_axis',(0.,0.0903879362721261,0.995906632660144));
#21107=DIRECTION('',(-1.,0.,0.));
#21108=DIRECTION('',(0.,0.0903879362721261,0.995906632660144));
#21109=DIRECTION('',(1.,0.,0.));
#21110=DIRECTION('',(0.,0.0903879362721261,0.995906632660144));
#21111=DIRECTION('center_axis',(1.,0.,0.));
#21112=DIRECTION('ref_axis',(0.,-0.587785252292473,0.809016994374947));
#21113=DIRECTION('center_axis',(-1.,0.,0.));
#21114=DIRECTION('ref_axis',(0.,1.,0.));
#21115=DIRECTION('',(0.,-0.97509490100756,0.221788038516636));
#21116=DIRECTION('center_axis',(0.,0.221788038516636,0.97509490100756));
#21117=DIRECTION('ref_axis',(0.,-0.97509490100756,0.221788038516636));
#21118=DIRECTION('',(1.,0.,0.));
#21119=DIRECTION('',(0.,-0.97509490100756,0.221788038516636));
#21120=DIRECTION('center_axis',(1.,0.,0.));
#21121=DIRECTION('ref_axis',(0.,-0.587785252292473,0.809016994374947));
#21122=DIRECTION('center_axis',(1.,0.,0.));
#21123=DIRECTION('ref_axis',(0.,1.,0.));
#21124=DIRECTION('center_axis',(0.,0.955350974631537,-0.295473374892852));
#21125=DIRECTION('ref_axis',(0.,0.295473374892852,0.955350974631537));
#21126=DIRECTION('',(-1.,0.,0.));
#21127=DIRECTION('',(0.,0.295473374892852,0.955350974631537));
#21128=DIRECTION('',(1.,0.,0.));
#21129=DIRECTION('',(0.,0.295473374892852,0.955350974631537));
#21130=DIRECTION('center_axis',(1.,0.,0.));
#21131=DIRECTION('ref_axis',(0.,-0.4067366430758,0.913545457642601));
#21132=DIRECTION('center_axis',(-1.,0.,0.));
#21133=DIRECTION('ref_axis',(0.,1.,0.));
#21134=DIRECTION('',(0.,-0.907674411817164,0.419675067322762));
#21135=DIRECTION('center_axis',(0.,0.419675067322762,0.907674411817164));
#21136=DIRECTION('ref_axis',(0.,-0.907674411817164,0.419675067322762));
#21137=DIRECTION('',(1.,0.,0.));
#21138=DIRECTION('',(0.,-0.907674411817164,0.419675067322762));
#21139=DIRECTION('center_axis',(1.,0.,0.));
#21140=DIRECTION('ref_axis',(0.,-0.4067366430758,0.913545457642601));
#21141=DIRECTION('center_axis',(1.,0.,0.));
#21142=DIRECTION('ref_axis',(0.,1.,0.));
#21143=DIRECTION('center_axis',(0.,0.873041894728938,-0.487645209192201));
#21144=DIRECTION('ref_axis',(0.,0.487645209192201,0.873041894728938));
#21145=DIRECTION('',(-1.,0.,0.));
#21146=DIRECTION('',(0.,0.487645209192201,0.873041894728938));
#21147=DIRECTION('',(1.,0.,0.));
#21148=DIRECTION('',(0.,0.487645209192201,0.873041894728938));
#21149=DIRECTION('center_axis',(1.,0.,0.));
#21150=DIRECTION('ref_axis',(0.,-0.207911690817759,0.978147600733806));
#21151=DIRECTION('center_axis',(-1.,0.,0.));
#21152=DIRECTION('ref_axis',(0.,1.,0.));
#21153=DIRECTION('',(0.,-0.800584195325295,0.59922028186248));
#21154=DIRECTION('center_axis',(0.,0.59922028186248,0.800584195325295));
#21155=DIRECTION('ref_axis',(0.,-0.800584195325295,0.59922028186248));
#21156=DIRECTION('',(1.,0.,0.));
#21157=DIRECTION('',(0.,-0.800584195325295,0.59922028186248));
#21158=DIRECTION('center_axis',(1.,0.,0.));
#21159=DIRECTION('ref_axis',(0.,-0.207911690817759,0.978147600733806));
#21160=DIRECTION('center_axis',(1.,0.,0.));
#21161=DIRECTION('ref_axis',(0.,1.,0.));
#21162=DIRECTION('center_axis',(0.,0.752576694706876,-0.65850460786852));
#21163=DIRECTION('ref_axis',(0.,0.65850460786852,0.752576694706876));
#21164=DIRECTION('',(-1.,0.,0.));
#21165=DIRECTION('',(0.,0.65850460786852,0.752576694706876));
#21166=DIRECTION('',(1.,0.,0.));
#21167=DIRECTION('',(0.,0.65850460786852,0.752576694706876));
#21168=DIRECTION('center_axis',(1.,0.,0.));
#21169=DIRECTION('ref_axis',(0.,1.22464679914735E-16,1.));
#21170=DIRECTION('center_axis',(-1.,0.,0.));
#21171=DIRECTION('ref_axis',(0.,1.,0.));
#21172=DIRECTION('',(0.,-0.658504607868519,0.752576694706877));
#21173=DIRECTION('center_axis',(-1.,0.,0.));
#21174=DIRECTION('ref_axis',(0.,1.,0.));
#21175=DIRECTION('center_axis',(0.,0.752576694706877,0.658504607868519));
#21176=DIRECTION('ref_axis',(0.,-0.658504607868519,0.752576694706877));
#21177=DIRECTION('',(1.,0.,0.));
#21178=DIRECTION('',(0.,-0.658504607868519,0.752576694706877));
#21179=DIRECTION('center_axis',(1.,0.,0.));
#21180=DIRECTION('ref_axis',(0.,1.22464679914735E-16,1.));
#21181=DIRECTION('center_axis',(1.,0.,0.));
#21182=DIRECTION('ref_axis',(0.,1.,0.));
#21183=DIRECTION('center_axis',(1.,0.,0.));
#21184=DIRECTION('ref_axis',(0.,1.,0.));
#21185=DIRECTION('center_axis',(0.,0.599220281862479,-0.800584195325296));
#21186=DIRECTION('ref_axis',(0.,0.800584195325295,0.599220281862479));
#21187=DIRECTION('',(-1.,0.,0.));
#21188=DIRECTION('',(0.,0.800584195325295,0.599220281862479));
#21189=DIRECTION('',(1.,0.,0.));
#21190=DIRECTION('',(0.,0.800584195325295,0.599220281862479));
#21191=DIRECTION('center_axis',(1.,0.,0.));
#21192=DIRECTION('ref_axis',(0.,0.20791169081776,0.978147600733805));
#21193=DIRECTION('center_axis',(-1.,0.,0.));
#21194=DIRECTION('ref_axis',(0.,1.,0.));
#21195=DIRECTION('',(0.,-0.4876452091922,0.873041894728939));
#21196=DIRECTION('center_axis',(0.,0.873041894728939,0.4876452091922));
#21197=DIRECTION('ref_axis',(0.,-0.4876452091922,0.873041894728939));
#21198=DIRECTION('',(1.,0.,0.));
#21199=DIRECTION('',(0.,-0.4876452091922,0.873041894728939));
#21200=DIRECTION('center_axis',(1.,0.,0.));
#21201=DIRECTION('ref_axis',(0.,0.20791169081776,0.978147600733805));
#21202=DIRECTION('center_axis',(1.,0.,0.));
#21203=DIRECTION('ref_axis',(0.,1.,0.));
#21204=DIRECTION('center_axis',(0.,0.419675067322761,-0.907674411817165));
#21205=DIRECTION('ref_axis',(0.,0.907674411817165,0.419675067322761));
#21206=DIRECTION('',(-1.,0.,0.));
#21207=DIRECTION('',(0.,0.907674411817165,0.419675067322761));
#21208=DIRECTION('',(1.,0.,0.));
#21209=DIRECTION('',(0.,0.907674411817165,0.419675067322761));
#21210=DIRECTION('center_axis',(1.,0.,0.));
#21211=DIRECTION('ref_axis',(0.,0.4067366430758,0.913545457642601));
#21212=DIRECTION('center_axis',(-1.,0.,0.));
#21213=DIRECTION('ref_axis',(0.,1.,0.));
#21214=DIRECTION('',(0.,-0.295473374892852,0.955350974631537));
#21215=DIRECTION('center_axis',(0.,0.955350974631537,0.295473374892852));
#21216=DIRECTION('ref_axis',(0.,-0.295473374892852,0.955350974631537));
#21217=DIRECTION('',(1.,0.,0.));
#21218=DIRECTION('',(0.,-0.295473374892852,0.955350974631537));
#21219=DIRECTION('center_axis',(1.,0.,0.));
#21220=DIRECTION('ref_axis',(0.,0.4067366430758,0.913545457642601));
#21221=DIRECTION('center_axis',(1.,0.,0.));
#21222=DIRECTION('ref_axis',(0.,1.,0.));
#21223=DIRECTION('center_axis',(0.,0.221788038516636,-0.97509490100756));
#21224=DIRECTION('ref_axis',(0.,0.97509490100756,0.221788038516636));
#21225=DIRECTION('',(-1.,0.,0.));
#21226=DIRECTION('',(0.,0.97509490100756,0.221788038516636));
#21227=DIRECTION('',(1.,0.,0.));
#21228=DIRECTION('',(0.,0.97509490100756,0.221788038516636));
#21229=DIRECTION('center_axis',(1.,0.,0.));
#21230=DIRECTION('ref_axis',(0.,0.587785252292473,0.809016994374947));
#21231=DIRECTION('center_axis',(-1.,0.,0.));
#21232=DIRECTION('ref_axis',(0.,1.,0.));
#21233=DIRECTION('',(0.,-0.0903879362721259,0.995906632660144));
#21234=DIRECTION('center_axis',(0.,0.995906632660144,0.0903879362721259));
#21235=DIRECTION('ref_axis',(0.,-0.0903879362721259,0.995906632660144));
#21236=DIRECTION('',(1.,0.,0.));
#21237=DIRECTION('',(0.,-0.0903879362721259,0.995906632660144));
#21238=DIRECTION('center_axis',(1.,0.,0.));
#21239=DIRECTION('ref_axis',(0.,0.587785252292473,0.809016994374947));
#21240=DIRECTION('center_axis',(1.,0.,0.));
#21241=DIRECTION('ref_axis',(0.,1.,0.));
#21242=DIRECTION('center_axis',(0.,0.0142078081702464,-0.999899063999461));
#21243=DIRECTION('ref_axis',(0.,0.999899063999461,0.0142078081702464));
#21244=DIRECTION('',(-1.,0.,0.));
#21245=DIRECTION('',(0.,0.999899063999461,0.0142078081702464));
#21246=DIRECTION('',(1.,0.,0.));
#21247=DIRECTION('',(0.,0.999899063999461,0.0142078081702464));
#21248=DIRECTION('center_axis',(1.,0.,0.));
#21249=DIRECTION('ref_axis',(0.,0.743144825477394,0.669130606358858));
#21250=DIRECTION('center_axis',(-1.,0.,0.));
#21251=DIRECTION('ref_axis',(0.,1.,0.));
#21252=DIRECTION('',(0.,0.118647888893132,0.992936391951268));
#21253=DIRECTION('center_axis',(0.,0.992936391951269,-0.118647888893132));
#21254=DIRECTION('ref_axis',(0.,0.118647888893132,0.992936391951268));
#21255=DIRECTION('',(1.,0.,0.));
#21256=DIRECTION('',(0.,0.118647888893132,0.992936391951268));
#21257=DIRECTION('center_axis',(1.,0.,0.));
#21258=DIRECTION('ref_axis',(0.,0.743144825477394,0.669130606358858));
#21259=DIRECTION('center_axis',(1.,0.,0.));
#21260=DIRECTION('ref_axis',(0.,1.,0.));
#21261=DIRECTION('center_axis',(0.,-0.19399337156981,-0.981002839846541));
#21262=DIRECTION('ref_axis',(0.,0.981002839846541,-0.19399337156981));
#21263=DIRECTION('',(-1.,0.,0.));
#21264=DIRECTION('',(0.,0.981002839846541,-0.19399337156981));
#21265=DIRECTION('',(1.,0.,0.));
#21266=DIRECTION('',(0.,0.981002839846541,-0.19399337156981));
#21267=DIRECTION('center_axis',(1.,0.,0.));
#21268=DIRECTION('ref_axis',(0.,0.866025403784439,0.5));
#21269=DIRECTION('center_axis',(-1.,0.,0.));
#21270=DIRECTION('ref_axis',(0.,1.,0.));
#21271=DIRECTION('',(0.,0.322498231978021,0.946570066276686));
#21272=DIRECTION('center_axis',(0.,0.946570066276686,-0.322498231978021));
#21273=DIRECTION('ref_axis',(0.,0.322498231978021,0.946570066276686));
#21274=DIRECTION('',(1.,0.,0.));
#21275=DIRECTION('',(0.,0.322498231978021,0.946570066276686));
#21276=DIRECTION('center_axis',(1.,0.,0.));
#21277=DIRECTION('ref_axis',(0.,0.866025403784439,0.5));
#21278=DIRECTION('center_axis',(1.,0.,0.));
#21279=DIRECTION('ref_axis',(0.,1.,0.));
#21280=DIRECTION('center_axis',(0.,-0.393716110088789,-0.919232084218427));
#21281=DIRECTION('ref_axis',(0.,0.919232084218427,-0.393716110088789));
#21282=DIRECTION('',(-1.,0.,0.));
#21283=DIRECTION('',(0.,0.919232084218427,-0.393716110088789));
#21284=DIRECTION('',(1.,0.,0.));
#21285=DIRECTION('',(0.,0.919232084218427,-0.393716110088789));
#21286=DIRECTION('center_axis',(1.,0.,0.));
#21287=DIRECTION('ref_axis',(0.,0.951056516295154,0.309016994374947));
#21288=DIRECTION('center_axis',(-1.,0.,0.));
#21289=DIRECTION('ref_axis',(0.,1.,0.));
#21290=DIRECTION('',(0.,0.51225385480726,0.858834086558692));
#21291=DIRECTION('center_axis',(0.,0.858834086558692,-0.51225385480726));
#21292=DIRECTION('ref_axis',(0.,0.51225385480726,0.858834086558692));
#21293=DIRECTION('',(1.,0.,0.));
#21294=DIRECTION('',(0.,0.51225385480726,0.858834086558692));
#21295=DIRECTION('center_axis',(1.,0.,0.));
#21296=DIRECTION('ref_axis',(0.,0.951056516295154,0.309016994374947));
#21297=DIRECTION('center_axis',(1.,0.,0.));
#21298=DIRECTION('ref_axis',(0.,1.,0.));
#21299=DIRECTION('center_axis',(0.,-0.576231565337382,-0.817286475545038));
#21300=DIRECTION('ref_axis',(0.,0.817286475545038,-0.576231565337382));
#21301=DIRECTION('',(-1.,0.,0.));
#21302=DIRECTION('',(0.,0.817286475545038,-0.576231565337382));
#21303=DIRECTION('',(1.,0.,0.));
#21304=DIRECTION('',(0.,0.817286475545038,-0.576231565337382));
#21305=DIRECTION('center_axis',(1.,0.,0.));
#21306=DIRECTION('ref_axis',(0.,0.994521895368273,0.104528463267653));
#21307=DIRECTION('center_axis',(-1.,0.,0.));
#21308=DIRECTION('ref_axis',(0.,1.,0.));
#21309=DIRECTION('',(0.,0.679621526114708,0.733562936114901));
#21310=DIRECTION('center_axis',(0.,0.733562936114902,-0.679621526114708));
#21311=DIRECTION('ref_axis',(0.,0.679621526114708,0.733562936114901));
#21312=DIRECTION('',(1.,0.,0.));
#21313=DIRECTION('',(0.,0.679621526114708,0.733562936114901));
#21314=DIRECTION('center_axis',(1.,0.,0.));
#21315=DIRECTION('ref_axis',(0.,0.994521895368273,0.104528463267653));
#21316=DIRECTION('center_axis',(1.,0.,0.));
#21317=DIRECTION('ref_axis',(0.,1.,0.));
#21318=DIRECTION('center_axis',(0.,-0.733562936114902,-0.679621526114708));
#21319=DIRECTION('ref_axis',(0.,0.679621526114708,-0.733562936114902));
#21320=DIRECTION('',(-1.,0.,0.));
#21321=DIRECTION('',(0.,0.679621526114708,-0.733562936114902));
#21322=DIRECTION('',(1.,0.,0.));
#21323=DIRECTION('',(0.,0.679621526114708,-0.733562936114902));
#21324=DIRECTION('center_axis',(1.,0.,0.));
#21325=DIRECTION('ref_axis',(0.,0.994521895368273,-0.104528463267654));
#21326=DIRECTION('center_axis',(-1.,0.,0.));
#21327=DIRECTION('ref_axis',(0.,1.,0.));
#21328=DIRECTION('',(0.,0.817286475545038,0.576231565337382));
#21329=DIRECTION('center_axis',(0.,0.576231565337382,-0.817286475545039));
#21330=DIRECTION('ref_axis',(0.,0.817286475545038,0.576231565337382));
#21331=DIRECTION('',(1.,0.,0.));
#21332=DIRECTION('',(0.,0.817286475545038,0.576231565337382));
#21333=DIRECTION('center_axis',(1.,0.,0.));
#21334=DIRECTION('ref_axis',(0.,0.994521895368273,-0.104528463267654));
#21335=DIRECTION('center_axis',(1.,0.,0.));
#21336=DIRECTION('ref_axis',(0.,1.,0.));
#21337=DIRECTION('center_axis',(0.,-0.858834086558692,-0.51225385480726));
#21338=DIRECTION('ref_axis',(0.,0.51225385480726,-0.858834086558692));
#21339=DIRECTION('',(-1.,0.,0.));
#21340=DIRECTION('',(0.,0.51225385480726,-0.858834086558692));
#21341=DIRECTION('',(1.,0.,0.));
#21342=DIRECTION('',(0.,0.51225385480726,-0.858834086558692));
#21343=DIRECTION('center_axis',(1.,0.,0.));
#21344=DIRECTION('ref_axis',(0.,0.951056516295154,-0.309016994374948));
#21345=DIRECTION('center_axis',(-1.,0.,0.));
#21346=DIRECTION('ref_axis',(0.,1.,0.));
#21347=DIRECTION('',(0.,0.919232084218427,0.393716110088789));
#21348=DIRECTION('center_axis',(0.,0.393716110088789,-0.919232084218427));
#21349=DIRECTION('ref_axis',(0.,0.919232084218427,0.393716110088789));
#21350=DIRECTION('',(1.,0.,0.));
#21351=DIRECTION('',(0.,0.919232084218427,0.393716110088789));
#21352=DIRECTION('center_axis',(1.,0.,0.));
#21353=DIRECTION('ref_axis',(0.,0.951056516295154,-0.309016994374948));
#21354=DIRECTION('center_axis',(1.,0.,0.));
#21355=DIRECTION('ref_axis',(0.,1.,0.));
#21356=DIRECTION('center_axis',(0.,-0.946570066276686,-0.322498231978021));
#21357=DIRECTION('ref_axis',(0.,0.322498231978021,-0.946570066276686));
#21358=DIRECTION('',(-1.,0.,0.));
#21359=DIRECTION('',(0.,0.322498231978021,-0.946570066276686));
#21360=DIRECTION('',(1.,0.,0.));
#21361=DIRECTION('',(0.,0.322498231978021,-0.946570066276686));
#21362=DIRECTION('center_axis',(1.,0.,0.));
#21363=DIRECTION('ref_axis',(0.,0.866025403784439,-0.5));
#21364=DIRECTION('center_axis',(-1.,0.,0.));
#21365=DIRECTION('ref_axis',(0.,1.,0.));
#21366=DIRECTION('',(0.,0.981002839846541,0.19399337156981));
#21367=DIRECTION('center_axis',(0.,0.19399337156981,-0.981002839846541));
#21368=DIRECTION('ref_axis',(0.,0.981002839846541,0.19399337156981));
#21369=DIRECTION('',(1.,0.,0.));
#21370=DIRECTION('',(0.,0.981002839846541,0.19399337156981));
#21371=DIRECTION('center_axis',(1.,0.,0.));
#21372=DIRECTION('ref_axis',(0.,0.866025403784439,-0.5));
#21373=DIRECTION('center_axis',(1.,0.,0.));
#21374=DIRECTION('ref_axis',(0.,1.,0.));
#21375=DIRECTION('center_axis',(0.,-0.992936391951269,-0.118647888893131));
#21376=DIRECTION('ref_axis',(0.,0.118647888893131,-0.992936391951268));
#21377=DIRECTION('',(-1.,0.,0.));
#21378=DIRECTION('',(0.,0.118647888893131,-0.992936391951268));
#21379=DIRECTION('',(1.,0.,0.));
#21380=DIRECTION('',(0.,0.118647888893131,-0.992936391951268));
#21381=DIRECTION('center_axis',(1.,0.,0.));
#21382=DIRECTION('ref_axis',(0.,0.743144825477394,-0.669130606358858));
#21383=DIRECTION('center_axis',(-1.,0.,0.));
#21384=DIRECTION('ref_axis',(0.,1.,0.));
#21385=DIRECTION('',(0.,0.999899063999461,-0.0142078081702469));
#21386=DIRECTION('center_axis',(0.,-0.0142078081702469,-0.999899063999461));
#21387=DIRECTION('ref_axis',(0.,0.999899063999461,-0.0142078081702469));
#21388=DIRECTION('',(1.,0.,0.));
#21389=DIRECTION('',(0.,0.999899063999461,-0.0142078081702469));
#21390=DIRECTION('center_axis',(1.,0.,0.));
#21391=DIRECTION('ref_axis',(0.,0.743144825477394,-0.669130606358858));
#21392=DIRECTION('center_axis',(1.,0.,0.));
#21393=DIRECTION('ref_axis',(0.,1.,0.));
#21394=DIRECTION('center_axis',(0.,-0.995906632660144,0.0903879362721262));
#21395=DIRECTION('ref_axis',(0.,-0.0903879362721261,-0.995906632660144));
#21396=DIRECTION('',(-1.,0.,0.));
#21397=DIRECTION('',(0.,-0.0903879362721261,-0.995906632660144));
#21398=DIRECTION('',(1.,0.,0.));
#21399=DIRECTION('',(0.,-0.0903879362721261,-0.995906632660144));
#21400=DIRECTION('center_axis',(1.,0.,0.));
#21401=DIRECTION('ref_axis',(0.,0.587785252292473,-0.809016994374947));
#21402=DIRECTION('center_axis',(-1.,0.,0.));
#21403=DIRECTION('ref_axis',(0.,1.,0.));
#21404=DIRECTION('',(0.,0.97509490100756,-0.221788038516636));
#21405=DIRECTION('center_axis',(0.,-0.221788038516636,-0.97509490100756));
#21406=DIRECTION('ref_axis',(0.,0.97509490100756,-0.221788038516636));
#21407=DIRECTION('',(1.,0.,0.));
#21408=DIRECTION('',(0.,0.97509490100756,-0.221788038516636));
#21409=DIRECTION('center_axis',(1.,0.,0.));
#21410=DIRECTION('ref_axis',(0.,0.587785252292473,-0.809016994374947));
#21411=DIRECTION('center_axis',(1.,0.,0.));
#21412=DIRECTION('ref_axis',(0.,1.,0.));
#21413=DIRECTION('center_axis',(0.,-0.955350974631537,0.295473374892852));
#21414=DIRECTION('ref_axis',(0.,-0.295473374892852,-0.955350974631537));
#21415=DIRECTION('',(-1.,0.,0.));
#21416=DIRECTION('',(0.,-0.295473374892852,-0.955350974631537));
#21417=DIRECTION('',(1.,0.,0.));
#21418=DIRECTION('',(0.,-0.295473374892852,-0.955350974631537));
#21419=DIRECTION('center_axis',(1.,0.,0.));
#21420=DIRECTION('ref_axis',(0.,0.4067366430758,-0.913545457642601));
#21421=DIRECTION('center_axis',(-1.,0.,0.));
#21422=DIRECTION('ref_axis',(0.,1.,0.));
#21423=DIRECTION('',(0.,0.907674411817164,-0.419675067322762));
#21424=DIRECTION('center_axis',(0.,-0.419675067322762,-0.907674411817164));
#21425=DIRECTION('ref_axis',(0.,0.907674411817164,-0.419675067322762));
#21426=DIRECTION('',(1.,0.,0.));
#21427=DIRECTION('',(0.,0.907674411817164,-0.419675067322762));
#21428=DIRECTION('center_axis',(1.,0.,0.));
#21429=DIRECTION('ref_axis',(0.,0.4067366430758,-0.913545457642601));
#21430=DIRECTION('center_axis',(1.,0.,0.));
#21431=DIRECTION('ref_axis',(0.,1.,0.));
#21432=DIRECTION('center_axis',(0.,-0.873041894728939,0.487645209192201));
#21433=DIRECTION('ref_axis',(0.,-0.487645209192201,-0.873041894728939));
#21434=DIRECTION('',(-1.,0.,0.));
#21435=DIRECTION('',(0.,-0.487645209192201,-0.873041894728939));
#21436=DIRECTION('',(1.,0.,0.));
#21437=DIRECTION('',(0.,-0.487645209192201,-0.873041894728939));
#21438=DIRECTION('center_axis',(1.,0.,0.));
#21439=DIRECTION('ref_axis',(0.,0.207911690817759,-0.978147600733806));
#21440=DIRECTION('center_axis',(-1.,0.,0.));
#21441=DIRECTION('ref_axis',(0.,1.,0.));
#21442=DIRECTION('',(0.,0.800584195325295,-0.59922028186248));
#21443=DIRECTION('center_axis',(0.,-0.59922028186248,-0.800584195325295));
#21444=DIRECTION('ref_axis',(0.,0.800584195325295,-0.59922028186248));
#21445=DIRECTION('',(1.,0.,0.));
#21446=DIRECTION('',(0.,0.800584195325295,-0.59922028186248));
#21447=DIRECTION('center_axis',(1.,0.,0.));
#21448=DIRECTION('ref_axis',(0.,0.207911690817759,-0.978147600733806));
#21449=DIRECTION('center_axis',(1.,0.,0.));
#21450=DIRECTION('ref_axis',(0.,1.,0.));
#21451=DIRECTION('center_axis',(0.,-0.752576694706877,0.65850460786852));
#21452=DIRECTION('ref_axis',(0.,-0.65850460786852,-0.752576694706877));
#21453=DIRECTION('',(-1.,0.,0.));
#21454=DIRECTION('',(0.,-0.65850460786852,-0.752576694706877));
#21455=DIRECTION('',(1.,0.,0.));
#21456=DIRECTION('',(0.,-0.65850460786852,-0.752576694706877));
#21457=DIRECTION('center_axis',(1.,0.,0.));
#21458=DIRECTION('ref_axis',(0.,0.,-1.));
#21459=DIRECTION('center_axis',(-1.,0.,0.));
#21460=DIRECTION('ref_axis',(0.,1.,0.));
#21461=DIRECTION('',(0.,0.65850460786852,-0.752576694706877));
#21462=DIRECTION('center_axis',(0.,-0.752576694706877,-0.65850460786852));
#21463=DIRECTION('ref_axis',(0.,0.65850460786852,-0.752576694706877));
#21464=DIRECTION('',(1.,0.,0.));
#21465=DIRECTION('',(0.,0.65850460786852,-0.752576694706877));
#21466=DIRECTION('center_axis',(1.,0.,0.));
#21467=DIRECTION('ref_axis',(0.,0.,-1.));
#21468=DIRECTION('center_axis',(1.,0.,0.));
#21469=DIRECTION('ref_axis',(0.,1.,0.));
#21470=DIRECTION('center_axis',(-1.,0.,0.));
#21471=DIRECTION('ref_axis',(0.,0.,1.));
#21472=DIRECTION('center_axis',(1.,0.,0.));
#21473=DIRECTION('ref_axis',(0.,0.,-1.));
#21474=DIRECTION('center_axis',(1.,0.,0.));
#21475=DIRECTION('ref_axis',(0.,1.,0.));
#21476=DIRECTION('center_axis',(1.,0.,0.));
#21477=DIRECTION('ref_axis',(0.,0.,-1.));
#21478=DIRECTION('',(-0.554700196225229,0.832050294337844,1.01896772969045E-16));
#21479=DIRECTION('center_axis',(1.,0.,0.));
#21480=DIRECTION('ref_axis',(0.,1.,0.));
#21481=DIRECTION('',(-0.707106781186547,0.707106781186548,8.65956056235493E-17));
#21482=DIRECTION('center_axis',(1.,0.,0.));
#21483=DIRECTION('ref_axis',(0.,-0.367056220099871,-0.93019875902196));
#21484=DIRECTION('center_axis',(1.,0.,0.));
#21485=DIRECTION('ref_axis',(0.,1.,0.));
#21486=DIRECTION('center_axis',(1.,0.,0.));
#21487=DIRECTION('ref_axis',(0.,0.,-1.));
#21488=DIRECTION('',(-1.,0.,0.));
#21489=DIRECTION('center_axis',(-1.,0.,0.));
#21490=DIRECTION('ref_axis',(0.,0.,1.));
#21491=DIRECTION('center_axis',(1.,0.,0.));
#21492=DIRECTION('ref_axis',(0.,0.,-1.));
#21493=DIRECTION('center_axis',(1.,0.,0.));
#21494=DIRECTION('ref_axis',(0.,1.,0.));
#21495=DIRECTION('center_axis',(1.,0.,0.));
#21496=DIRECTION('ref_axis',(0.,0.,-1.));
#21497=DIRECTION('',(-0.707106781186549,0.707106781186546,8.65956056235492E-17));
#21498=DIRECTION('center_axis',(1.,0.,0.));
#21499=DIRECTION('ref_axis',(0.,1.,0.));
#21500=DIRECTION('center_axis',(1.,0.,0.));
#21501=DIRECTION('ref_axis',(0.,0.,-1.));
#21502=DIRECTION('',(-1.,0.,0.));
#21503=DIRECTION('',(-1.,0.,0.));
#21504=DIRECTION('center_axis',(-1.,0.,0.));
#21505=DIRECTION('ref_axis',(0.,1.,0.));
#21506=DIRECTION('center_axis',(1.,0.,0.));
#21507=DIRECTION('ref_axis',(0.,0.,-1.));
#21508=DIRECTION('',(-0.707106781186548,-0.707106781186548,-8.65956056235493E-17));
#21509=DIRECTION('center_axis',(1.,0.,0.));
#21510=DIRECTION('ref_axis',(0.,0.,-1.));
#40639=CARTESIAN_POINT('',(0.,0.,0.));
#40640=CARTESIAN_POINT('Origin',(8.75,0.,0.));
#40641=CARTESIAN_POINT('',(2.76432045465689,-4.94788959559308,0.00239028935128519));
#40642=CARTESIAN_POINT('',(2.6196795453431,-4.94443125321576,0.00146311145371448));
#40643=CARTESIAN_POINT('',(8.75,-4.942,-6.05220448138622E-16));
#40644=CARTESIAN_POINT('',(2.442,2.17246025283987,4.44279282409917));
#40645=CARTESIAN_POINT('Ctrl Pts',(2.76432045465689,-4.94788959559308,0.00239028935128519));
#40646=CARTESIAN_POINT('Ctrl Pts',(2.75931691497812,-4.94892132323628,0.157204467377098));
#40647=CARTESIAN_POINT('Ctrl Pts',(2.75431337529936,-4.94231374587349,0.311936106973573));
#40648=CARTESIAN_POINT('Ctrl Pts',(2.74930983562059,-4.9277840870703,0.465924016286531));
#40649=CARTESIAN_POINT('Ctrl Pts',(2.6962765448657,-4.7737819866876,2.09806567831472));
#40650=CARTESIAN_POINT('Ctrl Pts',(2.6432432541108,-3.72979678823222,3.64665513416632));
#40651=CARTESIAN_POINT('Ctrl Pts',(2.59020996335591,-2.27271757376403,4.39850416463932));
#40652=CARTESIAN_POINT('Ctrl Pts',(2.54080664223727,-0.915371059847599,
5.09889138475105));
#40653=CARTESIAN_POINT('Ctrl Pts',(2.49140332111864,0.80045472016787,5.10787444045995));
#40654=CARTESIAN_POINT('Ctrl Pts',(2.442,2.17574915139364,4.44508346536535));
#40655=CARTESIAN_POINT('',(2.442,-2.16917135428613,4.44050218283298));
#40656=CARTESIAN_POINT('Origin',(2.442,0.,0.));
#40657=CARTESIAN_POINT('Ctrl Pts',(2.442,-2.16917135428612,4.44050218283299));
#40658=CARTESIAN_POINT('Ctrl Pts',(2.46851664537745,-2.9089989675068,4.07909871997413));
#40659=CARTESIAN_POINT('Ctrl Pts',(2.49503329075489,-3.55111543888009,3.52928885898635));
#40660=CARTESIAN_POINT('Ctrl Pts',(2.52154993613233,-4.02901758456164,2.85775650263327));
#40661=CARTESIAN_POINT('Ctrl Pts',(2.54806658150978,-4.5069197302432,2.18622414628017));
#40662=CARTESIAN_POINT('Ctrl Pts',(2.57458322688722,-4.82060755023301,1.39296929456177));
#40663=CARTESIAN_POINT('Ctrl Pts',(2.60109987226467,-4.91429750933697,0.576285982800623));
#40664=CARTESIAN_POINT('Ctrl Pts',(2.60729309662415,-4.93617972440233,0.385541531216247));
#40665=CARTESIAN_POINT('Ctrl Pts',(2.61348632098362,-4.94606100888929,0.193519052102877));
#40666=CARTESIAN_POINT('Ctrl Pts',(2.6196795453431,-4.94443125321576,0.00146311145371448));
#40667=CARTESIAN_POINT('Origin',(8.75,0.,0.));
#40668=CARTESIAN_POINT('',(3.76432045465689,-4.93571920292385,0.00301700625176843));
#40669=CARTESIAN_POINT('',(3.6196795453431,-4.93504902497496,0.00248727919068638));
#40670=CARTESIAN_POINT('',(8.75,-4.942,-6.05220448138622E-16));
#40671=CARTESIAN_POINT('Ctrl Pts',(3.76432045465689,-4.93571920292385,0.00301700625176843));
#40672=CARTESIAN_POINT('Ctrl Pts',(3.74418332617413,-4.9392039814057,0.630130822225083));
#40673=CARTESIAN_POINT('Ctrl Pts',(3.72404619769136,-4.82845404842863,1.25605983210146));
#40674=CARTESIAN_POINT('Ctrl Pts',(3.70390906920859,-4.59783645110691,1.83417191416958));
#40675=CARTESIAN_POINT('Ctrl Pts',(3.6508757784537,-3.99048023830714,3.3566921763544));
#40676=CARTESIAN_POINT('Ctrl Pts',(3.59784248769881,-2.55173533303798,4.54755958365334));
#40677=CARTESIAN_POINT('Ctrl Pts',(3.54480919694392,-0.942516547825695,
4.85964727579633));
#40678=CARTESIAN_POINT('Ctrl Pts',(3.49177590618903,0.666702237386595,5.17173496793932));
#40679=CARTESIAN_POINT('Ctrl Pts',(3.43874261543414,2.44639490254201,4.60504294492635));
#40680=CARTESIAN_POINT('Ctrl Pts',(3.38570932467925,3.5788553706631,3.41997949552812));
#40681=CARTESIAN_POINT('Ctrl Pts',(3.33267603392436,4.71131583878419,2.23491604612988));
#40682=CARTESIAN_POINT('Ctrl Pts',(3.27964274316948,5.19654410987096,0.431481170346373));
#40683=CARTESIAN_POINT('Ctrl Pts',(3.22660945241459,4.8118217284371,-1.16194233954266));
#40684=CARTESIAN_POINT('Ctrl Pts',(3.1735761616597,4.42709934700323,-2.7553658494317));
#40685=CARTESIAN_POINT('Ctrl Pts',(3.12054287090481,3.17242631304874,-4.13877799342627));
#40686=CARTESIAN_POINT('Ctrl Pts',(3.06750958014992,1.62382688421027,-4.67638660621195));
#40687=CARTESIAN_POINT('Ctrl Pts',(3.01447628939503,0.0752274553718063,
-5.21399521899763));
#40688=CARTESIAN_POINT('Ctrl Pts',(2.96144299864014,-1.76729836835063,-4.90580030057443));
#40689=CARTESIAN_POINT('Ctrl Pts',(2.90840970788525,-3.05655177905683,-3.89385590726044));
#40690=CARTESIAN_POINT('Ctrl Pts',(2.86037995680913,-4.22416780870228,-2.97738558037873));
#40691=CARTESIAN_POINT('Ctrl Pts',(2.81235020573301,-4.93798588240953,-1.48369494450495));
#40692=CARTESIAN_POINT('Ctrl Pts',(2.76432045465689,-4.94788959559308,0.00239028935128519));
#40693=CARTESIAN_POINT('Ctrl Pts',(2.6196795453431,-4.94443125321576,0.00146311145371448));
#40694=CARTESIAN_POINT('Ctrl Pts',(2.66651961173851,-4.93210522407074,-1.45107800275172));
#40695=CARTESIAN_POINT('Ctrl Pts',(2.71335967813392,-4.26133958869745,-2.90553314037676));
#40696=CARTESIAN_POINT('Ctrl Pts',(2.76019974452934,-3.14406853058354,-3.82348377368421));
#40697=CARTESIAN_POINT('Ctrl Pts',(2.81323303528422,-1.87907115895764,-4.86280644295348));
#40698=CARTESIAN_POINT('Ctrl Pts',(2.86626632603911,-0.0416879410413212,
-5.21437131779874));
#40699=CARTESIAN_POINT('Ctrl Pts',(2.919299616794,1.51912370630509,-4.71214944827796));
#40700=CARTESIAN_POINT('Ctrl Pts',(2.97233290754889,3.0799353536515,-4.20992757875717));
#40701=CARTESIAN_POINT('Ctrl Pts',(3.02536619830378,4.364175430428,-2.85391896487034));
#40702=CARTESIAN_POINT('Ctrl Pts',(3.07839948905867,4.78425699578354,-1.26926289529364));
#40703=CARTESIAN_POINT('Ctrl Pts',(3.13143277981356,5.20433856113907,0.315393174283052));
#40704=CARTESIAN_POINT('Ctrl Pts',(3.18446607056845,4.76026161507364,2.12869669954961));
#40705=CARTESIAN_POINT('Ctrl Pts',(3.23749936132334,3.6548001293483,3.33872180443716));
#40706=CARTESIAN_POINT('Ctrl Pts',(3.29053265207823,2.54933864362295,4.54874690932471));
#40707=CARTESIAN_POINT('Ctrl Pts',(3.34356594283312,0.782492618237691,5.15549359383325));
#40708=CARTESIAN_POINT('Ctrl Pts',(3.39659923358801,-0.833393310877007,
4.87963769585482));
#40709=CARTESIAN_POINT('Ctrl Pts',(3.4496325243429,-2.44927923999171,4.60378179787639));
#40710=CARTESIAN_POINT('Ctrl Pts',(3.50266581509778,-3.91420507283584,3.44532331741098));
#40711=CARTESIAN_POINT('Ctrl Pts',(3.55569910585267,-4.55550993645389,1.93676831562686));
#40712=CARTESIAN_POINT('Ctrl Pts',(3.57702591901615,-4.81340434226065,1.33011784736587));
#40713=CARTESIAN_POINT('Ctrl Pts',(3.59835273217962,-4.93810551184841,0.666850937312143));
#40714=CARTESIAN_POINT('Ctrl Pts',(3.6196795453431,-4.93504902497496,0.00248727919068638));
#40715=CARTESIAN_POINT('Origin',(8.75,0.,0.));
#40716=CARTESIAN_POINT('',(4.76432045465689,-4.93730273339884,-0.00383068200619119));
#40717=CARTESIAN_POINT('',(4.61967954534309,-4.93822978717952,-0.00413487577884502));
#40718=CARTESIAN_POINT('',(8.75,-4.942,-6.05220448138622E-16));
#40719=CARTESIAN_POINT('Ctrl Pts',(4.76432045465689,-4.93730273339884,-0.00383068200619119));
#40720=CARTESIAN_POINT('Ctrl Pts',(4.72904973737013,-4.92940489017672,1.09369834277235));
#40721=CARTESIAN_POINT('Ctrl Pts',(4.69377902008336,-4.56844519037125,2.1959421476368));
#40722=CARTESIAN_POINT('Ctrl Pts',(4.6585083027966,-3.89588421868249,3.05392627541324));
#40723=CARTESIAN_POINT('Ctrl Pts',(4.60547501204171,-2.88461696057815,4.34399705399991));
#40724=CARTESIAN_POINT('Ctrl Pts',(4.55244172128681,-1.16887112604092,5.08183738578865));
#40725=CARTESIAN_POINT('Ctrl Pts',(4.49940843053193,0.463129480941426,4.92847788550683));
#40726=CARTESIAN_POINT('Ctrl Pts',(4.44637513977704,2.09513008792377,4.77511838522502));
#40727=CARTESIAN_POINT('Ctrl Pts',(4.39334184902215,3.64338546735125,3.73055905287266));
#40728=CARTESIAN_POINT('Ctrl Pts',(4.34030855826726,4.39661485369635,2.27467863331172));
#40729=CARTESIAN_POINT('Ctrl Pts',(4.28727526751237,5.14984424004146,0.818798213750785));
#40730=CARTESIAN_POINT('Ctrl Pts',(4.23424197675748,5.10804763330419,-1.04840329301873));
#40731=CARTESIAN_POINT('Ctrl Pts',(4.18120868600259,4.29043066949209,-2.46912382375875));
#40732=CARTESIAN_POINT('Ctrl Pts',(4.1281753952477,3.47281370567999,-3.88984435449878));
#40733=CARTESIAN_POINT('Ctrl Pts',(4.07514210449281,1.87937638479307,-4.8640839092093));
#40734=CARTESIAN_POINT('Ctrl Pts',(4.02210881373792,0.242146596270669,-4.94426553960403));
#40735=CARTESIAN_POINT('Ctrl Pts',(3.96907552298303,-1.39508319225173,-5.02444716999875));
#40736=CARTESIAN_POINT('Ctrl Pts',(3.91604223222815,-3.07610544840959,-4.21057087607769));
#40737=CARTESIAN_POINT('Ctrl Pts',(3.86300894147326,-4.02863281632334,-2.87654617058181));
#40738=CARTESIAN_POINT('Ctrl Pts',(3.83011277920114,-4.61947857410121,-2.04906040527569));
#40739=CARTESIAN_POINT('Ctrl Pts',(3.79721661692902,-4.93002644297949,-1.02144076939389));
#40740=CARTESIAN_POINT('Ctrl Pts',(3.76432045465689,-4.93571920292385,0.00301700625176843));
#40741=CARTESIAN_POINT('Ctrl Pts',(3.6196795453431,-4.93504902497496,0.00248727919068638));
#40742=CARTESIAN_POINT('Ctrl Pts',(3.65138602293451,-4.93050495963249,-0.985219195157505));
#40743=CARTESIAN_POINT('Ctrl Pts',(3.68309250052593,-4.6435828004328,-1.97534977180522));
#40744=CARTESIAN_POINT('Ctrl Pts',(3.71479897811734,-4.09214380238604,-2.78546735077523));
#40745=CARTESIAN_POINT('Ctrl Pts',(3.76783226887223,-3.16978891030818,-4.14049649229039));
#40746=CARTESIAN_POINT('Ctrl Pts',(3.82086555962712,-1.50739523176048,-4.99190325221787));
#40747=CARTESIAN_POINT('Ctrl Pts',(3.87389885038201,0.131231392969287,-4.9484634883131));
#40748=CARTESIAN_POINT('Ctrl Pts',(3.9269321411369,1.76985801769906,-4.90502372440833));
#40749=CARTESIAN_POINT('Ctrl Pts',(3.97996543189179,3.38471758861089,-3.96673743667131));
#40750=CARTESIAN_POINT('Ctrl Pts',(4.03299872264668,4.2339806263878,-2.56470241627798));
#40751=CARTESIAN_POINT('Ctrl Pts',(4.08603201340157,5.0832436641647,-1.16266739588466));
#40752=CARTESIAN_POINT('Ctrl Pts',(4.13906530415646,5.16691016880668,0.703116357164973));
#40753=CARTESIAN_POINT('Ctrl Pts',(4.19209859491135,4.44651837456859,2.17551792657388));
#40754=CARTESIAN_POINT('Ctrl Pts',(4.24513188566624,3.7261265803305,3.64791949598279));
#40755=CARTESIAN_POINT('Ctrl Pts',(4.29816517642112,2.20167648721235,4.72693888175098));
#40756=CARTESIAN_POINT('Ctrl Pts',(4.35119846717601,0.573523415343645,4.91685582765776));
#40757=CARTESIAN_POINT('Ctrl Pts',(4.4042317579309,-1.05462965652506,5.10677277356454));
#40758=CARTESIAN_POINT('Ctrl Pts',(4.45726504868579,-2.78648570714431,4.40758727960991));
#40759=CARTESIAN_POINT('Ctrl Pts',(4.51029833944068,-3.82642545649684,3.14051583547344));
#40760=CARTESIAN_POINT('Ctrl Pts',(4.54675874140815,-4.54138431995091,2.26940386943988));
#40761=CARTESIAN_POINT('Ctrl Pts',(4.58321914337562,-4.92930435769488,1.12987684519085));
#40762=CARTESIAN_POINT('Ctrl Pts',(4.61967954534309,-4.93822978717952,-0.00413487577884502));
#40763=CARTESIAN_POINT('Origin',(8.75,0.,0.));
#40764=CARTESIAN_POINT('',(5.76432045465689,-4.94964305481555,-0.00149822017877888));
#40765=CARTESIAN_POINT('',(5.6196795453431,-4.95001972789837,-0.000833046281679996));
#40766=CARTESIAN_POINT('',(8.75,-4.942,-6.05220448138622E-16));
#40767=CARTESIAN_POINT('Ctrl Pts',(5.76432045465689,-4.94964305481555,-0.00149822017877888));
#40768=CARTESIAN_POINT('Ctrl Pts',(5.71391614856612,-4.94344322054585,1.55689473528395));
#40769=CARTESIAN_POINT('Ctrl Pts',(5.66351184247536,-4.14637927320866,3.12074849239652));
#40770=CARTESIAN_POINT('Ctrl Pts',(5.6131075363846,-2.87904405190479,4.02684576166472));
#40771=CARTESIAN_POINT('Ctrl Pts',(5.56007424562971,-1.54560723890131,4.98020319598355));
#40772=CARTESIAN_POINT('Ctrl Pts',(5.50704095487483,0.308436957536128,5.20540030448662));
#40773=CARTESIAN_POINT('Ctrl Pts',(5.45400766411994,1.83132849201121,4.59898004409288));
#40774=CARTESIAN_POINT('Ctrl Pts',(5.40097437336505,3.35422002648629,3.99255978369913));
#40775=CARTESIAN_POINT('Ctrl Pts',(5.34794108261015,4.54595889899902,2.55452215440856));
#40776=CARTESIAN_POINT('Ctrl Pts',(5.29490779185527,4.8590524110568,0.945511104271855));
#40777=CARTESIAN_POINT('Ctrl Pts',(5.24187450110038,5.17214592311458,-0.663499945864848));
#40778=CARTESIAN_POINT('Ctrl Pts',(5.18884121034549,4.60659407471741,-2.44348441684768));
#40779=CARTESIAN_POINT('Ctrl Pts',(5.1358079195906,3.42221517592476,-3.57670581664182));
#40780=CARTESIAN_POINT('Ctrl Pts',(5.08277462883571,2.23783627713212,-4.70992721643594));
#40781=CARTESIAN_POINT('Ctrl Pts',(5.02974133808082,0.434630327943992,-5.19638554504138));
#40782=CARTESIAN_POINT('Ctrl Pts',(4.97670804732593,-1.15899818313101,-4.81259855606007));
#40783=CARTESIAN_POINT('Ctrl Pts',(4.92367475657104,-2.75262669420602,-4.42881156707877));
#40784=CARTESIAN_POINT('Ctrl Pts',(4.87064146581615,-4.1366777671679,-3.17477926051071));
#40785=CARTESIAN_POINT('Ctrl Pts',(4.81760817506126,-4.67530896281311,-1.62661249453437));
#40786=CARTESIAN_POINT('Ctrl Pts',(4.79984560159314,-4.85571406399927,-1.10808110547425));
#40787=CARTESIAN_POINT('Ctrl Pts',(4.78208302812502,-4.94128014104076,-0.556553774579704));
#40788=CARTESIAN_POINT('Ctrl Pts',(4.76432045465689,-4.93730273339884,-0.00383068200619119));
#40789=CARTESIAN_POINT('Ctrl Pts',(4.61967954534309,-4.93822978717952,-0.00413487577884502));
#40790=CARTESIAN_POINT('Ctrl Pts',(4.63625243413051,-4.94228679539246,-0.519594089641197));
#40791=CARTESIAN_POINT('Ctrl Pts',(4.65282532291793,-4.86803933279054,-1.03391378094767));
#40792=CARTESIAN_POINT('Ctrl Pts',(4.66939821170535,-4.71060802454418,-1.5213680565377));
#40793=CARTESIAN_POINT('Ctrl Pts',(4.72243150246023,-4.20682739515321,-3.08122311009404));
#40794=CARTESIAN_POINT('Ctrl Pts',(4.77546479321513,-2.8512426882855,-4.36597582288839));
#40795=CARTESIAN_POINT('Ctrl Pts',(4.82849808397002,-1.26662024780191,-4.78540071462561));
#40796=CARTESIAN_POINT('Ctrl Pts',(4.88153137472491,0.318002192681684,-5.20482560636284));
#40797=CARTESIAN_POINT('Ctrl Pts',(4.9345646654798,2.13166236678116,-4.7589226770429));
#40798=CARTESIAN_POINT('Ctrl Pts',(4.98759795623469,3.34115384955769,-3.65254352104788));
#40799=CARTESIAN_POINT('Ctrl Pts',(5.04063124698957,4.55064533233423,-2.54616436505285));
#40800=CARTESIAN_POINT('Ctrl Pts',(5.09366453774446,5.15596812378785,-0.77930898238273));
#40801=CARTESIAN_POINT('Ctrl Pts',(5.14669782849935,4.87903246291005,0.83631812290041));
#40802=CARTESIAN_POINT('Ctrl Pts',(5.19973111925424,4.60209680203225,2.45194522818355));
#40803=CARTESIAN_POINT('Ctrl Pts',(5.25276441000913,3.44290268882303,3.91634405607971));
#40804=CARTESIAN_POINT('Ctrl Pts',(5.30579770076402,1.93399176423248,4.55675994305442));
#40805=CARTESIAN_POINT('Ctrl Pts',(5.35883099151891,0.425080839641918,5.19717583002913));
#40806=CARTESIAN_POINT('Ctrl Pts',(5.4118642822738,-1.43354689632998,5.01360877608239));
#40807=CARTESIAN_POINT('Ctrl Pts',(5.46489757302869,-2.78802580404174,4.09039081253591));
#40808=CARTESIAN_POINT('Ctrl Pts',(5.51649156380016,-4.10574475509872,3.19222857494401));
#40809=CARTESIAN_POINT('Ctrl Pts',(5.56808555457163,-4.94630829537066,1.5940182288886));
#40810=CARTESIAN_POINT('Ctrl Pts',(5.6196795453431,-4.95001972789837,-0.000833046281679996));
#40811=CARTESIAN_POINT('Origin',(8.75,0.,0.));
#40812=CARTESIAN_POINT('',(6.76432045465689,-4.94186257797741,0.00456669625063827));
#40813=CARTESIAN_POINT('',(6.6196795453431,-4.9407490012001,0.0045438707638676));
#40814=CARTESIAN_POINT('',(8.75,-4.942,-6.05220448138622E-16));
#40815=CARTESIAN_POINT('Ctrl Pts',(6.76432045465689,-4.94186257797741,0.00456669625063827));
#40816=CARTESIAN_POINT('Ctrl Pts',(6.75181585051702,-4.9454453112525,0.392766622957461));
#40817=CARTESIAN_POINT('Ctrl Pts',(6.73931124637715,-4.903575088203,0.780202475095632));
#40818=CARTESIAN_POINT('Ctrl Pts',(6.72680664223727,-4.81331559170814,1.15601664885576));
#40819=CARTESIAN_POINT('Ctrl Pts',(6.67377335148238,-4.4305159390795,2.74988256607248));
#40820=CARTESIAN_POINT('Ctrl Pts',(6.6207400607275,-3.17734138642797,4.13471006555375));
#40821=CARTESIAN_POINT('Ctrl Pts',(6.56770676997261,-1.62950854494116,4.67430030900523));
#40822=CARTESIAN_POINT('Ctrl Pts',(6.51467347921772,-0.0816757034543591,
5.2138905524567));
#40823=CARTESIAN_POINT('Ctrl Pts',(6.46164018846282,1.76081542686771,4.90824353987838));
#40824=CARTESIAN_POINT('Ctrl Pts',(6.40860689770793,3.05151233350821,3.89777551376765));
#40825=CARTESIAN_POINT('Ctrl Pts',(6.35557360695305,4.34220924014869,2.88730748765693));
#40826=CARTESIAN_POINT('Ctrl Pts',(6.30254031619816,5.08111192310762,1.17201844801381));
#40827=CARTESIAN_POINT('Ctrl Pts',(6.24950702544328,4.9287636414054,-0.460076566630388));
#40828=CARTESIAN_POINT('Ctrl Pts',(6.19647373468839,4.77641535970318,-2.0921715812746));
#40829=CARTESIAN_POINT('Ctrl Pts',(6.14344044393349,3.73281611333981,-3.64107257091991));
#40830=CARTESIAN_POINT('Ctrl Pts',(6.0904071531786,2.2774022442656,-4.39520426037522));
#40831=CARTESIAN_POINT('Ctrl Pts',(6.03737386242371,0.821988375191376,-5.14933594983054));
#40832=CARTESIAN_POINT('Ctrl Pts',(5.98434057166883,-1.04524011659369,-5.10869833909587));
#40833=CARTESIAN_POINT('Ctrl Pts',(5.93130728091394,-2.46646621509766,-4.29196061115554));
#40834=CARTESIAN_POINT('Ctrl Pts',(5.87827399015905,-3.8876923136016,-3.47522288321523));
#40835=CARTESIAN_POINT('Ctrl Pts',(5.82524069940415,-4.86291601882446,-1.88238503806929));
#40836=CARTESIAN_POINT('Ctrl Pts',(5.77220740864926,-4.94411315665113,-0.245207235429026));
#40837=CARTESIAN_POINT('Ctrl Pts',(5.76957842398514,-4.94813828930043,-0.164048490151806));
#40838=CARTESIAN_POINT('Ctrl Pts',(5.76694943932101,-4.94996642538603,-0.0827807830855278));
#40839=CARTESIAN_POINT('Ctrl Pts',(5.76432045465689,-4.94964305481555,-0.00149822017877888));
#40840=CARTESIAN_POINT('Ctrl Pts',(5.6196795453431,-4.95001972789837,-0.000833046281679996));
#40841=CARTESIAN_POINT('Ctrl Pts',(5.62111884532652,-4.95012326446717,-0.0453240689683047));
#40842=CARTESIAN_POINT('Ctrl Pts',(5.62255814530994,-4.94957554297509,-0.0898124775466891));
#40843=CARTESIAN_POINT('Ctrl Pts',(5.62399744529335,-4.94836875446486,-0.134283001160447));
#40844=CARTESIAN_POINT('Ctrl Pts',(5.67703073604824,-4.90390271772459,-1.77286997816412));
#40845=CARTESIAN_POINT('Ctrl Pts',(5.73006402680313,-3.96464056479241,-3.38717505902524));
#40846=CARTESIAN_POINT('Ctrl Pts',(5.78309731755802,-2.5620855277057,-4.23557586562432));
#40847=CARTESIAN_POINT('Ctrl Pts',(5.83613060831291,-1.15953049061901,-5.08397667222339));
#40848=CARTESIAN_POINT('Ctrl Pts',(5.8891638990678,0.706317430622214,-5.16647320456044));
#40849=CARTESIAN_POINT('Ctrl Pts',(5.94219718982269,2.17827547934186,-4.44516603182682));
#40850=CARTESIAN_POINT('Ctrl Pts',(5.99523048057758,3.65023352806152,-3.7238588590932));
#40851=CARTESIAN_POINT('Ctrl Pts',(6.04826377133247,4.72830170425962,-2.19874798128889));
#40852=CARTESIAN_POINT('Ctrl Pts',(6.10129706208736,4.91720840506355,-0.570479332131516));
#40853=CARTESIAN_POINT('Ctrl Pts',(6.15433035284225,5.10611510586748,1.05778931702586));
#40854=CARTESIAN_POINT('Ctrl Pts',(6.20736364359714,4.40586033127725,2.78921573753631));
#40855=CARTESIAN_POINT('Ctrl Pts',(6.26039693435203,3.1381457240098,3.82837126804708));
#40856=CARTESIAN_POINT('Ctrl Pts',(6.31343022510691,1.87043111674235,4.86752679855783));
#40857=CARTESIAN_POINT('Ctrl Pts',(6.3664635158618,0.0352566767976717,5.21441143906891));
#40858=CARTESIAN_POINT('Ctrl Pts',(6.41949680661669,-1.52428642115839,4.70966411245116));
#40859=CARTESIAN_POINT('Ctrl Pts',(6.47253009737158,-3.08382951911445,4.2049167858334));
#40860=CARTESIAN_POINT('Ctrl Pts',(6.52556338812647,-4.3677412750819,2.84853749208683));
#40861=CARTESIAN_POINT('Ctrl Pts',(6.57859667888136,-4.78618420382354,1.26365577601926));
#40862=CARTESIAN_POINT('Ctrl Pts',(6.59229096770194,-4.89423479317131,0.854406648587289));
#40863=CARTESIAN_POINT('Ctrl Pts',(6.60598525652252,-4.94457775183742,0.429921462983896));
#40864=CARTESIAN_POINT('Ctrl Pts',(6.6196795453431,-4.9407490012001,0.0045438707638676));
#40865=CARTESIAN_POINT('Origin',(8.75,0.,0.));
#40866=CARTESIAN_POINT('',(7.76432045465689,-4.93388715137377,-0.000577480970858357));
#40867=CARTESIAN_POINT('',(7.6196795453431,-4.93408355834929,-0.0011800419470579));
#40868=CARTESIAN_POINT('',(8.75,-4.942,-6.05220448138622E-16));
#40869=CARTESIAN_POINT('Ctrl Pts',(7.76432045465689,-4.93388715137377,-0.000577480970858357));
#40870=CARTESIAN_POINT('Ctrl Pts',(7.73668226171302,-4.93299226451753,0.860940067097838));
#40871=CARTESIAN_POINT('Ctrl Pts',(7.70904406876916,-4.71867004547136,1.72287425155414));
#40872=CARTESIAN_POINT('Ctrl Pts',(7.68140587582529,-4.29348773831838,2.46380691579945));
#40873=CARTESIAN_POINT('Ctrl Pts',(7.6283725850704,-3.4776306030537,3.88553870168424));
#40874=CARTESIAN_POINT('Ctrl Pts',(7.57533929431551,-1.88539720710199,4.86174896359399));
#40875=CARTESIAN_POINT('Ctrl Pts',(7.52230600356062,-0.248270018437432,
4.94396030276934));
#40876=CARTESIAN_POINT('Ctrl Pts',(7.46927271280573,1.38885717022713,5.02617164194469));
#40877=CARTESIAN_POINT('Ctrl Pts',(7.41623942205083,3.07087815160453,4.21438405838564));
#40878=CARTESIAN_POINT('Ctrl Pts',(7.36320613129594,4.02506145193688,2.88153809371726));
#40879=CARTESIAN_POINT('Ctrl Pts',(7.31017284054106,4.97924475226923,1.54869212904887));
#40880=CARTESIAN_POINT('Ctrl Pts',(7.25713954978617,5.20559037155652,-0.305212216728855));
#40881=CARTESIAN_POINT('Ctrl Pts',(7.20410625903128,4.60011364733754,-1.8284791245895));
#40882=CARTESIAN_POINT('Ctrl Pts',(7.15107296827639,3.99463692311855,-3.35174603245014));
#40883=CARTESIAN_POINT('Ctrl Pts',(7.0980396775215,2.55733785539328,-4.5443755023937));
#40884=CARTESIAN_POINT('Ctrl Pts',(7.04500638676661,0.948521065327934,-4.85846573168681));
#40885=CARTESIAN_POINT('Ctrl Pts',(6.99197309601172,-0.6602957247374,-5.17255596097992));
#40886=CARTESIAN_POINT('Ctrl Pts',(6.93893980525684,-2.44063023714281,-4.60810694962259));
#40887=CARTESIAN_POINT('Ctrl Pts',(6.88590651450195,-3.57458511704265,-3.42443027646787));
#40888=CARTESIAN_POINT('Ctrl Pts',(6.84537782788693,-4.44116724515231,-2.5198501484589));
#40889=CARTESIAN_POINT('Ctrl Pts',(6.80484914127191,-4.930250577109,-1.25362852508438));
#40890=CARTESIAN_POINT('Ctrl Pts',(6.76432045465689,-4.94186257797741,0.00456669625063827));
#40891=CARTESIAN_POINT('Ctrl Pts',(6.6196795453431,-4.9407490012001,0.0045438707638676));
#40892=CARTESIAN_POINT('Ctrl Pts',(6.65901854727741,-4.92975031184129,-1.21742027373473));
#40893=CARTESIAN_POINT('Ctrl Pts',(6.69835754921173,-4.47171793942916,-2.44674870157877));
#40894=CARTESIAN_POINT('Ctrl Pts',(6.73769655114603,-3.65047313959733,-3.34341606856897));
#40895=CARTESIAN_POINT('Ctrl Pts',(6.79072984190092,-2.54334504511365,-4.55222205870107));
#40896=CARTESIAN_POINT('Ctrl Pts',(6.8437631326558,-0.776114754630469,-5.15644990057672));
#40897=CARTESIAN_POINT('Ctrl Pts',(6.89679642341069,0.839340542852879,-4.87851335994245));
#40898=CARTESIAN_POINT('Ctrl Pts',(6.94982971416558,2.45479584033622,-4.60057681930817));
#40899=CARTESIAN_POINT('Ctrl Pts',(7.00286300492048,3.91847614481972,-3.44047589616397));
#40900=CARTESIAN_POINT('Ctrl Pts',(7.05589629567537,4.5579571217266,-1.93116856527833));
#40901=CARTESIAN_POINT('Ctrl Pts',(7.10892958643026,5.19743809863347,-0.421861234392705));
#40902=CARTESIAN_POINT('Ctrl Pts',(7.16196287718514,5.01271974796372,1.43665250423437));
#40903=CARTESIAN_POINT('Ctrl Pts',(7.21499616794003,4.08866289196774,2.79055924617738));
#40904=CARTESIAN_POINT('Ctrl Pts',(7.26802945869492,3.16460603597175,4.1444659881204));
#40905=CARTESIAN_POINT('Ctrl Pts',(7.32106274944981,1.50121067464953,4.99376573337936));
#40906=CARTESIAN_POINT('Ctrl Pts',(7.3740960402047,-0.137348450334091,4.94828460718909));
#40907=CARTESIAN_POINT('Ctrl Pts',(7.42712933095959,-1.77590757531773,4.90280348099881));
#40908=CARTESIAN_POINT('Ctrl Pts',(7.48016262171448,-3.38963046396277,3.96254148335925));
#40909=CARTESIAN_POINT('Ctrl Pts',(7.53319591246937,-4.23716223434557,2.5594611445621));
#40910=CARTESIAN_POINT('Ctrl Pts',(7.56202379009394,-4.69786421628478,1.79677363774235));
#40911=CARTESIAN_POINT('Ctrl Pts',(7.59085166771852,-4.93217199616782,0.89733253701383));
#40912=CARTESIAN_POINT('Ctrl Pts',(7.6196795453431,-4.93408355834929,-0.0011800419470579));
#40913=CARTESIAN_POINT('Origin',(8.75,0.,0.));
#40914=CARTESIAN_POINT('',(8.76432045465689,-4.94398902458143,-0.00436563055240979));
#40915=CARTESIAN_POINT('',(8.6196795453431,-4.94509229898035,-0.00412964409767292));
#40916=CARTESIAN_POINT('',(8.75,-4.942,-6.05220448138622E-16));
#40917=CARTESIAN_POINT('Ctrl Pts',(8.76432045465689,-4.94398902458143,-0.00436563055240979));
#40918=CARTESIAN_POINT('Ctrl Pts',(8.72154867290902,-4.93175999696903,1.32200133659815));
#40919=CARTESIAN_POINT('Ctrl Pts',(8.67877689116116,-4.38072220103998,2.65732794935703));
#40920=CARTESIAN_POINT('Ctrl Pts',(8.63600510941329,-3.42664403930687,3.5724630306423));
#40921=CARTESIAN_POINT('Ctrl Pts',(8.5829718186584,-2.24367006706628,4.70715096886972));
#40922=CARTESIAN_POINT('Ctrl Pts',(8.52993852790351,-0.441068126124786,
5.1958430039501));
#40923=CARTESIAN_POINT('Ctrl Pts',(8.47690523714862,1.15303462585385,4.81403080889657));
#40924=CARTESIAN_POINT('Ctrl Pts',(8.42387194639373,2.74713737783251,4.43221861384304));
#40925=CARTESIAN_POINT('Ctrl Pts',(8.37083865563885,4.13274094084831,3.17990218865558));
#40926=CARTESIAN_POINT('Ctrl Pts',(8.31780536488396,4.67328994778057,1.63240391490459));
#40927=CARTESIAN_POINT('Ctrl Pts',(8.26477207412907,5.21383895471282,0.0849056411536261));
#40928=CARTESIAN_POINT('Ctrl Pts',(8.21173878337417,4.90933340556155,-1.75777448116088));
#40929=CARTESIAN_POINT('Ctrl Pts',(8.15870549261928,3.89966514731939,-3.04909711491891));
#40930=CARTESIAN_POINT('Ctrl Pts',(8.10567220186439,2.88999688907721,-4.34041974867696));
#40931=CARTESIAN_POINT('Ctrl Pts',(8.05263891110951,1.17516592174414,-5.0803848938785));
#40932=CARTESIAN_POINT('Ctrl Pts',(7.99960562035462,-0.457023158113981,
-4.92904770826675));
#40933=CARTESIAN_POINT('Ctrl Pts',(7.94657232959973,-2.08921223797207,-4.77771052265501));
#40934=CARTESIAN_POINT('Ctrl Pts',(7.89353903884484,-3.6387594303552,-3.73507100623));
#40935=CARTESIAN_POINT('Ctrl Pts',(7.84050574808995,-4.39379258925795,-2.28012459308761));
#40936=CARTESIAN_POINT('Ctrl Pts',(7.81511065027893,-4.75534173410583,-1.58342058046442));
#40937=CARTESIAN_POINT('Ctrl Pts',(7.78971555246791,-4.93470940987996,-0.792174907168253));
#40938=CARTESIAN_POINT('Ctrl Pts',(7.76432045465689,-4.93388715137377,-0.000577480970858357));
#40939=CARTESIAN_POINT('Ctrl Pts',(7.6196795453431,-4.93408355834929,-0.0011800419470579));
#40940=CARTESIAN_POINT('Ctrl Pts',(7.64388495847341,-4.93568860721656,-0.755618799449938));
#40941=CARTESIAN_POINT('Ctrl Pts',(7.66809037160372,-4.77345034543105,-1.50940293321614));
#40942=CARTESIAN_POINT('Ctrl Pts',(7.69229578473404,-4.44381576150152,-2.18102880046318));
#40943=CARTESIAN_POINT('Ctrl Pts',(7.74532907548893,-3.72159686615413,-3.6525397267366));
#40944=CARTESIAN_POINT('Ctrl Pts',(7.79836236624381,-2.19581842333879,-4.72966289932871));
#40945=CARTESIAN_POINT('Ctrl Pts',(7.8513956569987,-0.567433059567756,-4.91756086627617));
#40946=CARTESIAN_POINT('Ctrl Pts',(7.90442894775359,1.06095230420328,-5.10545883322364));
#40947=CARTESIAN_POINT('Ctrl Pts',(7.95746223850848,2.79194458893001,-4.40413159452647));
#40948=CARTESIAN_POINT('Ctrl Pts',(8.01049552926337,3.83031458280598,-3.13577348470557));
#40949=CARTESIAN_POINT('Ctrl Pts',(8.06352882001826,4.86868457668194,-1.86741537488468));
#40950=CARTESIAN_POINT('Ctrl Pts',(8.11656211077315,5.21443227970714,-0.0320263939400439));
#40951=CARTESIAN_POINT('Ctrl Pts',(8.16959540152804,4.7087189288313,1.52720371918551));
#40952=CARTESIAN_POINT('Ctrl Pts',(8.22262869228293,4.20300557795547,3.08643383231107));
#40953=CARTESIAN_POINT('Ctrl Pts',(8.27566198303782,2.84583117317862,4.36950507761757));
#40954=CARTESIAN_POINT('Ctrl Pts',(8.32869527379271,1.26069053981566,4.78696610740548));
#40955=CARTESIAN_POINT('Ctrl Pts',(8.3817285645476,-0.324450093547317,5.20442713719338));
#40956=CARTESIAN_POINT('Ctrl Pts',(8.43476185530248,-2.1375569554964,4.75627795146268));
#40957=CARTESIAN_POINT('Ctrl Pts',(8.48779514605737,-3.34567685873883,3.6484012262265));
#40958=CARTESIAN_POINT('Ctrl Pts',(8.53175661248595,-4.34713691924224,2.73003684094686));
#40959=CARTESIAN_POINT('Ctrl Pts',(8.57571807891452,-4.93288436617281,1.35834522977113));
#40960=CARTESIAN_POINT('Ctrl Pts',(8.6196795453431,-4.94509229898035,-0.00412964409767292));
#40961=CARTESIAN_POINT('Origin',(8.75,0.,0.));
#40962=CARTESIAN_POINT('',(9.76432045465689,-4.94845593707282,0.00263657310841547));
#40963=CARTESIAN_POINT('',(9.6196795453431,-4.94762324771633,0.00315517675713146));
#40964=CARTESIAN_POINT('',(8.75,-4.942,-6.05220448138622E-16));
#40965=CARTESIAN_POINT('Ctrl Pts',(9.76432045465689,-4.94845593707282,0.00263657310841547));
#40966=CARTESIAN_POINT('Ctrl Pts',(9.75944837485992,-4.94942745139196,0.153366619893802));
#40967=CARTESIAN_POINT('Ctrl Pts',(9.75457629506294,-4.94314008508034,0.304014507117773));
#40968=CARTESIAN_POINT('Ctrl Pts',(9.74970421526596,-4.92932988376321,0.453969574366955));
#40969=CARTESIAN_POINT('Ctrl Pts',(9.69667092451108,-4.77900385209818,2.08625209291875));
#40970=CARTESIAN_POINT('Ctrl Pts',(9.64363763375619,-3.73732446482242,3.63644489277922));
#40971=CARTESIAN_POINT('Ctrl Pts',(9.5906043430013,-2.28284606639771,4.39237923164047));
#40972=CARTESIAN_POINT('Ctrl Pts',(9.53757105224641,-0.828367667972992,
5.14831357050172));
#40973=CARTESIAN_POINT('Ctrl Pts',(9.48453776149151,1.03890974160068,5.10998944836375));
#40974=CARTESIAN_POINT('Ctrl Pts',(9.43150447073663,2.46114667006327,4.29501321835778));
#40975=CARTESIAN_POINT('Ctrl Pts',(9.37847117998174,3.88338359852585,3.4800369883518));
#40976=CARTESIAN_POINT('Ctrl Pts',(9.32543788922685,4.86058004587734,1.88840865047781));
#40977=CARTESIAN_POINT('Ctrl Pts',(9.27240459847196,4.9438055532949,0.251332705057519));
#40978=CARTESIAN_POINT('Ctrl Pts',(9.21937130771707,5.02703106071247,-1.38574324036278));
#40979=CARTESIAN_POINT('Ctrl Pts',(9.16633801696218,4.2162856281961,-3.06826679332938));
#40980=CARTESIAN_POINT('Ctrl Pts',(9.11330472620729,2.88403102634981,-4.02327559539163));
#40981=CARTESIAN_POINT('Ctrl Pts',(9.0602714354524,1.55177642450353,-4.97828439745387));
#40982=CARTESIAN_POINT('Ctrl Pts',(9.00723814469752,-0.301987346672683,
-5.20577844861174));
#40983=CARTESIAN_POINT('Ctrl Pts',(8.95420485394263,-1.82562904905711,-4.60124548928475));
#40984=CARTESIAN_POINT('Ctrl Pts',(8.90117156318774,-3.34927075144153,-3.99671252995776));
#40985=CARTESIAN_POINT('Ctrl Pts',(8.84813827243285,-4.54279038503418,-2.56015256014591));
#40986=CARTESIAN_POINT('Ctrl Pts',(8.79510498167796,-4.85787720006066,-0.951530654552757));
#40987=CARTESIAN_POINT('Ctrl Pts',(8.78484347267093,-4.91884392764563,-0.640275442247928));
#40988=CARTESIAN_POINT('Ctrl Pts',(8.77458196366391,-4.94692292800709,-0.322578387277471));
#40989=CARTESIAN_POINT('Ctrl Pts',(8.76432045465689,-4.94398902458143,-0.00436563055240979));
#40990=CARTESIAN_POINT('Ctrl Pts',(8.6196795453431,-4.94509229898035,-0.00412964409767292));
#40991=CARTESIAN_POINT('Ctrl Pts',(8.62875136966941,-4.94761151025364,-0.285287979087153));
#40992=CARTESIAN_POINT('Ctrl Pts',(8.63782319399572,-4.92570720098754,-0.566053829919258));
#40993=CARTESIAN_POINT('Ctrl Pts',(8.64689501832204,-4.87799246076471,-0.842362572383541));
#40994=CARTESIAN_POINT('Ctrl Pts',(8.69992830907693,-4.59905521501237,-2.45764538101576));
#40995=CARTESIAN_POINT('Ctrl Pts',(8.75296159983182,-3.43804777897189,-3.92060673353855));
#40996=CARTESIAN_POINT('Ctrl Pts',(8.80599489058671,-1.9283445855655,-4.55915258682474));
#40997=CARTESIAN_POINT('Ctrl Pts',(8.8590281813416,-0.418641392159106,-5.19769844011094));
#40998=CARTESIAN_POINT('Ctrl Pts',(8.91206147209648,1.4397575586132,-5.01182879416055));
#40999=CARTESIAN_POINT('Ctrl Pts',(8.96509476285137,2.79309159671432,-4.08693338372359));
#41000=CARTESIAN_POINT('Ctrl Pts',(9.01812805360626,4.14642563481545,-3.16203797328663));
#41001=CARTESIAN_POINT('Ctrl Pts',(9.07116134436116,4.9946947602454,-1.4981167983631));
#41002=CARTESIAN_POINT('Ctrl Pts',(9.12419463511605,4.94819857170044,0.140413837109267));
#41003=CARTESIAN_POINT('Ctrl Pts',(9.17722792587094,4.90170238315548,1.77894447258163));
#41004=CARTESIAN_POINT('Ctrl Pts',(9.23026121662582,3.96044088063561,3.39208456860284));
#41005=CARTESIAN_POINT('Ctrl Pts',(9.28329450738071,2.55683577355735,4.23874698203242));
#41006=CARTESIAN_POINT('Ctrl Pts',(9.3363277981356,1.15323066647911,5.085409395462));
#41007=CARTESIAN_POINT('Ctrl Pts',(9.38936108889049,-0.712718045157501,
5.16559412629996));
#41008=CARTESIAN_POINT('Ctrl Pts',(9.44239437964538,-2.18378128164371,4.44246378314692));
#41009=CARTESIAN_POINT('Ctrl Pts',(9.49542767040027,-3.65484451812992,3.71933343999387));
#41010=CARTESIAN_POINT('Ctrl Pts',(9.54846096115516,-4.73102227946572,2.19288802284981));
#41011=CARTESIAN_POINT('Ctrl Pts',(9.60149425191005,-4.91791144181518,0.564386570615904));
#41012=CARTESIAN_POINT('Ctrl Pts',(9.60755601638773,-4.93927308220122,0.378247032327898));
#41013=CARTESIAN_POINT('Ctrl Pts',(9.61361778086541,-4.94901639309396,0.190774157883547));
#41014=CARTESIAN_POINT('Ctrl Pts',(9.6196795453431,-4.94762324771633,0.00315517675713146));
#41015=CARTESIAN_POINT('Origin',(8.75,0.,0.));
#41016=CARTESIAN_POINT('',(10.7643204546569,-4.93580407701378,0.00307338633379534));
#41017=CARTESIAN_POINT('',(10.6196795453431,-4.93516283533062,0.00258890295936728));
#41018=CARTESIAN_POINT('',(8.75,-4.942,-6.05220448138622E-16));
#41019=CARTESIAN_POINT('Ctrl Pts',(10.7643204546569,-4.93580407701378,0.00307338633379534));
#41020=CARTESIAN_POINT('Ctrl Pts',(10.7443147860559,-4.93932984348302,0.626070349929172));
#41021=CARTESIAN_POINT('Ctrl Pts',(10.7243091174549,-4.83006652292542,1.24787603993653));
#41022=CARTESIAN_POINT('Ctrl Pts',(10.704303448854,-4.60237556535654,1.82277827304598));
#41023=CARTESIAN_POINT('Ctrl Pts',(10.6512701580991,-3.99878660285512,3.34679418534805));
#41024=CARTESIAN_POINT('Ctrl Pts',(10.5982368673442,-2.56296628237974,4.54120352427818));
#41025=CARTESIAN_POINT('Ctrl Pts',(10.5452035765893,-0.954539878637368,
4.85728680405981));
#41026=CARTESIAN_POINT('Ctrl Pts',(10.4921702858344,0.653886525104984,5.17337008384144));
#41027=CARTESIAN_POINT('Ctrl Pts',(10.4391369950795,2.43491901211431,4.61112730447459));
#41028=CARTESIAN_POINT('Ctrl Pts',(10.3861037043246,3.57033957324573,3.42885648715834));
#41029=CARTESIAN_POINT('Ctrl Pts',(10.3330704135697,4.70576013437717,2.24658566984208));
#41030=CARTESIAN_POINT('Ctrl Pts',(10.2800371228148,5.19556876963067,0.444286814576416));
#41031=CARTESIAN_POINT('Ctrl Pts',(10.22700383206,4.81474417863934,-1.15005216039585));
#41032=CARTESIAN_POINT('Ctrl Pts',(10.1739705413051,4.43391958764801,-2.74439113536811));
#41033=CARTESIAN_POINT('Ctrl Pts',(10.1209372505502,3.18246177041184,-4.130770230047));
#41034=CARTESIAN_POINT('Ctrl Pts',(10.0679039597953,1.63529865834168,-4.67227779304397));
#41035=CARTESIAN_POINT('Ctrl Pts',(10.0148706690404,0.0881355462715097,
-5.21378535604094));
#41036=CARTESIAN_POINT('Ctrl Pts',(9.96183737828552,-1.75473286063265,-4.910421387356));
#41037=CARTESIAN_POINT('Ctrl Pts',(9.90880408753063,-3.04668072605759,-3.90155328439197));
#41038=CARTESIAN_POINT('Ctrl Pts',(9.86064287657272,-4.21993950007811,-2.98536820811364));
#41039=CARTESIAN_POINT('Ctrl Pts',(9.8124816656148,-4.93885237801332,-1.48735166259974));
#41040=CARTESIAN_POINT('Ctrl Pts',(9.76432045465689,-4.94845593707282,0.00263657310841547));
#41041=CARTESIAN_POINT('Ctrl Pts',(9.6196795453431,-4.94762324771633,0.00315517675713146));
#41042=CARTESIAN_POINT('Ctrl Pts',(9.6666510716203,-4.93682801392686,-1.45067067453174));
#41043=CARTESIAN_POINT('Ctrl Pts',(9.7136225978975,-4.25735291877213,-2.91326938798931));
#41044=CARTESIAN_POINT('Ctrl Pts',(9.76059412417471,-3.13340004119507,-3.83225642833011));
#41045=CARTESIAN_POINT('Ctrl Pts',(9.8136274149296,-1.86439891486239,-4.86984048771844));
#41046=CARTESIAN_POINT('Ctrl Pts',(9.8666607056845,-0.0287960988339278,
-5.21445111917136));
#41047=CARTESIAN_POINT('Ctrl Pts',(9.91969399643938,1.53012043070582,-4.70777193778096));
#41048=CARTESIAN_POINT('Ctrl Pts',(9.97272728719427,3.08903696024558,-4.20109275639056));
#41049=CARTESIAN_POINT('Ctrl Pts',(10.0257605779492,4.37126720329662,-2.84312376215679));
#41050=CARTESIAN_POINT('Ctrl Pts',(10.078793868704,4.78774617411819,-1.25772481999673));
#41051=CARTESIAN_POINT('Ctrl Pts',(10.1318271594589,5.20422514493976,0.32767412216334));
#41052=CARTESIAN_POINT('Ctrl Pts',(10.1848604502138,4.75495284353188,2.14050301224973));
#41053=CARTESIAN_POINT('Ctrl Pts',(10.2378937409687,3.64632791260652,3.34793636505146));
#41054=CARTESIAN_POINT('Ctrl Pts',(10.2909270317236,2.53770298168117,4.55536971785319));
#41055=CARTESIAN_POINT('Ctrl Pts',(10.3439603224785,0.769725421238379,5.15740753337025));
#41056=CARTESIAN_POINT('Ctrl Pts',(10.3969936132334,-0.845384278590161,
4.87746968950768));
#41057=CARTESIAN_POINT('Ctrl Pts',(10.4500269039883,-2.4604939784187,4.59753184564511));
#41058=CARTESIAN_POINT('Ctrl Pts',(10.5030601947432,-3.92273581763298,3.43561834240286));
#41059=CARTESIAN_POINT('Ctrl Pts',(10.5560934854981,-4.56034630228406,1.92551986586069));
#41060=CARTESIAN_POINT('Ctrl Pts',(10.5772888387797,-4.81517452972229,1.32199196395519));
#41061=CARTESIAN_POINT('Ctrl Pts',(10.5984841920614,-4.93828509595529,0.662848773962371));
#41062=CARTESIAN_POINT('Ctrl Pts',(10.6196795453431,-4.93516283533062,0.00258890295936728));
#41063=CARTESIAN_POINT('Origin',(8.75,0.,0.));
#41064=CARTESIAN_POINT('',(11.7643204546569,-4.93720552711113,-0.00379265621960889));
#41065=CARTESIAN_POINT('',(11.6196795453431,-4.9381236876051,-0.00410472656473214));
#41066=CARTESIAN_POINT('',(8.75,-4.942,-6.05220448138622E-16));
#41067=CARTESIAN_POINT('Ctrl Pts',(11.7643204546569,-4.93720552711113,-0.00379265621960889));
#41068=CARTESIAN_POINT('Ctrl Pts',(11.7291811972519,-4.92942537133172,1.08969997146474));
#41069=CARTESIAN_POINT('Ctrl Pts',(11.694041939847,-4.57137406349285,2.18781921440517));
#41070=CARTESIAN_POINT('Ctrl Pts',(11.658902682442,-3.90343992071078,3.04426317473012));
#41071=CARTESIAN_POINT('Ctrl Pts',(11.6058693916871,-2.89537235710122,4.33683578204868));
#41072=CARTESIAN_POINT('Ctrl Pts',(11.5528361009322,-1.1814595146183,5.07892498719433));
#41073=CARTESIAN_POINT('Ctrl Pts',(11.4998028101773,0.450915814594913,4.92961016401842));
#41074=CARTESIAN_POINT('Ctrl Pts',(11.4467695194224,2.08329114380809,4.78029534084251));
#41075=CARTESIAN_POINT('Ctrl Pts',(11.3937362286675,3.63412895975154,3.73957648934505));
#41076=CARTESIAN_POINT('Ctrl Pts',(11.3407029379126,4.39096418931034,2.28556666546216));
#41077=CARTESIAN_POINT('Ctrl Pts',(11.2876696471578,5.14779941886913,0.83155684157926));
#41078=CARTESIAN_POINT('Ctrl Pts',(11.2346363564029,5.11063206204329,-1.03574395468909));
#41079=CARTESIAN_POINT('Ctrl Pts',(11.181603065648,4.29653704961789,-2.45848548077665));
#41080=CARTESIAN_POINT('Ctrl Pts',(11.1285697748931,3.4824420371925,-3.88122700686422));
#41081=CARTESIAN_POINT('Ctrl Pts',(11.0755364841382,1.89141936916755,-4.85940926277102));
#41082=CARTESIAN_POINT('Ctrl Pts',(11.0225031933833,0.254395295479178,-4.94364890604547));
#41083=CARTESIAN_POINT('Ctrl Pts',(10.9694699026284,-1.38262877820921,-5.02788854931992));
#41084=CARTESIAN_POINT('Ctrl Pts',(10.9164366118735,-3.06565425756101,-4.21818557996203));
#41085=CARTESIAN_POINT('Ctrl Pts',(10.8634033211186,-4.0214881949732,-2.88652285244607));
#41086=CARTESIAN_POINT('Ctrl Pts',(10.8303756989647,-4.6167543320991,-2.05720125510973));
#41087=CARTESIAN_POINT('Ctrl Pts',(10.7973480768108,-4.92998334264735,-1.0254405177534));
#41088=CARTESIAN_POINT('Ctrl Pts',(10.7643204546569,-4.93580407701378,0.00307338633379534));
#41089=CARTESIAN_POINT('Ctrl Pts',(10.6196795453431,-4.93516283533062,0.00258890295936728));
#41090=CARTESIAN_POINT('Ctrl Pts',(10.6515174828163,-4.93047282911924,-0.989199825904508));
#41091=CARTESIAN_POINT('Ctrl Pts',(10.6833554202895,-4.64095603026269,-1.98350818994138));
#41092=CARTESIAN_POINT('Ctrl Pts',(10.7151933577627,-4.08520230705393,-2.7956228753998));
#41093=CARTESIAN_POINT('Ctrl Pts',(10.7682266485176,-3.15946869708483,-4.14838369027595));
#41094=CARTESIAN_POINT('Ctrl Pts',(10.8212599392725,-1.49502234705878,-4.99562187018618));
#41095=CARTESIAN_POINT('Ctrl Pts',(10.8742932300274,0.143479170036918,-4.94811063718052));
#41096=CARTESIAN_POINT('Ctrl Pts',(10.9273265207823,1.78198068713267,-4.90059940417486));
#41097=CARTESIAN_POINT('Ctrl Pts',(10.9803598115372,3.39453737129806,-3.95833875825322));
#41098=CARTESIAN_POINT('Ctrl Pts',(11.0333931022921,4.24033010293758,-2.55420942144691));
#41099=CARTESIAN_POINT('Ctrl Pts',(11.0864263930469,5.08612283457709,-1.1500800846406));
#41100=CARTESIAN_POINT('Ctrl Pts',(11.1394596838018,5.16515161369075,0.715917943050361));
#41101=CARTESIAN_POINT('Ctrl Pts',(11.1924929745567,4.44111010008868,2.18653292499499));
#41102=CARTESIAN_POINT('Ctrl Pts',(11.2455262653116,3.71706858648663,3.6571479069396));
#41103=CARTESIAN_POINT('Ctrl Pts',(11.2985595560665,2.18995678016881,4.73237984313789));
#41104=CARTESIAN_POINT('Ctrl Pts',(11.3515928468214,0.561339864738128,4.91826012956756));
#41105=CARTESIAN_POINT('Ctrl Pts',(11.4046261375763,-1.06727705069257,5.10414041599724));
#41106=CARTESIAN_POINT('Ctrl Pts',(11.4576594283312,-2.79739907523614,4.40066905265832));
#41107=CARTESIAN_POINT('Ctrl Pts',(11.5106927190861,-3.83419680251794,3.13102539604688));
#41108=CARTESIAN_POINT('Ctrl Pts',(11.5470216611717,-4.54442549194757,2.26129224892483));
#41109=CARTESIAN_POINT('Ctrl Pts',(11.5833506032574,-4.92930870695169,1.12588026422444));
#41110=CARTESIAN_POINT('Ctrl Pts',(11.6196795453431,-4.9381236876051,-0.00410472656473213));
#41111=CARTESIAN_POINT('Origin',(8.75,0.,0.));
#41112=CARTESIAN_POINT('',(12.7643204546569,-4.949590084061,-0.00157034721157134));
#41113=CARTESIAN_POINT('',(12.6196795453431,-4.94998806776073,-0.000908059682992989));
#41114=CARTESIAN_POINT('',(8.75,-4.942,-6.05220448138622E-16));
#41115=CARTESIAN_POINT('Ctrl Pts',(12.7643204546569,-4.949590084061,-0.00157034721157134));
#41116=CARTESIAN_POINT('Ctrl Pts',(12.7140476084479,-4.94314587879761,1.55280243246766));
#41117=CARTESIAN_POINT('Ctrl Pts',(12.663774762239,-4.15080012520513,3.11283579625446));
#41118=CARTESIAN_POINT('Ctrl Pts',(12.61350191603,-2.8890133989013,4.01969958641386));
#41119=CARTESIAN_POINT('Ctrl Pts',(12.5604686252751,-1.55794290313953,4.9763585919273));
#41120=CARTESIAN_POINT('Ctrl Pts',(12.5074353345202,0.295537250634443,5.20614859064765));
#41121=CARTESIAN_POINT('Ctrl Pts',(12.4544020437653,1.8199267078499,4.60350370034535));
#41122=CARTESIAN_POINT('Ctrl Pts',(12.4013687530104,3.34431616506535,4.00085881004305));
#41123=CARTESIAN_POINT('Ctrl Pts',(12.3483354622555,4.53961492572229,2.56577903071809));
#41124=CARTESIAN_POINT('Ctrl Pts',(12.2953021715007,4.8566945907577,0.957548827601382));
#41125=CARTESIAN_POINT('Ctrl Pts',(12.2422688807458,5.17377425579312,-0.650681375515335));
#41126=CARTESIAN_POINT('Ctrl Pts',(12.1892355899909,4.61263482520701,-2.43206200242381));
#41127=CARTESIAN_POINT('Ctrl Pts',(12.136202299236,3.43106759472794,-3.56821479324049));
#41128=CARTESIAN_POINT('Ctrl Pts',(12.0831690084811,2.24950036424889,-4.70436758405716));
#41129=CARTESIAN_POINT('Ctrl Pts',(12.0301357177262,0.447505333876852,-5.19529253878204));
#41130=CARTESIAN_POINT('Ctrl Pts',(11.9771024269713,-1.14706924085875,-4.81545567582185));
#41131=CARTESIAN_POINT('Ctrl Pts',(11.9240691362164,-2.74164381559436,-4.43561881286166));
#41132=CARTESIAN_POINT('Ctrl Pts',(11.8710358454615,-4.12879793469354,-3.1850201322164));
#41133=CARTESIAN_POINT('Ctrl Pts',(11.8180025547066,-4.67126385187503,-1.63819278714807));
#41134=CARTESIAN_POINT('Ctrl Pts',(11.8001085213567,-4.85429800033287,-1.11627571005884));
#41135=CARTESIAN_POINT('Ctrl Pts',(11.7822144880068,-4.94116743118268,-0.560634063599559));
#41136=CARTESIAN_POINT('Ctrl Pts',(11.7643204546569,-4.93720552711113,-0.00379265621960889));
#41137=CARTESIAN_POINT('Ctrl Pts',(11.6196795453431,-4.9381236876051,-0.00410472656473213));
#41138=CARTESIAN_POINT('Ctrl Pts',(11.6363838940123,-4.94217688876905,-0.523681190767773));
#41139=CARTESIAN_POINT('Ctrl Pts',(11.6530882426815,-4.86672036673493,-1.04211026004547));
#41140=CARTESIAN_POINT('Ctrl Pts',(11.6697925913507,-4.70682314126475,-1.53303655666506));
#41141=CARTESIAN_POINT('Ctrl Pts',(11.7228258821056,-4.19917832270976,-3.09163890288159));
#41142=CARTESIAN_POINT('Ctrl Pts',(11.7758591728605,-2.84041525557975,-4.3730276454307));
#41143=CARTESIAN_POINT('Ctrl Pts',(11.8288924636154,-1.2547586151515,-4.78852440028367));
#41144=CARTESIAN_POINT('Ctrl Pts',(11.8819257543703,0.330898025276773,-5.20402115513665));
#41145=CARTESIAN_POINT('Ctrl Pts',(11.9349590451252,2.14344823900332,-4.75362592229347));
#41146=CARTESIAN_POINT('Ctrl Pts',(11.9879923358801,3.35019458202354,-3.64425320570872));
#41147=CARTESIAN_POINT('Ctrl Pts',(12.041025626635,4.55694092504374,-2.53488048912399));
#41148=CARTESIAN_POINT('Ctrl Pts',(12.0940589173898,5.15788339735766,-0.76653028879776));
#41149=CARTESIAN_POINT('Ctrl Pts',(12.1470922081447,4.87694505508189,0.848405671997188));
#41150=CARTESIAN_POINT('Ctrl Pts',(12.2001254988996,4.59600671280612,2.46334163279215));
#41151=CARTESIAN_POINT('Ctrl Pts',(12.2531587896545,3.43318755594063,3.9248633540558));
#41152=CARTESIAN_POINT('Ctrl Pts',(12.3061920804094,1.92269439062044,4.56153824532443));
#41153=CARTESIAN_POINT('Ctrl Pts',(12.3592253711643,0.412201225300242,5.19821313659306));
#41154=CARTESIAN_POINT('Ctrl Pts',(12.4122586619192,-1.44596594847468,5.01004119786668));
#41155=CARTESIAN_POINT('Ctrl Pts',(12.4652919526741,-2.79815304941714,4.08346970538315));
#41156=CARTESIAN_POINT('Ctrl Pts',(12.5167544835637,-4.11029056644383,3.18434175434171));
#41157=CARTESIAN_POINT('Ctrl Pts',(12.5682170144534,-4.94597675512516,1.58990687892319));
#41158=CARTESIAN_POINT('Ctrl Pts',(12.6196795453431,-4.94998806776073,-0.000908059682992989));
#41159=CARTESIAN_POINT('Origin',(8.75,0.,0.));
#41160=CARTESIAN_POINT('',(13.7643204546569,-4.94198723275246,0.00456325735460533));
#41161=CARTESIAN_POINT('',(13.6196795453431,-4.94087041225341,0.00455116726388009));
#41162=CARTESIAN_POINT('',(8.75,-4.942,-6.05220448138622E-16));
#41163=CARTESIAN_POINT('Ctrl Pts',(13.7643204546569,-4.94198723275246,0.00456325735460533));
#41164=CARTESIAN_POINT('Ctrl Pts',(13.7519473103988,-4.94554485058906,0.388644192184096));
#41165=CARTESIAN_POINT('Ctrl Pts',(13.7395741661407,-4.90456715137494,0.7719772057555));
#41166=CARTESIAN_POINT('Ctrl Pts',(13.7272010218827,-4.8161816818024,1.14405398553911));
#41167=CARTESIAN_POINT('Ctrl Pts',(13.6741677311278,-4.43734731209181,2.73883503987936));
#41168=CARTESIAN_POINT('Ctrl Pts',(13.6211344403729,-3.18757636531753,4.12682582225269));
#41169=CARTESIAN_POINT('Ctrl Pts',(13.568101149618,-1.64107775501197,4.67026475588749));
#41170=CARTESIAN_POINT('Ctrl Pts',(13.5150678588631,-0.0945791447063754,
5.2137036895223));
#41171=CARTESIAN_POINT('Ctrl Pts',(13.4620345681082,1.74864712913051,4.91259077441855));
#41172=CARTESIAN_POINT('Ctrl Pts',(13.4090012773533,3.04184000442437,3.90531638018477));
#41173=CARTESIAN_POINT('Ctrl Pts',(13.3559679865984,4.33503287971822,2.89804198595098));
#41174=CARTESIAN_POINT('Ctrl Pts',(13.3029346958435,5.07819235646905,1.18460611258716));
#41175=CARTESIAN_POINT('Ctrl Pts',(13.2499014050887,4.92989087406059,-0.447857354634542));
#41176=CARTESIAN_POINT('Ctrl Pts',(13.1968681143338,4.78158939165213,-2.08032082185625));
#41177=CARTESIAN_POINT('Ctrl Pts',(13.1438348235789,3.74182695008439,-3.63181188293583));
#41178=CARTESIAN_POINT('Ctrl Pts',(13.090801532824,2.28828517637576,-4.38954982336234));
#41179=CARTESIAN_POINT('Ctrl Pts',(13.0377682420691,0.83474340266712,-5.14728776378884));
#41180=CARTESIAN_POINT('Ctrl Pts',(12.9847349513142,-1.03257770318241,-5.11127258356227));
#41181=CARTESIAN_POINT('Ctrl Pts',(12.9317016605593,-2.45582271629555,-4.29805800017847));
#41182=CARTESIAN_POINT('Ctrl Pts',(12.8786683698044,-3.8790677294087,-3.48484341679467));
#41183=CARTESIAN_POINT('Ctrl Pts',(12.8256350790495,-4.85823664978545,-1.89442943025364));
#41184=CARTESIAN_POINT('Ctrl Pts',(12.7726017882947,-4.94349069109905,-0.257458430829869));
#41185=CARTESIAN_POINT('Ctrl Pts',(12.7698413437487,-4.94792826323556,-0.17225218390715));
#41186=CARTESIAN_POINT('Ctrl Pts',(12.7670808992028,-4.94994393057285,-0.0869197989643819));
#41187=CARTESIAN_POINT('Ctrl Pts',(12.7643204546569,-4.949590084061,-0.00157034721157134));
#41188=CARTESIAN_POINT('Ctrl Pts',(12.6196795453431,-4.94998806776073,-0.000908059682992989));
#41189=CARTESIAN_POINT('Ctrl Pts',(12.6212503052083,-4.95011050264269,-0.0494635468567493));
#41190=CARTESIAN_POINT('Ctrl Pts',(12.6228210650735,-4.94945813523979,-0.0980156616365649));
#41191=CARTESIAN_POINT('Ctrl Pts',(12.6243918249387,-4.94802086470688,-0.146544529912058));
#41192=CARTESIAN_POINT('Ctrl Pts',(12.6774251156936,-4.89949455094414,-1.78501622648295));
#41193=CARTESIAN_POINT('Ctrl Pts',(12.7304584064485,-3.95623489530868,-3.3969885733841));
#41194=CARTESIAN_POINT('Ctrl Pts',(12.7834916972034,-2.55158197219604,-4.24191143928385));
#41195=CARTESIAN_POINT('Ctrl Pts',(12.8365249879583,-1.14692904908337,-5.08683430518362));
#41196=CARTESIAN_POINT('Ctrl Pts',(12.8895582787132,0.719117141506524,-5.16470769008199));
#41197=CARTESIAN_POINT('Ctrl Pts',(12.9425915694681,2.18928350503452,-4.43975501421699));
#41198=CARTESIAN_POINT('Ctrl Pts',(12.995624860223,3.65944986856251,-3.71480233835198));
#41199=CARTESIAN_POINT('Ctrl Pts',(13.0486581509778,4.73373640502861,-2.18702360172358));
#41200=CARTESIAN_POINT('Ctrl Pts',(13.1016914417327,4.91860735974007,-0.558292365221102));
#41201=CARTESIAN_POINT('Ctrl Pts',(13.1547247324876,5.10347831445153,1.07043887128138));
#41202=CARTESIAN_POINT('Ctrl Pts',(13.2077580232425,4.39893368740835,2.80012260765795));
#41203=CARTESIAN_POINT('Ctrl Pts',(13.2607913139974,3.12864872498507,3.83613459652236));
#41204=CARTESIAN_POINT('Ctrl Pts',(13.3138246047523,1.85836376256179,4.87214658538676));
#41205=CARTESIAN_POINT('Ctrl Pts',(13.3668578955072,0.0223384647584107,
5.21448682673899));
#41206=CARTESIAN_POINT('Ctrl Pts',(13.4198911862621,-1.53595051362779,4.70587466445995));
#41207=CARTESIAN_POINT('Ctrl Pts',(13.472924477017,-3.09423949201398,4.19726250218091));
#41208=CARTESIAN_POINT('Ctrl Pts',(13.5259577677719,-4.37479215098299,2.8376979362706));
#41209=CARTESIAN_POINT('Ctrl Pts',(13.5789910585267,-4.78930381973335,1.2517878520372));
#41210=CARTESIAN_POINT('Ctrl Pts',(13.5925538874655,-4.89531177768519,0.846204361392297));
#41211=CARTESIAN_POINT('Ctrl Pts',(13.6061167164043,-4.94467730729444,0.42581699893638));
#41212=CARTESIAN_POINT('Ctrl Pts',(13.6196795453431,-4.94087041225341,0.00455116726388009));
#41213=CARTESIAN_POINT('Origin',(8.75,0.,0.));
#41214=CARTESIAN_POINT('',(14.7643204546569,-4.93250450453637,0.00244705770993248));
#41215=CARTESIAN_POINT('',(14.6196795453431,-4.93380912478971,-0.000781869070653209));
#41216=CARTESIAN_POINT('',(8.75,-4.942,-6.05220448138622E-16));
#41217=CARTESIAN_POINT('Ctrl Pts',(14.7643204546569,-4.93235156762733,0.00248647065513752));
#41218=CARTESIAN_POINT('Ctrl Pts',(14.7368137215948,-4.93231616464049,0.858797103940552));
#41219=CARTESIAN_POINT('Ctrl Pts',(14.7093069885327,-4.72122797606844,1.71429698878651));
#41220=CARTESIAN_POINT('Ctrl Pts',(14.6818002554707,-4.30032841604571,2.45180850600084));
#41221=CARTESIAN_POINT('Ctrl Pts',(14.6287669647158,-3.48882932980696,3.87373900713432));
#41222=CARTESIAN_POINT('Ctrl Pts',(14.5757336739609,-1.89741367011298,4.85707991822524));
#41223=CARTESIAN_POINT('Ctrl Pts',(14.522700383206,-0.260105224363101,4.94413079607572));
#41224=CARTESIAN_POINT('Ctrl Pts',(14.4696670924511,1.37720322138678,5.03118167392621));
#41225=CARTESIAN_POINT('Ctrl Pts',(14.4166338016962,3.06040445319256,4.22194251853627));
#41226=CARTESIAN_POINT('Ctrl Pts',(14.3636005109413,4.01768931210048,2.89107485014993));
#41227=CARTESIAN_POINT('Ctrl Pts',(14.3105672201864,4.9749741710084,1.56020718176359));
#41228=CARTESIAN_POINT('Ctrl Pts',(14.2575339294315,5.20634265701846,-0.292288999619142));
#41229=CARTESIAN_POINT('Ctrl Pts',(14.2045006386767,4.60474522293428,-1.81685003135272));
#41230=CARTESIAN_POINT('Ctrl Pts',(14.1514673479218,4.0031477888501,-3.34141106308629));
#41231=CARTESIAN_POINT('Ctrl Pts',(14.0984340571669,2.56858443467169,-4.5380369451707));
#41232=CARTESIAN_POINT('Ctrl Pts',(14.045400766412,0.960497304699148,-4.85621770190632));
#41233=CARTESIAN_POINT('Ctrl Pts',(13.9923674756571,-0.64758982527339,-5.17439845864193));
#41234=CARTESIAN_POINT('Ctrl Pts',(13.9393341849022,-2.42920073104005,-4.61413409002874));
#41235=CARTESIAN_POINT('Ctrl Pts',(13.8863008941473,-3.56605728759995,-3.43321624256855));
#41236=CARTESIAN_POINT('Ctrl Pts',(13.8456407476505,-4.43767497297469,-2.5278171621994));
#41237=CARTESIAN_POINT('Ctrl Pts',(13.8049806011537,-4.93029632707818,-1.25758860566906));
#41238=CARTESIAN_POINT('Ctrl Pts',(13.7643204546569,-4.94198723275246,0.00456325735460533));
#41239=CARTESIAN_POINT('Ctrl Pts',(13.6196795453431,-4.94087041225341,0.00455116726388009));
#41240=CARTESIAN_POINT('Ctrl Pts',(13.6591500071592,-4.92979160959116,-1.22141407925688));
#41241=CARTESIAN_POINT('Ctrl Pts',(13.6986204689753,-4.46838339598338,-2.45481928224828));
#41242=CARTESIAN_POINT('Ctrl Pts',(13.7380909307914,-3.6421712883116,-3.3524436960653));
#41243=CARTESIAN_POINT('Ctrl Pts',(13.7911242215463,-2.53205640960778,-4.5585095573779));
#41244=CARTESIAN_POINT('Ctrl Pts',(13.8441575123012,-0.763355973668449,
-5.15838567744665));
#41245=CARTESIAN_POINT('Ctrl Pts',(13.8971908030561,0.85141559526732,-4.87643353874572));
#41246=CARTESIAN_POINT('Ctrl Pts',(13.950224093811,2.46618716420311,-4.59448140004478));
#41247=CARTESIAN_POINT('Ctrl Pts',(14.0032573845658,3.92702986613531,-3.43070100257412));
#41248=CARTESIAN_POINT('Ctrl Pts',(14.0562906753207,4.56274980759158,-1.9198394346831));
#41249=CARTESIAN_POINT('Ctrl Pts',(14.1093239660756,5.19846974904784,-0.408977866792093));
#41250=CARTESIAN_POINT('Ctrl Pts',(14.1623572568305,5.00906693002818,1.44896487151931));
#41251=CARTESIAN_POINT('Ctrl Pts',(14.2153905475854,4.08169456080327,2.80062703726421));
#41252=CARTESIAN_POINT('Ctrl Pts',(14.2684238383403,3.15432219157834,4.15228920300912));
#41253=CARTESIAN_POINT('Ctrl Pts',(14.3214571290952,1.48898027214817,4.99767079618755));
#41254=CARTESIAN_POINT('Ctrl Pts',(14.3744904198501,-0.149531273418242,
4.94803484746135));
#41255=CARTESIAN_POINT('Ctrl Pts',(14.427523710605,-1.78804281898468,4.89839889873514));
#41256=CARTESIAN_POINT('Ctrl Pts',(14.4805570013599,-3.39972399068732,3.95374540810427));
#41257=CARTESIAN_POINT('Ctrl Pts',(14.5335902921148,-4.243641679441,2.54875117840475));
#41258=CARTESIAN_POINT('Ctrl Pts',(14.5622867098575,-4.70028719761052,1.78850604242019));
#41259=CARTESIAN_POINT('Ctrl Pts',(14.5909831276003,-4.93213822096086,0.893477127079331));
#41260=CARTESIAN_POINT('Ctrl Pts',(14.6196795453431,-4.93380912478971,-0.000781869070653209));
#41261=CARTESIAN_POINT('Origin',(0.59341010809499,0.,0.));
#41262=CARTESIAN_POINT('',(14.093410108095,-4.37198870530024,0.00403694074333234));
#41263=CARTESIAN_POINT('',(14.290589891905,-4.36475384329838,-0.000691689918779215));
#41264=CARTESIAN_POINT('',(0.59341010809499,-4.372,-3.0022354348761E-13));
#41265=CARTESIAN_POINT('',(15.,-3.64743349744463,2.4217429795102));
#41266=CARTESIAN_POINT('Ctrl Pts',(14.093410108095,-4.37198870530024,0.00403694074333216));
#41267=CARTESIAN_POINT('Ctrl Pts',(14.1340702545918,-4.36164620436778,-1.11254095183847));
#41268=CARTESIAN_POINT('Ctrl Pts',(14.2277636918435,-3.35742155165682,-3.70194317815195));
#41269=CARTESIAN_POINT('Ctrl Pts',(14.3744904198501,1.00322544797992,-5.07323874560084));
#41270=CARTESIAN_POINT('Ctrl Pts',(14.5335902921147,4.810536850935,-1.89741011965601));
#41271=CARTESIAN_POINT('Ctrl Pts',(14.6926901643794,4.19648807260473,3.01908925610601));
#41272=CARTESIAN_POINT('Ctrl Pts',(14.8481600670078,-0.168782852515597,
5.11779741395519));
#41273=CARTESIAN_POINT('Ctrl Pts',(14.9505966788814,-2.89351652081187,3.54232264574166));
#41274=CARTESIAN_POINT('Ctrl Pts',(15.,-3.64743349744463,2.4217429795102));
#41275=CARTESIAN_POINT('',(15.,1.10295997362678,4.23058663740352));
#41276=CARTESIAN_POINT('Origin',(15.,0.,0.));
#41277=CARTESIAN_POINT('Ctrl Pts',(14.290589891905,-4.36475384329838,-0.000691689918779284));
#41278=CARTESIAN_POINT('Ctrl Pts',(14.3149267649171,-4.36600746342641,-0.671622630368523));
#41279=CARTESIAN_POINT('Ctrl Pts',(14.3922969286841,-3.90437662282341,-2.80304411594494));
#41280=CARTESIAN_POINT('Ctrl Pts',(14.522700383206,-0.581919347715841,-5.1410577240212));
#41281=CARTESIAN_POINT('Ctrl Pts',(14.6818002554707,4.01308660375755,-3.2607181841902));
#41282=CARTESIAN_POINT('Ctrl Pts',(14.8143834823579,4.75806562994111,0.786704444467226));
#41283=CARTESIAN_POINT('Ctrl Pts',(14.9204500638677,3.11408383257965,3.31830903713004));
#41284=CARTESIAN_POINT('Ctrl Pts',(14.9734833546226,1.80781376844615,4.04682358287313));
#41285=CARTESIAN_POINT('Ctrl Pts',(15.,1.10295997362678,4.23058663740352));
#41286=CARTESIAN_POINT('Origin',(0.59341010809499,0.,0.));
#41287=CARTESIAN_POINT('',(13.093410108095,-4.37871465955376,-0.00138922663093295));
#41288=CARTESIAN_POINT('',(13.290589891905,-4.37100069655441,0.0040262450982749));
#41289=CARTESIAN_POINT('',(0.59341010809499,-4.372,-3.0022354348761E-13));
#41290=CARTESIAN_POINT('Ctrl Pts',(13.093410108095,-4.37871465955376,-0.00138922663093346));
#41291=CARTESIAN_POINT('Ctrl Pts',(13.0961705526409,-4.37902769414498,-0.0768946501564255));
#41292=CARTESIAN_POINT('Ctrl Pts',(13.1519642879417,-4.34298620877237,-1.60269498775243));
#41293=CARTESIAN_POINT('Ctrl Pts',(13.2607913139974,-2.56543051256322,-4.48988777162764));
#41294=CARTESIAN_POINT('Ctrl Pts',(13.4198911862621,2.39041400874848,-4.58547156439403));
#41295=CARTESIAN_POINT('Ctrl Pts',(13.5789910585267,5.14992922194199,-0.467835636203029));
#41296=CARTESIAN_POINT('Ctrl Pts',(13.7380909307914,3.17759419623094,4.07959959549261));
#41297=CARTESIAN_POINT('Ctrl Pts',(13.8971908030561,-1.71430297245472,4.87874912898118));
#41298=CARTESIAN_POINT('Ctrl Pts',(14.0156305288239,-4.18350516313649,2.13646272095719));
#41299=CARTESIAN_POINT('Ctrl Pts',(14.0810369638369,-4.37513599489588,0.343818779487714));
#41300=CARTESIAN_POINT('Ctrl Pts',(14.093410108095,-4.37198870530024,0.00403694074333216));
#41301=CARTESIAN_POINT('Ctrl Pts',(13.290589891905,-4.37100069655441,0.00402624509827507));
#41302=CARTESIAN_POINT('Ctrl Pts',(13.3300603537211,-4.36119969994578,-1.08053872005514));
#41303=CARTESIAN_POINT('Ctrl Pts',(13.4225641062921,-3.40455674710145,-3.63777190456466));
#41304=CARTESIAN_POINT('Ctrl Pts',(13.568101149618,0.889390123239341,-5.09411585972022));
#41305=CARTESIAN_POINT('Ctrl Pts',(13.7272010218827,4.7664465535393,-2.00545869799919));
#41306=CARTESIAN_POINT('Ctrl Pts',(13.8863008941473,4.26377407797028,2.92549576490892));
#41307=CARTESIAN_POINT('Ctrl Pts',(14.045400766412,-0.156020461739612,5.16912688108217));
#41308=CARTESIAN_POINT('Ctrl Pts',(14.1801637656646,-3.77910640678081,3.04553020145906));
#41309=CARTESIAN_POINT('Ctrl Pts',(14.2618934741622,-4.36327565804152,0.790425333789909));
#41310=CARTESIAN_POINT('Ctrl Pts',(14.290589891905,-4.36475384329838,-0.000691689918779284));
#41311=CARTESIAN_POINT('Origin',(0.59341010809499,0.,0.));
#41312=CARTESIAN_POINT('',(12.093410108095,-4.367758511641,-0.00335521914055352));
#41313=CARTESIAN_POINT('',(12.290589891905,-4.37906674064143,-0.000803325968382063));
#41314=CARTESIAN_POINT('',(0.59341010809499,-4.372,-3.0022354348761E-13));
#41315=CARTESIAN_POINT('Ctrl Pts',(12.093410108095,-4.367758511641,-0.00335521914055378));
#41316=CARTESIAN_POINT('Ctrl Pts',(12.1113041414449,-4.37126345793821,-0.495971696895518));
#41317=CARTESIAN_POINT('Ctrl Pts',(12.1822314655497,-4.06664955489653,-2.44436906711752));
#41318=CARTESIAN_POINT('Ctrl Pts',(12.3061920804094,-1.19826567241535,-5.0303809958746));
#41319=CARTESIAN_POINT('Ctrl Pts',(12.4652919526741,3.58420434344045,-3.72747292097139));
#41320=CARTESIAN_POINT('Ctrl Pts',(12.6243918249387,5.07346067115539,1.00028675173837));
#41321=CARTESIAN_POINT('Ctrl Pts',(12.7834916972034,1.90115420721842,4.80896873992654));
#41322=CARTESIAN_POINT('Ctrl Pts',(12.9398311249222,-2.93260813533299,4.20969054412402));
#41323=CARTESIAN_POINT('Ctrl Pts',(13.043137261886,-4.37301371552075,1.37370542993683));
#41324=CARTESIAN_POINT('Ctrl Pts',(13.093410108095,-4.37871465955376,-0.00138922663093346));
#41325=CARTESIAN_POINT('Ctrl Pts',(12.290589891905,-4.37906674064143,-0.000803325968382323));
#41326=CARTESIAN_POINT('Ctrl Pts',(12.2921606517702,-4.37917505413878,-0.0437585242530951));
#41327=CARTESIAN_POINT('Ctrl Pts',(12.3467647023903,-4.35911256894886,-1.53689886108888));
#41328=CARTESIAN_POINT('Ctrl Pts',(12.4544020437653,-2.66546494290799,-4.43123778702695));
#41329=CARTESIAN_POINT('Ctrl Pts',(12.61350191603,2.28699597084696,-4.63791267903968));
#41330=CARTESIAN_POINT('Ctrl Pts',(12.7726017882947,5.13813765686258,-0.583208933669766));
#41331=CARTESIAN_POINT('Ctrl Pts',(12.9317016605593,3.2682859109503,4.00734790289743));
#41332=CARTESIAN_POINT('Ctrl Pts',(13.090801532824,-1.60449996642509,4.91591419297749));
#41333=CARTESIAN_POINT('Ctrl Pts',(13.2104309432726,-4.15993144754704,2.20280898171477));
#41334=CARTESIAN_POINT('Ctrl Pts',(13.2770270629662,-4.37436851224028,0.376704152033278));
#41335=CARTESIAN_POINT('Ctrl Pts',(13.290589891905,-4.37100069655441,0.00402624509827507));
#41336=CARTESIAN_POINT('Origin',(0.59341010809499,0.,0.));
#41337=CARTESIAN_POINT('',(11.093410108095,-4.36651870188269,0.00271890834687631));
#41338=CARTESIAN_POINT('',(11.290589891905,-4.3685707734135,-0.00363129594146361));
#41339=CARTESIAN_POINT('',(0.59341010809499,-4.372,-3.0022354348761E-13));
#41340=CARTESIAN_POINT('Ctrl Pts',(11.093410108095,-4.36651870188269,0.00271890834687608));
#41341=CARTESIAN_POINT('Ctrl Pts',(11.1264377302489,-4.36136931891016,-0.907168341484959));
#41342=CARTESIAN_POINT('Ctrl Pts',(11.2124986431577,-3.63931805594909,-3.28556918685279));
#41343=CARTESIAN_POINT('Ctrl Pts',(11.3515928468214,0.265749570496903,-5.16429585585985));
#41344=CARTESIAN_POINT('Ctrl Pts',(11.5106927190861,4.4883018395813,-2.56821360809099));
#41345=CARTESIAN_POINT('Ctrl Pts',(11.6697925913507,4.58694349318866,2.38757701187169));
#41346=CARTESIAN_POINT('Ctrl Pts',(11.8288924636154,0.471041268600573,5.14963052385883));
#41347=CARTESIAN_POINT('Ctrl Pts',(11.9700983025302,-3.56606539792994,3.4016459105259));
#41348=CARTESIAN_POINT('Ctrl Pts',(12.05827085069,-4.36087570284549,0.964016243473005));
#41349=CARTESIAN_POINT('Ctrl Pts',(12.093410108095,-4.367758511641,-0.00335521914055378));
#41350=CARTESIAN_POINT('Ctrl Pts',(11.290589891905,-4.3685707734135,-0.00363129594146409));
#41351=CARTESIAN_POINT('Ctrl Pts',(11.3072942405742,-4.37215648678634,-0.463280891549555));
#41352=CARTESIAN_POINT('Ctrl Pts',(11.3770318799983,-4.09347257870959,-2.3779972764569));
#41353=CARTESIAN_POINT('Ctrl Pts',(11.4998028101773,-1.31076150706236,-5.00224776370858));
#41354=CARTESIAN_POINT('Ctrl Pts',(11.658902682442,3.49972182018105,-3.80690501300621));
#41355=CARTESIAN_POINT('Ctrl Pts',(11.8180025547066,5.09461487296727,0.886272086847998));
#41356=CARTESIAN_POINT('Ctrl Pts',(11.9771024269713,2.00850883058607,4.76513062511062));
#41357=CARTESIAN_POINT('Ctrl Pts',(12.1346315393708,-2.87435311497258,4.27065541760681));
#41358=CARTESIAN_POINT('Ctrl Pts',(12.2391273610153,-4.37551808446131,1.40653032672016));
#41359=CARTESIAN_POINT('Ctrl Pts',(12.290589891905,-4.37906674064143,-0.000803325968382323));
#41360=CARTESIAN_POINT('Origin',(0.59341010809499,0.,0.));
#41361=CARTESIAN_POINT('',(10.093410108095,-4.37771132272003,0.00233247625034503));
#41362=CARTESIAN_POINT('',(10.290589891905,-4.3659514196814,0.00229030427700283));
#41363=CARTESIAN_POINT('',(0.59341010809499,-4.372,-3.0022354348761E-13));
#41364=CARTESIAN_POINT('Ctrl Pts',(10.093410108095,-4.37771132272003,0.00233247625034497));
#41365=CARTESIAN_POINT('Ctrl Pts',(10.1415713190529,-4.36921541818575,-1.31580361571968));
#41366=CARTESIAN_POINT('Ctrl Pts',(10.2427658207657,-3.03288703287329,-4.10034412525587));
#41367=CARTESIAN_POINT('Ctrl Pts',(10.3969936132334,1.70828597395473,-4.88081279799705));
#41368=CARTESIAN_POINT('Ctrl Pts',(10.556093485498,5.02963780132612,-1.20138175675703));
#41369=CARTESIAN_POINT('Ctrl Pts',(10.7151933577627,3.72969242293982,3.58189460618598));
#41370=CARTESIAN_POINT('Ctrl Pts',(10.8742932300274,-0.997143291267936,
5.07407920638337));
#41371=CARTESIAN_POINT('Ctrl Pts',(11.0003654801381,-4.01673646885604,2.56218392279602));
#41372=CARTESIAN_POINT('Ctrl Pts',(11.073404439494,-4.36963781378144,0.553860698075588));
#41373=CARTESIAN_POINT('Ctrl Pts',(11.093410108095,-4.36651870188269,0.00271890834687608));
#41374=CARTESIAN_POINT('Ctrl Pts',(10.290589891905,-4.3659514196814,0.00229030427700276));
#41375=CARTESIAN_POINT('Ctrl Pts',(10.3224278293782,-4.36180234903057,-0.875107575648617));
#41376=CARTESIAN_POINT('Ctrl Pts',(10.4072990576063,-3.67904443619338,-3.21995217888924));
#41377=CARTESIAN_POINT('Ctrl Pts',(10.5452035765893,0.149882990889038,-5.1689567258239));
#41378=CARTESIAN_POINT('Ctrl Pts',(10.704303448854,4.42958624251035,-2.66820993668828));
#41379=CARTESIAN_POINT('Ctrl Pts',(10.8634033211187,4.63932753487269,2.28412315339565));
#41380=CARTESIAN_POINT('Ctrl Pts',(11.0225031933833,0.586393813370393,5.13777391729214));
#41381=CARTESIAN_POINT('Ctrl Pts',(11.1648987169788,-3.52322847002093,3.46679259372449));
#41382=CARTESIAN_POINT('Ctrl Pts',(11.2542609498193,-4.36077249429243,0.996023576525303));
#41383=CARTESIAN_POINT('Ctrl Pts',(11.290589891905,-4.3685707734135,-0.00363129594146409));
#41384=CARTESIAN_POINT('Origin',(0.59341010809499,0.,0.));
#41385=CARTESIAN_POINT('',(9.09341010809498,-4.37375961462363,-0.00386210780576171));
#41386=CARTESIAN_POINT('',(9.29058989190502,-4.37697467402181,0.00279126523279556));
#41387=CARTESIAN_POINT('',(0.59341010809499,-4.372,-3.0022354348761E-13));
#41388=CARTESIAN_POINT('Ctrl Pts',(9.09341010809498,-4.37375961462363,-0.00386210780576188));
#41389=CARTESIAN_POINT('Ctrl Pts',(9.103671617102,-4.37635512773107,-0.285372867093846));
#41390=CARTESIAN_POINT('Ctrl Pts',(9.16696641686391,-4.22313498793317,-2.01896688929275));
#41391=CARTESIAN_POINT('Ctrl Pts',(9.28329450738073,-1.90711126815764,-4.80661015155663));
#41392=CARTESIAN_POINT('Ctrl Pts',(9.44239437964536,3.01275227347471,-4.20284407001334));
#41393=CARTESIAN_POINT('Ctrl Pts',(9.60149425191006,5.16445949583093,0.26255028868963));
#41394=CARTESIAN_POINT('Ctrl Pts',(9.76059412417471,2.5709935704035,4.48670999721959));
#41395=CARTESIAN_POINT('Ctrl Pts',(9.91969399643938,-2.38473498159332,4.58842169004869));
#41396=CARTESIAN_POINT('Ctrl Pts',(10.0306326577461,-4.3124633006313,1.7196401851414));
#41397=CARTESIAN_POINT('Ctrl Pts',(10.088538028298,-4.37857078459848,0.135677632977564));
#41398=CARTESIAN_POINT('Ctrl Pts',(10.093410108095,-4.37771132272003,0.00233247625034497));
#41399=CARTESIAN_POINT('Ctrl Pts',(9.29058989190502,-4.37697467402181,0.00279126523279523));
#41400=CARTESIAN_POINT('Ctrl Pts',(9.33756141818222,-4.36742454004203,-1.28335333651436));
#41401=CARTESIAN_POINT('Ctrl Pts',(9.43756623521432,-3.08763898870623,-4.03814554925744));
#41402=CARTESIAN_POINT('Ctrl Pts',(9.59060434300129,1.59841338882536,-4.91789113187562));
#41403=CARTESIAN_POINT('Ctrl Pts',(9.74970421526597,5.00143481089275,-1.31386010630501));
#41404=CARTESIAN_POINT('Ctrl Pts',(9.90880408753063,3.80907230476851,3.49736282416303));
#41405=CARTESIAN_POINT('Ctrl Pts',(10.0679039597953,-0.883115813962409,
5.09516290273885));
#41406=CARTESIAN_POINT('Ctrl Pts',(10.1951658945868,-3.98729343645151,2.62854910513976));
#41407=CARTESIAN_POINT('Ctrl Pts',(10.2693945386233,-4.36871356526036,0.586397175184639));
#41408=CARTESIAN_POINT('Ctrl Pts',(10.290589891905,-4.3659514196814,0.00229030427700276));
#41409=CARTESIAN_POINT('Origin',(0.59341010809499,0.,0.));
#41410=CARTESIAN_POINT('',(8.09341010809498,-4.36482287045854,-0.000510875517043062));
#41411=CARTESIAN_POINT('',(8.29058989190502,-4.37473563964834,-0.00365333953792402));
#41412=CARTESIAN_POINT('',(0.59341010809499,-4.372,-3.0022354348761E-13));
#41413=CARTESIAN_POINT('Ctrl Pts',(8.09341010809498,-4.36482287045854,-0.000510875517042778));
#41414=CARTESIAN_POINT('Ctrl Pts',(8.118805205906,-4.36555029137901,-0.70080710120195));
#41415=CARTESIAN_POINT('Ctrl Pts',(8.1972335944719,-3.87549509935531,-2.86259042526824));
#41416=CARTESIAN_POINT('Ctrl Pts',(8.32869527379272,-0.477421201803847,
-5.14904297265438));
#41417=CARTESIAN_POINT('Ctrl Pts',(8.48779514605736,4.07371659009023,-3.18518565892236));
#41418=CARTESIAN_POINT('Ctrl Pts',(8.64689501832206,4.8818701276596,1.70526203113781));
#41419=CARTESIAN_POINT('Ctrl Pts',(8.8059948905867,1.20449733678236,5.02889259219775));
#41420=CARTESIAN_POINT('Ctrl Pts',(8.95483325384436,-3.27102321588964,3.81556246242598));
#41421=CARTESIAN_POINT('Ctrl Pts',(9.05063832634711,-4.36294105761814,1.16952445236876));
#41422=CARTESIAN_POINT('Ctrl Pts',(9.09341010809498,-4.37375961462363,-0.00386210780576188));
#41423=CARTESIAN_POINT('Ctrl Pts',(8.29058989190502,-4.37473563964834,-0.00365333953792416));
#41424=CARTESIAN_POINT('Ctrl Pts',(8.29966171623133,-4.37696429033364,-0.252383457015382));
#41425=CARTESIAN_POINT('Ctrl Pts',(8.36176683131253,-4.24430437552142,-1.95279653103946));
#41426=CARTESIAN_POINT('Ctrl Pts',(8.47690523714862,-2.01441124631645,-4.76263854153384));
#41427=CARTESIAN_POINT('Ctrl Pts',(8.63600510941329,2.91775399818566,-4.26934305867557));
#41428=CARTESIAN_POINT('Ctrl Pts',(8.79510498167796,5.16904858522312,0.146680844662566));
#41429=CARTESIAN_POINT('Ctrl Pts',(8.95420485394263,2.67095350892793,4.42793246332181));
#41430=CARTESIAN_POINT('Ctrl Pts',(9.1133047262073,-2.28124869702632,4.64074163565498));
#41431=CARTESIAN_POINT('Ctrl Pts',(9.22543307219475,-4.29417680922933,1.78561397709894));
#41432=CARTESIAN_POINT('Ctrl Pts',(9.28452812742733,-4.37820713690952,0.168770663347971));
#41433=CARTESIAN_POINT('Ctrl Pts',(9.29058989190502,-4.37697467402181,0.00279126523279523));
#41434=CARTESIAN_POINT('Origin',(0.59341010809499,0.,0.));
#41435=CARTESIAN_POINT('',(7.09341010809498,-4.37187842794764,0.00403998300431283));
#41436=CARTESIAN_POINT('',(7.29058989190502,-4.36499662426206,-0.00104393836387107));
#41437=CARTESIAN_POINT('',(0.59341010809499,-4.372,-3.0022354348761E-13));
#41438=CARTESIAN_POINT('Ctrl Pts',(7.09341010809498,-4.37187842794764,0.00403998300431242));
#41439=CARTESIAN_POINT('Ctrl Pts',(7.13393879471,-4.3616057311049,-1.1090376187109));
#41440=CARTESIAN_POINT('Ctrl Pts',(7.22750077207991,-3.36276294787998,-3.69501069902628));
#41441=CARTESIAN_POINT('Ctrl Pts',(7.3740960402047,0.990855843724147,-5.07531075254117));
#41442=CARTESIAN_POINT('Ctrl Pts',(7.53319591246937,4.80542779279021,-1.91008854942909));
#41443=CARTESIAN_POINT('Ctrl Pts',(7.69229578473403,4.20470963362949,3.01014807526144));
#41444=CARTESIAN_POINT('Ctrl Pts',(7.8513956569987,-0.25935090699094,5.16462115214535));
#41445=CARTESIAN_POINT('Ctrl Pts',(7.98510043145236,-3.81061099465694,2.98731690196163));
#41446=CARTESIAN_POINT('Ctrl Pts',(8.06577191515111,-4.36403119799085,0.76164103062551));
#41447=CARTESIAN_POINT('Ctrl Pts',(8.09341010809498,-4.36482287045854,-0.000510875517042778));
#41448=CARTESIAN_POINT('Ctrl Pts',(7.29058989190502,-4.36499662426206,-0.00104393836387148));
#41449=CARTESIAN_POINT('Ctrl Pts',(7.31479530503533,-4.36641655013163,-0.668467298906582));
#41450=CARTESIAN_POINT('Ctrl Pts',(7.39203400892053,-3.90842952464144,-2.79634607106463));
#41451=CARTESIAN_POINT('Ctrl Pts',(7.52230600356061,-0.59275896293977,-5.13704344525249));
#41452=CARTESIAN_POINT('Ctrl Pts',(7.68140587582529,4.00127074294363,-3.27573060374049));
#41453=CARTESIAN_POINT('Ctrl Pts',(7.84050574808995,4.91888038941839,1.59536649744721));
#41454=CARTESIAN_POINT('Ctrl Pts',(7.99960562035462,1.31695819333312,5.00061992792881));
#41455=CARTESIAN_POINT('Ctrl Pts',(8.14963366829297,-3.2206259976218,3.87905632732833));
#41456=CARTESIAN_POINT('Ctrl Pts',(8.24662842547644,-4.36393574441683,1.20167651650311));
#41457=CARTESIAN_POINT('Ctrl Pts',(8.29058989190502,-4.37473563964834,-0.00365333953792416));
#41458=CARTESIAN_POINT('Origin',(0.59341010809499,0.,0.));
#41459=CARTESIAN_POINT('',(6.09341010809498,-4.37876152077167,-0.00132541857997806));
#41460=CARTESIAN_POINT('',(6.29058989190502,-4.37089328879944,0.00401979016151965));
#41461=CARTESIAN_POINT('',(0.59341010809499,-4.372,-3.0022354348761E-13));
#41462=CARTESIAN_POINT('Ctrl Pts',(6.09341010809498,-4.37876152077167,-0.00132541857997809));
#41463=CARTESIAN_POINT('Ctrl Pts',(6.09603909275911,-4.3790475944532,-0.0732330197592887));
#41464=CARTESIAN_POINT('Ctrl Pts',(6.15170136817812,-4.34480561702315,-1.5954211178316));
#41465=CARTESIAN_POINT('Ctrl Pts',(6.26039693435203,-2.57655053740016,-4.48352114617468));
#41466=CARTESIAN_POINT('Ctrl Pts',(6.41949680661669,2.37904818745876,-4.59137280590671));
#41467=CARTESIAN_POINT('Ctrl Pts',(6.57859667888136,5.14874622778692,-0.48061089166393));
#41468=CARTESIAN_POINT('Ctrl Pts',(6.73769655114603,3.18770867422774,4.07174261783812));
#41469=CARTESIAN_POINT('Ctrl Pts',(6.8967964234107,-1.70223743368489,4.8829255836368));
#41470=CARTESIAN_POINT('Ctrl Pts',(7.01536760906034,-4.18091231648288,2.14385213795481));
#41471=CARTESIAN_POINT('Ctrl Pts',(7.08090550395511,-4.37504793621934,0.347465737670911));
#41472=CARTESIAN_POINT('Ctrl Pts',(7.09341010809498,-4.37187842794764,0.00403998300431242));
#41473=CARTESIAN_POINT('Ctrl Pts',(6.29058989190502,-4.37089328879944,0.00401979016151986));
#41474=CARTESIAN_POINT('Ctrl Pts',(6.32992889383933,-4.36116316539251,-1.0770055517542));
#41475=CARTESIAN_POINT('Ctrl Pts',(6.42230118652852,-3.40970001782311,-3.63066936637308));
#41476=CARTESIAN_POINT('Ctrl Pts',(6.56770676997262,0.876802331596175,-5.09625315459363));
#41477=CARTESIAN_POINT('Ctrl Pts',(6.72680664223727,4.76138972002301,-2.0173612671069));
#41478=CARTESIAN_POINT('Ctrl Pts',(6.88590651450195,4.27114975899821,2.91510862278235));
#41479=CARTESIAN_POINT('Ctrl Pts',(7.04500638676661,-0.143478642277096,
5.16913846066508));
#41480=CARTESIAN_POINT('Ctrl Pts',(7.17990084590097,-3.77469316016274,3.0533520140145));
#41481=CARTESIAN_POINT('Ctrl Pts',(7.26176201428044,-4.36330553768636,0.793836068762296));
#41482=CARTESIAN_POINT('Ctrl Pts',(7.29058989190502,-4.36499662426206,-0.00104393836387148));
#41483=CARTESIAN_POINT('Origin',(0.59341010809499,0.,0.));
#41484=CARTESIAN_POINT('',(5.09341010809498,-4.36784450635769,-0.00338885911202358));
#41485=CARTESIAN_POINT('',(5.29058989190502,-4.37909474916464,-0.000736964456646283));
#41486=CARTESIAN_POINT('',(0.59341010809499,-4.372,-3.0022354348761E-13));
#41487=CARTESIAN_POINT('Ctrl Pts',(5.09341010809498,-4.3678445063577,-0.0033888591120243));
#41488=CARTESIAN_POINT('Ctrl Pts',(5.11117268156311,-4.37136316807571,-0.492362019923694));
#41489=CARTESIAN_POINT('Ctrl Pts',(5.18196854578612,-4.06965919180842,-2.43703442403858));
#41490=CARTESIAN_POINT('Ctrl Pts',(5.30579770076401,-1.21072695590433,-5.0273964823116));
#41491=CARTESIAN_POINT('Ctrl Pts',(5.46489757302869,3.57495682182765,-3.73634277167034));
#41492=CARTESIAN_POINT('Ctrl Pts',(5.62399744529335,5.07592364569998,0.98771152242332));
#41493=CARTESIAN_POINT('Ctrl Pts',(5.78309731755802,1.91306507591506,4.80424360372137));
#41494=CARTESIAN_POINT('Ctrl Pts',(5.93956820515856,-2.92623401914661,4.21644954493704));
#41495=CARTESIAN_POINT('Ctrl Pts',(6.04300580200421,-4.37327676249022,1.37732573505887));
#41496=CARTESIAN_POINT('Ctrl Pts',(6.09341010809498,-4.37876152077167,-0.00132541857997809));
#41497=CARTESIAN_POINT('Ctrl Pts',(5.29058989190502,-4.37909474916464,-0.000736964456646279));
#41498=CARTESIAN_POINT('Ctrl Pts',(5.29202919188843,-4.37918634404097,-0.0400964851336176));
#41499=CARTESIAN_POINT('Ctrl Pts',(5.34650178262674,-4.36084783999699,-1.52963244896985));
#41500=CARTESIAN_POINT('Ctrl Pts',(5.45400766411994,-2.67643755901513,-4.42461982427826));
#41501=CARTESIAN_POINT('Ctrl Pts',(5.6131075363846,2.27549715061658,-4.64356448598052));
#41502=CARTESIAN_POINT('Ctrl Pts',(5.77220740864928,5.13667525644702,-0.595941201221052));
#41503=CARTESIAN_POINT('Ctrl Pts',(5.93130728091394,3.27820871991814,3.9992406950588));
#41504=CARTESIAN_POINT('Ctrl Pts',(6.0904071531786,-1.5923189924077,4.91986775797726));
#41505=CARTESIAN_POINT('Ctrl Pts',(6.21016802350897,-4.15726929526591,2.21014455144395));
#41506=CARTESIAN_POINT('Ctrl Pts',(6.27689560308444,-4.37428043930257,0.380335215735453));
#41507=CARTESIAN_POINT('Ctrl Pts',(6.29058989190502,-4.37089328879944,0.00401979016151986));
#41508=CARTESIAN_POINT('Origin',(0.59341010809499,0.,0.));
#41509=CARTESIAN_POINT('',(4.09341010809498,-4.36644361699374,0.00266903102634173));
#41510=CARTESIAN_POINT('',(4.29058989190502,-4.36866463568371,-0.00365796780793459));
#41511=CARTESIAN_POINT('',(0.59341010809499,-4.372,-3.0022354348761E-13));
#41512=CARTESIAN_POINT('Ctrl Pts',(4.09341010809498,-4.36644361699374,0.0026690310263415));
#41513=CARTESIAN_POINT('Ctrl Pts',(4.1263062703671,-4.36140744813966,-0.903629915781166));
#41514=CARTESIAN_POINT('Ctrl Pts',(4.21223572339411,-3.6437738264693,-3.27831824856905));
#41515=CARTESIAN_POINT('Ctrl Pts',(4.35119846717601,0.252959447065525,-5.16494338006019));
#41516=CARTESIAN_POINT('Ctrl Pts',(4.51029833944068,4.48192017162094,-2.5793250070162));
#41517=CARTESIAN_POINT('Ctrl Pts',(4.66939821170534,4.59284779079654,2.37620209998279));
#41518=CARTESIAN_POINT('Ctrl Pts',(4.82849808397002,0.483799317188488,5.14844819531533));
#41519=CARTESIAN_POINT('Ctrl Pts',(4.96983538276656,-3.56138743320807,3.40885374374836));
#41520=CARTESIAN_POINT('Ctrl Pts',(5.05813939080822,-4.36085758394431,0.96755345095109));
#41521=CARTESIAN_POINT('Ctrl Pts',(5.09341010809498,-4.3678445063577,-0.0033888591120243));
#41522=CARTESIAN_POINT('Ctrl Pts',(4.29058989190502,-4.36866463568371,-0.00365796780793456));
#41523=CARTESIAN_POINT('Ctrl Pts',(4.30716278069244,-4.37225371700844,-0.459665188165218));
#41524=CARTESIAN_POINT('Ctrl Pts',(4.37676896023474,-4.09638109039665,-2.37066280594993));
#41525=CARTESIAN_POINT('Ctrl Pts',(4.49940843053193,-1.32315190100328,-4.99898526062427));
#41526=CARTESIAN_POINT('Ctrl Pts',(4.6585083027966,3.49027724579729,-3.81556502166019));
#41527=CARTESIAN_POINT('Ctrl Pts',(4.81760817506126,5.09679560530872,0.873644852702682));
#41528=CARTESIAN_POINT('Ctrl Pts',(4.97670804732593,2.02031037891206,4.76013919238013));
#41529=CARTESIAN_POINT('Ctrl Pts',(5.13436861960719,-2.86783763983711,4.27736208016393));
#41530=CARTESIAN_POINT('Ctrl Pts',(5.23899590113355,-4.37581138554451,1.41016748213276));
#41531=CARTESIAN_POINT('Ctrl Pts',(5.29058989190502,-4.37909474916464,-0.000736964456646279));
#41532=CARTESIAN_POINT('Origin',(0.59341010809499,0.,0.));
#41533=CARTESIAN_POINT('',(3.09341010809498,-4.3772103018885,0.00211459834950888));
#41534=CARTESIAN_POINT('',(3.29058989190502,-4.36585073597542,0.00220040158241119));
#41535=CARTESIAN_POINT('',(0.59341010809499,-4.372,-3.0022354348761E-13));
#41536=CARTESIAN_POINT('Ctrl Pts',(3.09341010809498,-4.3772103018885,0.00211459834950896));
#41537=CARTESIAN_POINT('Ctrl Pts',(3.1414398591711,-4.3684488623825,-1.31256865588346));
#41538=CARTESIAN_POINT('Ctrl Pts',(3.24250290100212,-3.03968752820866,-4.09305073566412));
#41539=CARTESIAN_POINT('Ctrl Pts',(3.396599233588,1.69656360505873,-4.88527221384132));
#41540=CARTESIAN_POINT('Ctrl Pts',(3.55569910585268,5.02644857336042,-1.21371541889335));
#41541=CARTESIAN_POINT('Ctrl Pts',(3.71479897811734,3.73865941844861,3.57257592687282));
#41542=CARTESIAN_POINT('Ctrl Pts',(3.87389885038201,-0.984620426994229,
5.07656875848712));
#41543=CARTESIAN_POINT('Ctrl Pts',(4.00010256037456,-4.01351918209848,2.56951083998331));
#41544=CARTESIAN_POINT('Ctrl Pts',(4.07327297961222,-4.3695264683743,0.55745284394327));
#41545=CARTESIAN_POINT('Ctrl Pts',(4.09341010809498,-4.36644361699374,0.0026690310263415));
#41546=CARTESIAN_POINT('Ctrl Pts',(3.29058989190502,-4.36585073597542,0.00220040158241119));
#41547=CARTESIAN_POINT('Ctrl Pts',(3.32229636949643,-4.36183077367725,-0.871586062571754));
#41548=CARTESIAN_POINT('Ctrl Pts',(3.40703613784273,-3.68343867970127,-3.21262781785179));
#41549=CARTESIAN_POINT('Ctrl Pts',(3.54480919694392,0.137121248351661,-5.16935479018605));
#41550=CARTESIAN_POINT('Ctrl Pts',(3.70390906920859,4.42293632971135,-2.67915589298676));
#41551=CARTESIAN_POINT('Ctrl Pts',(3.86300894147325,4.6449860818125,2.2726085151474));
#41552=CARTESIAN_POINT('Ctrl Pts',(4.02210881373793,0.599116510517935,5.13631111808859));
#41553=CARTESIAN_POINT('Ctrl Pts',(4.16463579721518,-3.51842248411001,3.4739769218908));
#41554=CARTESIAN_POINT('Ctrl Pts',(4.25412948993755,-4.36076864666985,0.999559200156457));
#41555=CARTESIAN_POINT('Ctrl Pts',(4.29058989190502,-4.36866463568371,-0.00365796780793456));
#41556=CARTESIAN_POINT('Ctrl Pts',(2.11291034656191,-1.91898364244009,3.92834389788462));
#41557=CARTESIAN_POINT('Ctrl Pts',(2.13942699193936,-2.57348107768915,3.6086239586659));
#41558=CARTESIAN_POINT('Ctrl Pts',(2.19246028269425,-3.70959326419019,2.63583208807155));
#41559=CARTESIAN_POINT('Ctrl Pts',(2.29852686420402,-4.81962414156407,-0.171217860704528));
#41560=CARTESIAN_POINT('Ctrl Pts',(2.43111009109125,-3.28780625975168,-3.99092434960932));
#41561=CARTESIAN_POINT('Ctrl Pts',(2.59020996335592,1.58858351891899,-4.92397269005252));
#41562=CARTESIAN_POINT('Ctrl Pts',(2.74930983562058,4.99693901203929,-1.32514448694853));
#41563=CARTESIAN_POINT('Ctrl Pts',(2.90840970788525,3.81836490750785,3.48733811875686));
#41564=CARTESIAN_POINT('Ctrl Pts',(3.06750958014992,-0.870820132749773,
5.09763547084385));
#41565=CARTESIAN_POINT('Ctrl Pts',(3.22660945241459,-4.75871313630775,2.02310260362725));
#41566=CARTESIAN_POINT('Ctrl Pts',(3.38570932467925,-4.27484870062277,-2.9097329643648));
#41567=CARTESIAN_POINT('Ctrl Pts',(3.54480919694392,0.137121248351661,-5.16935479018605));
#41568=CARTESIAN_POINT('Ctrl Pts',(3.70390906920859,4.42293632971135,-2.67915589298676));
#41569=CARTESIAN_POINT('Ctrl Pts',(3.86300894147325,4.6449860818125,2.2726085151474));
#41570=CARTESIAN_POINT('Ctrl Pts',(4.02210881373793,0.599116510517935,5.13631111808859));
#41571=CARTESIAN_POINT('Ctrl Pts',(4.18120868600259,-3.99720561815913,3.28068243765374));
#41572=CARTESIAN_POINT('Ctrl Pts',(4.34030855826727,-4.92085506071136,-1.58926923856624));
#41573=CARTESIAN_POINT('Ctrl Pts',(4.49940843053193,-1.32315190100328,-4.99898526062427));
#41574=CARTESIAN_POINT('Ctrl Pts',(4.6585083027966,3.49027724579729,-3.81556502166019));
#41575=CARTESIAN_POINT('Ctrl Pts',(4.81760817506126,5.09679560530872,0.873644852702682));
#41576=CARTESIAN_POINT('Ctrl Pts',(4.97670804732593,2.02031037891206,4.76013919238013));
#41577=CARTESIAN_POINT('Ctrl Pts',(5.1358079195906,-2.91246205836179,4.27295475701679));
#41578=CARTESIAN_POINT('Ctrl Pts',(5.29490779185526,-5.16922638901484,-0.140276351883654));
#41579=CARTESIAN_POINT('Ctrl Pts',(5.45400766411994,-2.67643755901513,-4.42461982427826));
#41580=CARTESIAN_POINT('Ctrl Pts',(5.6131075363846,2.27549715061658,-4.64356448598052));
#41581=CARTESIAN_POINT('Ctrl Pts',(5.77220740864928,5.13667525644702,-0.595941201221052));
#41582=CARTESIAN_POINT('Ctrl Pts',(5.93130728091394,3.27820871991814,3.9992406950588));
#41583=CARTESIAN_POINT('Ctrl Pts',(6.0904071531786,-1.5923189924077,4.91986775797726));
#41584=CARTESIAN_POINT('Ctrl Pts',(6.24950702544328,-4.99980312661834,1.32005577562594));
#41585=CARTESIAN_POINT('Ctrl Pts',(6.40860689770794,-3.81340254294399,-3.49264077619605));
#41586=CARTESIAN_POINT('Ctrl Pts',(6.56770676997262,0.876802331596175,-5.09625315459363));
#41587=CARTESIAN_POINT('Ctrl Pts',(6.72680664223727,4.76138972002301,-2.0173612671069));
#41588=CARTESIAN_POINT('Ctrl Pts',(6.88590651450195,4.27114975899821,2.91510862278235));
#41589=CARTESIAN_POINT('Ctrl Pts',(7.04500638676661,-0.143478642277096,
5.16913846066508));
#41590=CARTESIAN_POINT('Ctrl Pts',(7.20410625903128,-4.42627698454096,2.67369605656947));
#41591=CARTESIAN_POINT('Ctrl Pts',(7.36320613129595,-4.6421539560531,-2.27837336598945));
#41592=CARTESIAN_POINT('Ctrl Pts',(7.52230600356061,-0.59275896293977,-5.13704344525249));
#41593=CARTESIAN_POINT('Ctrl Pts',(7.68140587582529,4.00127074294363,-3.27573060374049));
#41594=CARTESIAN_POINT('Ctrl Pts',(7.84050574808995,4.91888038941839,1.59536649744721));
#41595=CARTESIAN_POINT('Ctrl Pts',(7.99960562035462,1.31695819333312,5.00061992792881));
#41596=CARTESIAN_POINT('Ctrl Pts',(8.15870549261929,-3.49500247063371,3.81123815535816));
#41597=CARTESIAN_POINT('Ctrl Pts',(8.31780536488395,-5.09570900655666,-0.879959241718225));
#41598=CARTESIAN_POINT('Ctrl Pts',(8.47690523714862,-2.01441124631645,-4.76263854153384));
#41599=CARTESIAN_POINT('Ctrl Pts',(8.63600510941329,2.91775399818566,-4.26934305867557));
#41600=CARTESIAN_POINT('Ctrl Pts',(8.79510498167796,5.16904858522312,0.146680844662566));
#41601=CARTESIAN_POINT('Ctrl Pts',(8.95420485394263,2.67095350892793,4.42793246332181));
#41602=CARTESIAN_POINT('Ctrl Pts',(9.1133047262073,-2.28124869702632,4.64074163565498));
#41603=CARTESIAN_POINT('Ctrl Pts',(9.27240459847195,-5.13740966782362,0.589576501850538));
#41604=CARTESIAN_POINT('Ctrl Pts',(9.43150447073664,-3.27325122773264,-4.00329925770802));
#41605=CARTESIAN_POINT('Ctrl Pts',(9.59060434300129,1.59841338882536,-4.91789113187562));
#41606=CARTESIAN_POINT('Ctrl Pts',(9.74970421526597,5.00143481089275,-1.31386010630501));
#41607=CARTESIAN_POINT('Ctrl Pts',(9.90880408753063,3.80907230476851,3.49736282416303));
#41608=CARTESIAN_POINT('Ctrl Pts',(10.0679039597953,-0.883115813962409,
5.09516290273885));
#41609=CARTESIAN_POINT('Ctrl Pts',(10.22700383206,-4.76388553535737,2.01146045261232));
#41610=CARTESIAN_POINT('Ctrl Pts',(10.3861037043246,-4.26753471994517,-2.92039825401031));
#41611=CARTESIAN_POINT('Ctrl Pts',(10.5452035765893,0.149882990889038,-5.1689567258239));
#41612=CARTESIAN_POINT('Ctrl Pts',(10.704303448854,4.42958624251035,-2.66820993668828));
#41613=CARTESIAN_POINT('Ctrl Pts',(10.8634033211187,4.63932753487269,2.28412315339565));
#41614=CARTESIAN_POINT('Ctrl Pts',(11.0225031933833,0.586393813370393,5.13777391729214));
#41615=CARTESIAN_POINT('Ctrl Pts',(11.181603065648,-4.00532623396138,3.27077059848325));
#41616=CARTESIAN_POINT('Ctrl Pts',(11.3407029379126,-4.91689999117348,-1.60145967239454));
#41617=CARTESIAN_POINT('Ctrl Pts',(11.4998028101773,-1.31076150706236,-5.00224776370858));
#41618=CARTESIAN_POINT('Ctrl Pts',(11.658902682442,3.49972182018105,-3.80690501300621));
#41619=CARTESIAN_POINT('Ctrl Pts',(11.8180025547066,5.09461487296727,0.886272086847998));
#41620=CARTESIAN_POINT('Ctrl Pts',(11.9771024269713,2.00850883058607,4.76513062511062));
#41621=CARTESIAN_POINT('Ctrl Pts',(12.136202299236,-2.92304128095414,4.26572488890354));
#41622=CARTESIAN_POINT('Ctrl Pts',(12.2953021715007,-5.16886309007812,-0.153085358464505));
#41623=CARTESIAN_POINT('Ctrl Pts',(12.4544020437653,-2.66546494290799,-4.43123778702695));
#41624=CARTESIAN_POINT('Ctrl Pts',(12.61350191603,2.28699597084696,-4.63791267903968));
#41625=CARTESIAN_POINT('Ctrl Pts',(12.7726017882947,5.13813765686258,-0.583208933669766));
#41626=CARTESIAN_POINT('Ctrl Pts',(12.9317016605593,3.2682859109503,4.00734790289743));
#41627=CARTESIAN_POINT('Ctrl Pts',(13.090801532824,-1.60449996642509,4.91591419297749));
#41628=CARTESIAN_POINT('Ctrl Pts',(13.2499014050887,-5.00306910342174,1.30764854213172));
#41629=CARTESIAN_POINT('Ctrl Pts',(13.4090012773533,-3.80471649711291,-3.50205289112016));
#41630=CARTESIAN_POINT('Ctrl Pts',(13.568101149618,0.889390123239341,-5.09411585972022));
#41631=CARTESIAN_POINT('Ctrl Pts',(13.7272010218827,4.7664465535393,-2.00545869799919));
#41632=CARTESIAN_POINT('Ctrl Pts',(13.8863008941473,4.26377407797028,2.92549576490892));
#41633=CARTESIAN_POINT('Ctrl Pts',(14.045400766412,-0.156020461739612,5.16912688108217));
#41634=CARTESIAN_POINT('Ctrl Pts',(14.2045006386767,-4.43340011533161,2.66202951501289));
#41635=CARTESIAN_POINT('Ctrl Pts',(14.3636005109413,-4.63551232968508,-2.28854382581323));
#41636=CARTESIAN_POINT('Ctrl Pts',(14.522700383206,-0.581919347715841,-5.1410577240212));
#41637=CARTESIAN_POINT('Ctrl Pts',(14.6818002554707,4.01308660375755,-3.2607181841902));
#41638=CARTESIAN_POINT('Ctrl Pts',(14.8143834823579,4.75806562994111,0.786704444467226));
#41639=CARTESIAN_POINT('Ctrl Pts',(14.9204500638677,3.11408383257965,3.31830903713004));
#41640=CARTESIAN_POINT('Ctrl Pts',(14.9734833546226,1.80781376844615,4.04682358287313));
#41641=CARTESIAN_POINT('Ctrl Pts',(15.,1.10295997362678,4.23058663740352));
#41642=CARTESIAN_POINT('Ctrl Pts',(2.22260689770794,-2.00237954638876,4.09906332620075));
#41643=CARTESIAN_POINT('Ctrl Pts',(2.24912354308539,-2.68532037429503,3.76544887910198));
#41644=CARTESIAN_POINT('Ctrl Pts',(2.30215683384027,-3.87080614621125,2.75038105804722));
#41645=CARTESIAN_POINT('Ctrl Pts',(2.40822341535006,-5.02907715778026,-0.178658710094689));
#41646=CARTESIAN_POINT('Ctrl Pts',(2.54080664223727,-3.43068896545911,-4.16436342244229));
#41647=CARTESIAN_POINT('Ctrl Pts',(2.69990651450196,1.65762077157099,-5.13796052424968));
#41648=CARTESIAN_POINT('Ctrl Pts',(2.8590063867666,5.21409784376103,-1.38273310829352));
#41649=CARTESIAN_POINT('Ctrl Pts',(3.01810625903129,3.98430482800797,3.63889215410996));
#41650=CARTESIAN_POINT('Ctrl Pts',(3.17720613129595,-0.908664557549035,
5.3191704066765));
#41651=CARTESIAN_POINT('Ctrl Pts',(3.33630600356062,-4.96551905943183,2.11102334806669));
#41652=CARTESIAN_POINT('Ctrl Pts',(3.49540587582528,-4.46062666336713,-3.03618522036417));
#41653=CARTESIAN_POINT('Ctrl Pts',(3.65450574808995,0.143080314496841,-5.39400653083915));
#41654=CARTESIAN_POINT('Ctrl Pts',(3.81360562035462,4.61514993964848,-2.79558764496926));
#41655=CARTESIAN_POINT('Ctrl Pts',(3.97270549261929,4.84684961235789,2.3713723801698));
#41656=CARTESIAN_POINT('Ctrl Pts',(4.13180536488395,0.625153138376691,5.35952683456545));
#41657=CARTESIAN_POINT('Ctrl Pts',(4.29090523714863,-4.17091766469395,3.42325555365425));
#41658=CARTESIAN_POINT('Ctrl Pts',(4.45000510941329,-5.13470740781455,-1.65833629147738));
#41659=CARTESIAN_POINT('Ctrl Pts',(4.60910498167796,-1.38065392780811,-5.2162330189771));
#41660=CARTESIAN_POINT('Ctrl Pts',(4.76820485394262,3.64195901082506,-3.98138326368112));
#41661=CARTESIAN_POINT('Ctrl Pts',(4.92730472620729,5.31829404195296,0.911612035230917));
#41662=CARTESIAN_POINT('Ctrl Pts',(5.08640459847196,2.10810977781265,4.96700708957871));
#41663=CARTESIAN_POINT('Ctrl Pts',(5.24550447073663,-3.03903291634182,4.45865041205641));
#41664=CARTESIAN_POINT('Ctrl Pts',(5.4046043430013,-5.39387254956214,-0.146372533690109));
#41665=CARTESIAN_POINT('Ctrl Pts',(5.56370421526596,-2.79275117663017,-4.61690659614762));
#41666=CARTESIAN_POINT('Ctrl Pts',(5.72280408753063,2.3743865510322,-4.84536623628618));
#41667=CARTESIAN_POINT('Ctrl Pts',(5.8819039597953,5.35990679778392,-0.621839835308898));
#41668=CARTESIAN_POINT('Ctrl Pts',(6.04100383205997,3.42067433217443,4.17304118272146));
#41669=CARTESIAN_POINT('Ctrl Pts',(6.20010370432463,-1.66151858265413,5.1336771985115));
#41670=CARTESIAN_POINT('Ctrl Pts',(6.35920357658931,-5.21708642809535,1.37742324986404));
#41671=CARTESIAN_POINT('Ctrl Pts',(6.51830344885397,-3.9791268071616,-3.64442525640584));
#41672=CARTESIAN_POINT('Ctrl Pts',(6.67740332111864,0.914906733015021,-5.31772801721321));
#41673=CARTESIAN_POINT('Ctrl Pts',(6.83650319338331,4.96831196311641,-2.1050325024112));
#41674=CARTESIAN_POINT('Ctrl Pts',(6.99560306564798,4.45676697176347,3.04179449614205));
#41675=CARTESIAN_POINT('Ctrl Pts',(7.15470293791264,-0.149713990408975,
5.3937807999895));
#41676=CARTESIAN_POINT('Ctrl Pts',(7.31380281017731,-4.61863577389657,2.78989053295287));
#41677=CARTESIAN_POINT('Ctrl Pts',(7.47290268244198,-4.84389440702522,-2.37738776204113));
#41678=CARTESIAN_POINT('Ctrl Pts',(7.63200255470664,-0.618519302134332,
-5.36029098747527));
#41679=CARTESIAN_POINT('Ctrl Pts',(7.79110242697132,4.17515945318134,-3.41808852110343));
#41680=CARTESIAN_POINT('Ctrl Pts',(7.95020229923597,5.13264692052304,1.66469852729966));
#41681=CARTESIAN_POINT('Ctrl Pts',(8.10930217150066,1.37419105168933,5.21793872626056));
#41682=CARTESIAN_POINT('Ctrl Pts',(8.26840204376531,-3.64688958623763,3.9768683588161));
#41683=CARTESIAN_POINT('Ctrl Pts',(8.42750191602999,-5.31716022138873,-0.91820083730981));
#41684=CARTESIAN_POINT('Ctrl Pts',(8.58660178829464,-2.10195427852144,-4.96961505637633));
#41685=CARTESIAN_POINT('Ctrl Pts',(8.74570166055932,3.04455483525227,-4.4548817551871));
#41686=CARTESIAN_POINT('Ctrl Pts',(8.90480153282398,5.39368701870719,0.153055355295186));
#41687=CARTESIAN_POINT('Ctrl Pts',(9.06390140508865,2.7870287986572,4.62036319708922));
#41688=CARTESIAN_POINT('Ctrl Pts',(9.22300127735332,-2.38038805028225,4.84242070948262));
#41689=CARTESIAN_POINT('Ctrl Pts',(9.38210114961799,-5.36067312548293,0.615198536468943));
#41690=CARTESIAN_POINT('Ctrl Pts',(9.54120102188265,-3.41550139545205,-4.17727612389385));
#41691=CARTESIAN_POINT('Ctrl Pts',(9.70030089414733,1.6678778316151,-5.13161467145851));
#41692=CARTESIAN_POINT('Ctrl Pts',(9.85940076641199,5.21878902271104,-1.37095832684435));
#41693=CARTESIAN_POINT('Ctrl Pts',(10.0185006386767,3.97460838388701,3.64935251688739));
#41694=CARTESIAN_POINT('Ctrl Pts',(10.1776005109413,-0.921494589043101,
5.31659038478835));
#41695=CARTESIAN_POINT('Ctrl Pts',(10.336700383206,-4.97091624252066,2.09887524812842));
#41696=CARTESIAN_POINT('Ctrl Pts',(10.4958002554707,-4.45299482900043,-3.04731400612877));
#41697=CARTESIAN_POINT('Ctrl Pts',(10.6549001277353,0.156396661581818,-5.39359116724809));
#41698=CARTESIAN_POINT('Ctrl Pts',(10.814,4.62208884682804,-2.78416599523604));
#41699=CARTESIAN_POINT('Ctrl Pts',(10.9730998722647,4.84094515418326,2.38338742584421));
#41700=CARTESIAN_POINT('Ctrl Pts',(11.1321997445293,0.611877533530606,5.36105320464015));
#41701=CARTESIAN_POINT('Ctrl Pts',(11.291299616794,-4.17939118923417,3.4129129620953));
#41702=CARTESIAN_POINT('Ctrl Pts',(11.4503994890587,-5.13058045739557,-1.67105650170719));
#41703=CARTESIAN_POINT('Ctrl Pts',(11.6094993613233,-1.36772506752482,-5.21963730513232));
#41704=CARTESIAN_POINT('Ctrl Pts',(11.768599233588,3.65181403103062,-3.97234690515425));
#41705=CARTESIAN_POINT('Ctrl Pts',(11.9276991058527,5.31601853853538,0.924788028408167));
#41706=CARTESIAN_POINT('Ctrl Pts',(12.0867989781174,2.09579535341577,4.9722154418469));
#41707=CARTESIAN_POINT('Ctrl Pts',(12.245898850382,-3.05007189471929,4.45110634564912));
#41708=CARTESIAN_POINT('Ctrl Pts',(12.4049987226467,-5.39349346224528,-0.159738198836918));
#41709=CARTESIAN_POINT('Ctrl Pts',(12.5640985949113,-2.78130170849642,-4.62381216477972));
#41710=CARTESIAN_POINT('Ctrl Pts',(12.723198467176,2.38638509126345,-4.83946881101991));
#41711=CARTESIAN_POINT('Ctrl Pts',(12.8822983394407,5.36143275173995,-0.608554244144905));
#41712=CARTESIAN_POINT('Ctrl Pts',(13.0413982117054,3.41032029408859,4.18150071660979));
#41713=CARTESIAN_POINT('Ctrl Pts',(13.20049808397,-1.67422892196505,5.1295518180154));
#41714=CARTESIAN_POINT('Ctrl Pts',(13.3595979562347,-5.22049433893182,1.36447681820791));
#41715=CARTESIAN_POINT('Ctrl Pts',(13.5186978284993,-3.97006327992432,-3.6542464065165));
#41716=CARTESIAN_POINT('Ctrl Pts',(13.677797700764,0.928041569583217,-5.31549783898529));
#41717=CARTESIAN_POINT('Ctrl Pts',(13.8368975730287,4.97358855838203,-2.09261266703394));
#41718=CARTESIAN_POINT('Ctrl Pts',(13.9959974452933,4.4490707556497,3.05263304654951));
#41719=CARTESIAN_POINT('Ctrl Pts',(14.155097317558,-0.162800856920419,5.39376871717677));
#41720=CARTESIAN_POINT('Ctrl Pts',(14.3141971898227,-4.62606846435103,2.77771698249975));
#41721=CARTESIAN_POINT('Ctrl Pts',(14.4732970620874,-4.83696414639145,-2.3880002134858));
#41722=CARTESIAN_POINT('Ctrl Pts',(14.632396934352,-0.607208614885573,-5.36447972026183));
#41723=CARTESIAN_POINT('Ctrl Pts',(14.7914968066167,4.18748881206356,-3.40242368624789));
#41724=CARTESIAN_POINT('Ctrl Pts',(14.9240800335039,4.96484341349299,0.820893338439942));
#41725=CARTESIAN_POINT('Ctrl Pts',(15.0301466150137,3.24941684451702,3.46251734386715));
#41726=CARTESIAN_POINT('Ctrl Pts',(15.0831799057686,1.88637841071624,4.22269194534932));
#41727=CARTESIAN_POINT('Ctrl Pts',(15.109696551146,1.15089281786034,4.41444104296314));
#41728=CARTESIAN_POINT('Ctrl Pts',(2.33230344885397,-2.08577545033743,4.26978275451687));
#41729=CARTESIAN_POINT('Ctrl Pts',(2.35882009423142,-2.7971596709009,3.92227379953806));
#41730=CARTESIAN_POINT('Ctrl Pts',(2.4118533849863,-4.03201902823232,2.8649300280229));
#41731=CARTESIAN_POINT('Ctrl Pts',(2.51791996649609,-5.23853017399645,-0.186099559484853));
#41732=CARTESIAN_POINT('Ctrl Pts',(2.6505031933833,-3.57357167116653,-4.33780249527526));
#41733=CARTESIAN_POINT('Ctrl Pts',(2.80960306564798,1.72665802422299,-5.35194835844684));
#41734=CARTESIAN_POINT('Ctrl Pts',(2.96870293791264,5.43125667548277,-1.44032172963851));
#41735=CARTESIAN_POINT('Ctrl Pts',(3.12780281017732,4.15024474850808,3.79044618946306));
#41736=CARTESIAN_POINT('Ctrl Pts',(3.28690268244198,-0.946508982348298,
5.54070534250915));
#41737=CARTESIAN_POINT('Ctrl Pts',(3.44600255470665,-5.1723249825559,2.19894409250613));
#41738=CARTESIAN_POINT('Ctrl Pts',(3.60510242697131,-4.6464046261115,-3.16263747636354));
#41739=CARTESIAN_POINT('Ctrl Pts',(3.76420229923598,0.149039380642027,-5.61865827149225));
#41740=CARTESIAN_POINT('Ctrl Pts',(3.92330217150065,4.80736354958561,-2.91201939695178));
#41741=CARTESIAN_POINT('Ctrl Pts',(4.08240204376532,5.04871314290327,2.4701362451922));
#41742=CARTESIAN_POINT('Ctrl Pts',(4.24150191602998,0.651189766235444,5.58274255104231));
#41743=CARTESIAN_POINT('Ctrl Pts',(4.40060178829465,-4.34462971122875,3.56582866965477));
#41744=CARTESIAN_POINT('Ctrl Pts',(4.55970166055932,-5.34855975491775,-1.72740334438853));
#41745=CARTESIAN_POINT('Ctrl Pts',(4.71880153282399,-1.43815595461293,-5.43348077732993));
#41746=CARTESIAN_POINT('Ctrl Pts',(4.87790140508865,3.79364077585284,-4.14720150570204));
#41747=CARTESIAN_POINT('Ctrl Pts',(5.03700127735333,5.53979247859722,0.949579217759153));
#41748=CARTESIAN_POINT('Ctrl Pts',(5.19610114961799,2.19590917671323,5.17387498677729));
#41749=CARTESIAN_POINT('Ctrl Pts',(5.35520102188265,-3.16560377432185,4.64434606709603));
#41750=CARTESIAN_POINT('Ctrl Pts',(5.51430089414734,-5.61851871010945,-0.152468715496564));
#41751=CARTESIAN_POINT('Ctrl Pts',(5.67340076641199,-2.9090647942452,-4.80919336801698));
#41752=CARTESIAN_POINT('Ctrl Pts',(5.83250063867666,2.47327595144782,-5.04716798659183));
#41753=CARTESIAN_POINT('Ctrl Pts',(5.99160051094134,5.58313833912081,-0.647738469396749));
#41754=CARTESIAN_POINT('Ctrl Pts',(6.15070038320599,3.56313994443072,4.34684167038412));
#41755=CARTESIAN_POINT('Ctrl Pts',(6.30980025547067,-1.73071817290056,5.34748663904573));
#41756=CARTESIAN_POINT('Ctrl Pts',(6.46890012773532,-5.43436972957236,1.43479072410215));
#41757=CARTESIAN_POINT('Ctrl Pts',(6.62800000000001,-4.14485107137922,-3.79620973661563));
#41758=CARTESIAN_POINT('Ctrl Pts',(6.78709987226466,0.953011134433869,-5.53920287983279));
#41759=CARTESIAN_POINT('Ctrl Pts',(6.94619974452934,5.17523420620982,-2.19270373771549));
#41760=CARTESIAN_POINT('Ctrl Pts',(7.10529961679399,4.64238418452872,3.16848036950175));
#41761=CARTESIAN_POINT('Ctrl Pts',(7.26439948905868,-0.155949338540855,
5.61842313931392));
#41762=CARTESIAN_POINT('Ctrl Pts',(7.42349936132333,-4.81099456325219,2.90608500933629));
#41763=CARTESIAN_POINT('Ctrl Pts',(7.58259923358801,-5.04563485799734,-2.47640215809281));
#41764=CARTESIAN_POINT('Ctrl Pts',(7.74169910585267,-0.644279641328896,
-5.58353852969804));
#41765=CARTESIAN_POINT('Ctrl Pts',(7.90079897811735,4.34904816341905,-3.56044643846636));
#41766=CARTESIAN_POINT('Ctrl Pts',(8.05989885038201,5.34641345162768,1.73403055715211));
#41767=CARTESIAN_POINT('Ctrl Pts',(8.21899872264668,1.43142391004554,5.43525752459233));
#41768=CARTESIAN_POINT('Ctrl Pts',(8.37809859491134,-3.79877670184155,4.14249856227404));
#41769=CARTESIAN_POINT('Ctrl Pts',(8.53719846717601,-5.53861143622079,-0.95644243290139));
#41770=CARTESIAN_POINT('Ctrl Pts',(8.69629833944068,-2.18949731072642,-5.17659157121883));
#41771=CARTESIAN_POINT('Ctrl Pts',(8.85539821170535,3.17135567231888,-4.64042045169863));
#41772=CARTESIAN_POINT('Ctrl Pts',(9.01449808397001,5.61832545219127,0.159429865927808));
#41773=CARTESIAN_POINT('Ctrl Pts',(9.17359795623469,2.90310408838647,4.81279393085663));
#41774=CARTESIAN_POINT('Ctrl Pts',(9.33269782849934,-2.47952740353819,5.04409978331027));
#41775=CARTESIAN_POINT('Ctrl Pts',(9.49179770076403,-5.58393658314223,0.640820571087352));
#41776=CARTESIAN_POINT('Ctrl Pts',(9.65089757302868,-3.55775156317145,-4.35125299007969));
#41777=CARTESIAN_POINT('Ctrl Pts',(9.80999744529336,1.73734227440484,-5.34533821104139));
#41778=CARTESIAN_POINT('Ctrl Pts',(9.96909731755802,5.43614323452935,-1.42805654738371));
#41779=CARTESIAN_POINT('Ctrl Pts',(10.1281971898227,4.1401444630055,3.80134220961176));
#41780=CARTESIAN_POINT('Ctrl Pts',(10.2872970620874,-0.959873364123795,
5.53801786683784));
#41781=CARTESIAN_POINT('Ctrl Pts',(10.446396934352,-5.17794694968394,2.18629004364453));
#41782=CARTESIAN_POINT('Ctrl Pts',(10.6054968066167,-4.6384549380557,-3.17422975824723));
#41783=CARTESIAN_POINT('Ctrl Pts',(10.7645966788814,0.162910332274605,-5.61822560867227));
#41784=CARTESIAN_POINT('Ctrl Pts',(10.923696551146,4.81459145114573,-2.90012205378381));
#41785=CARTESIAN_POINT('Ctrl Pts',(11.0827964234107,5.04256277349384,2.48265169829277));
#41786=CARTESIAN_POINT('Ctrl Pts',(11.2418962956754,0.637361253690814,5.58433249198815));
#41787=CARTESIAN_POINT('Ctrl Pts',(11.40099616794,-4.35345614450695,3.55505532570735));
#41788=CARTESIAN_POINT('Ctrl Pts',(11.5600960402047,-5.34426092361766,-1.74065333101984));
#41789=CARTESIAN_POINT('Ctrl Pts',(11.7191959124694,-1.42468862798729,-5.43702684655607));
#41790=CARTESIAN_POINT('Ctrl Pts',(11.878295784734,3.8039062418802,-4.13778879730229));
#41791=CARTESIAN_POINT('Ctrl Pts',(12.0373956569987,5.53742220410349,0.963303969968333));
#41792=CARTESIAN_POINT('Ctrl Pts',(12.1964955292634,2.18308187624546,5.17930025858317));
#41793=CARTESIAN_POINT('Ctrl Pts',(12.355595401528,-3.17710250848444,4.63648780239471));
#41794=CARTESIAN_POINT('Ctrl Pts',(12.5146952737927,-5.61812383441245,-0.166391039209329));
#41795=CARTESIAN_POINT('Ctrl Pts',(12.6737951460574,-2.89713847408484,-4.81638654253248));
#41796=CARTESIAN_POINT('Ctrl Pts',(12.832895018322,2.48577421167993,-5.04102494300014));
#41797=CARTESIAN_POINT('Ctrl Pts',(12.9919948905867,5.58472784661733,-0.63389955462005));
#41798=CARTESIAN_POINT('Ctrl Pts',(13.1510947628514,3.55235467722688,4.35565353032216));
#41799=CARTESIAN_POINT('Ctrl Pts',(13.3101946351161,-1.74395787750501,5.34318944305331));
#41800=CARTESIAN_POINT('Ctrl Pts',(13.4692945073807,-5.43791957444192,1.4213050942841));
#41801=CARTESIAN_POINT('Ctrl Pts',(13.6283943796454,-4.13541006273573,-3.80643992191284));
#41802=CARTESIAN_POINT('Ctrl Pts',(13.7874942519101,0.966693015927084,-5.53687981825035));
#41803=CARTESIAN_POINT('Ctrl Pts',(13.9465941241747,5.18073056322477,-2.17976663606868));
#41804=CARTESIAN_POINT('Ctrl Pts',(14.1056939964394,4.63436743332911,3.17977032819009));
#41805=CARTESIAN_POINT('Ctrl Pts',(14.264793868704,-0.169581252101216,5.61841055327138));
#41806=CARTESIAN_POINT('Ctrl Pts',(14.4238937409687,-4.81873681337047,2.89340444998659));
#41807=CARTESIAN_POINT('Ctrl Pts',(14.5829936132334,-5.0384159630978,-2.48745660115836));
#41808=CARTESIAN_POINT('Ctrl Pts',(14.7420934854981,-0.63249788205531,-5.58790171650246));
#41809=CARTESIAN_POINT('Ctrl Pts',(14.9011933577627,4.36189102036958,-3.54412918830557));
#41810=CARTESIAN_POINT('Ctrl Pts',(15.0337765846499,5.17162119704487,0.855082232412658));
#41811=CARTESIAN_POINT('Ctrl Pts',(15.1398431661597,3.38474985645439,3.60672565060427));
#41812=CARTESIAN_POINT('Ctrl Pts',(15.1928764569146,1.96494305298632,4.3985603078255));
#41813=CARTESIAN_POINT('Ctrl Pts',(15.2193931022921,1.19882566209391,4.59829544852276));
#41814=CARTESIAN_POINT('Ctrl Pts',(2.442,-2.16917135428609,4.440502182833));
#41815=CARTESIAN_POINT('Ctrl Pts',(2.46851664537744,-2.90899896750678,4.07909871997414));
#41816=CARTESIAN_POINT('Ctrl Pts',(2.52154993613233,-4.19323191025339,2.97947899799857));
#41817=CARTESIAN_POINT('Ctrl Pts',(2.62761651764211,-5.44798319021263,-0.193540408875019));
#41818=CARTESIAN_POINT('Ctrl Pts',(2.76019974452933,-3.71645437687396,-4.51124156810822));
#41819=CARTESIAN_POINT('Ctrl Pts',(2.919299616794,1.795695276875,-5.565936192644));
#41820=CARTESIAN_POINT('Ctrl Pts',(3.07839948905867,5.64841550720451,-1.4979103509835));
#41821=CARTESIAN_POINT('Ctrl Pts',(3.23749936132334,4.31618466900822,3.94200022481617));
#41822=CARTESIAN_POINT('Ctrl Pts',(3.39659923358801,-0.984353407147573,
5.7622402783418));
#41823=CARTESIAN_POINT('Ctrl Pts',(3.55569910585267,-5.37913090567997,2.28686483694558));
#41824=CARTESIAN_POINT('Ctrl Pts',(3.71479897811734,-4.83218258885587,-3.28908973236292));
#41825=CARTESIAN_POINT('Ctrl Pts',(3.87389885038201,0.154998446787216,-5.84331001214534));
#41826=CARTESIAN_POINT('Ctrl Pts',(4.03299872264668,4.99957715952273,-3.02845114893429));
#41827=CARTESIAN_POINT('Ctrl Pts',(4.19209859491135,5.25057667344865,2.5689001102146));
#41828=CARTESIAN_POINT('Ctrl Pts',(4.35119846717601,0.677226394094196,5.80595826751917));
#41829=CARTESIAN_POINT('Ctrl Pts',(4.51029833944069,-4.51834175776356,3.70840178565529));
#41830=CARTESIAN_POINT('Ctrl Pts',(4.66939821170534,-5.56241210202095,-1.79647039729968));
#41831=CARTESIAN_POINT('Ctrl Pts',(4.82849808397002,-1.49565798141775,-5.65072853568276));
#41832=CARTESIAN_POINT('Ctrl Pts',(4.98759795623469,3.94532254088061,-4.31301974772297));
#41833=CARTESIAN_POINT('Ctrl Pts',(5.14669782849935,5.76129091524147,0.987546400287391));
#41834=CARTESIAN_POINT('Ctrl Pts',(5.30579770076402,2.28370857561381,5.38074288397587));
#41835=CARTESIAN_POINT('Ctrl Pts',(5.46489757302869,-3.29217463230187,4.83004172213565));
#41836=CARTESIAN_POINT('Ctrl Pts',(5.62399744529335,-5.84316487065676,-0.158564897303022));
#41837=CARTESIAN_POINT('Ctrl Pts',(5.78309731755803,-3.02537841186024,-5.00148013988634));
#41838=CARTESIAN_POINT('Ctrl Pts',(5.94219718982269,2.57216535186344,-5.24896973689749));
#41839=CARTESIAN_POINT('Ctrl Pts',(6.10129706208736,5.80636988045771,-0.67363710348459));
#41840=CARTESIAN_POINT('Ctrl Pts',(6.26039693435203,3.70560555668701,4.52064215804677));
#41841=CARTESIAN_POINT('Ctrl Pts',(6.41949680661669,-1.79991776314699,5.56129607957998));
#41842=CARTESIAN_POINT('Ctrl Pts',(6.57859667888136,-5.65165303104936,1.49215819834025));
#41843=CARTESIAN_POINT('Ctrl Pts',(6.73769655114604,-4.31057533559683,-3.94799421682542));
#41844=CARTESIAN_POINT('Ctrl Pts',(6.89679642341068,0.991115535852721,-5.76067774245237));
#41845=CARTESIAN_POINT('Ctrl Pts',(7.05589629567538,5.38215644930322,-2.28037497301978));
#41846=CARTESIAN_POINT('Ctrl Pts',(7.21499616794003,4.82800139729398,3.29516624286144));
#41847=CARTESIAN_POINT('Ctrl Pts',(7.3740960402047,-0.162184686672736,5.84306547863835));
#41848=CARTESIAN_POINT('Ctrl Pts',(7.53319591246937,-5.0033533526078,3.02227948571969));
#41849=CARTESIAN_POINT('Ctrl Pts',(7.69229578473404,-5.24737530896947,-2.57541655414449));
#41850=CARTESIAN_POINT('Ctrl Pts',(7.8513956569987,-0.670039980523453,-5.80678607192081));
#41851=CARTESIAN_POINT('Ctrl Pts',(8.01049552926337,4.52293687365675,-3.7028043558293));
#41852=CARTESIAN_POINT('Ctrl Pts',(8.16959540152804,5.56017998273234,1.80336258700456));
#41853=CARTESIAN_POINT('Ctrl Pts',(8.32869527379271,1.48865676840175,5.65257632292408));
#41854=CARTESIAN_POINT('Ctrl Pts',(8.48779514605737,-3.95066381744548,4.30812876573197));
#41855=CARTESIAN_POINT('Ctrl Pts',(8.64689501832204,-5.76006265105285,-0.994684028492972));
#41856=CARTESIAN_POINT('Ctrl Pts',(8.80599489058671,-2.27704034293141,-5.38356808606133));
#41857=CARTESIAN_POINT('Ctrl Pts',(8.96509476285137,3.2981565093855,-4.82595914821016));
#41858=CARTESIAN_POINT('Ctrl Pts',(9.12419463511605,5.84296388567535,0.165804376560428));
#41859=CARTESIAN_POINT('Ctrl Pts',(9.2832945073807,3.01917937811574,5.00522466462404));
#41860=CARTESIAN_POINT('Ctrl Pts',(9.44239437964538,-2.57866675679413,5.24577885713792));
#41861=CARTESIAN_POINT('Ctrl Pts',(9.60149425191005,-5.80720004080153,0.666442605705756));
#41862=CARTESIAN_POINT('Ctrl Pts',(9.7605941241747,-3.70000173089087,-4.52522985626553));
#41863=CARTESIAN_POINT('Ctrl Pts',(9.9196939964394,1.80680671719459,-5.55906175062428));
#41864=CARTESIAN_POINT('Ctrl Pts',(10.078793868704,5.65349744634764,-1.48515476792305));
#41865=CARTESIAN_POINT('Ctrl Pts',(10.2378937409687,4.305680542124,3.95333190233613));
#41866=CARTESIAN_POINT('Ctrl Pts',(10.3969936132334,-0.998252139204486,
5.75944534888733));
#41867=CARTESIAN_POINT('Ctrl Pts',(10.5560934854981,-5.38497765684723,2.27370483916063));
#41868=CARTESIAN_POINT('Ctrl Pts',(10.7151933577627,-4.82391504711097,-3.30114551036569));
#41869=CARTESIAN_POINT('Ctrl Pts',(10.8742932300274,0.169424002967387,-5.84286005009646));
#41870=CARTESIAN_POINT('Ctrl Pts',(11.033393102292,5.00709405546342,-3.01607811233158));
#41871=CARTESIAN_POINT('Ctrl Pts',(11.1924929745567,5.24418039280442,2.58191597074134));
#41872=CARTESIAN_POINT('Ctrl Pts',(11.3515928468214,0.662844973851022,5.80761177933616));
#41873=CARTESIAN_POINT('Ctrl Pts',(11.5106927190861,-4.52752109977973,3.6971976893194));
#41874=CARTESIAN_POINT('Ctrl Pts',(11.6697925913507,-5.55794138983975,-1.81025016033249));
#41875=CARTESIAN_POINT('Ctrl Pts',(11.8288924636154,-1.48165218844976,-5.65441638797981));
#41876=CARTESIAN_POINT('Ctrl Pts',(11.9879923358801,3.95599845272978,-4.30323068945033));
#41877=CARTESIAN_POINT('Ctrl Pts',(12.1470922081447,5.75882586967161,1.0018199115285));
#41878=CARTESIAN_POINT('Ctrl Pts',(12.3061920804094,2.27036839907515,5.38638507531945));
#41879=CARTESIAN_POINT('Ctrl Pts',(12.4652919526741,-3.30413312224959,4.8218692591403));
#41880=CARTESIAN_POINT('Ctrl Pts',(12.6243918249387,-5.84275420657962,-0.173043879581744));
#41881=CARTESIAN_POINT('Ctrl Pts',(12.7834916972034,-3.01297523967326,-5.00896092028525));
#41882=CARTESIAN_POINT('Ctrl Pts',(12.9425915694681,2.58516333209641,-5.24258107498037));
#41883=CARTESIAN_POINT('Ctrl Pts',(13.1016914417327,5.80802294149471,-0.659244865095191));
#41884=CARTESIAN_POINT('Ctrl Pts',(13.2607913139974,3.69438906036517,4.52980634403453));
#41885=CARTESIAN_POINT('Ctrl Pts',(13.4198911862621,-1.81368683304497,5.55682706809122));
#41886=CARTESIAN_POINT('Ctrl Pts',(13.5789910585268,-5.655344809952,1.47813337036028));
#41887=CARTESIAN_POINT('Ctrl Pts',(13.7380909307914,-4.30075684554715,-3.95863343730917));
#41888=CARTESIAN_POINT('Ctrl Pts',(13.8971908030561,1.00534446227096,-5.75826179751541));
#41889=CARTESIAN_POINT('Ctrl Pts',(14.0562906753207,5.38787256806751,-2.26692060510343));
#41890=CARTESIAN_POINT('Ctrl Pts',(14.2153905475854,4.81966411100853,3.30690760983067));
#41891=CARTESIAN_POINT('Ctrl Pts',(14.3744904198501,-0.176361647282018,
5.84305238936599));
#41892=CARTESIAN_POINT('Ctrl Pts',(14.5335902921148,-5.01140516238991,3.00909191747344));
#41893=CARTESIAN_POINT('Ctrl Pts',(14.6926901643794,-5.23986777980416,-2.58691298883092));
#41894=CARTESIAN_POINT('Ctrl Pts',(14.8517900366441,-0.657787149225042,
-5.81132371274309));
#41895=CARTESIAN_POINT('Ctrl Pts',(15.0108899089088,4.53629322867559,-3.68583469036325));
#41896=CARTESIAN_POINT('Ctrl Pts',(15.143473135796,5.37839898059675,0.889271126385368));
#41897=CARTESIAN_POINT('Ctrl Pts',(15.2495397173057,3.52008286839176,3.75093395734139));
#41898=CARTESIAN_POINT('Ctrl Pts',(15.3025730080606,2.04350769525641,4.57442867030168));
#41899=CARTESIAN_POINT('Ctrl Pts',(15.3290896534381,1.24675850632747,4.78214985408238));
#41900=CARTESIAN_POINT('',(15.,3.61714728420828,-3.37770697643486));
#41901=CARTESIAN_POINT('Ctrl Pts',(15.,3.61714728420828,-3.37770697643486));
#41902=CARTESIAN_POINT('Ctrl Pts',(15.,3.68957840109089,-3.29192253111056));
#41903=CARTESIAN_POINT('Ctrl Pts',(15.,3.75871853092304,-3.20370683073969));
#41904=CARTESIAN_POINT('Ctrl Pts',(15.,3.82438207257458,-3.11313443623491));
#41905=CARTESIAN_POINT('Ctrl Pts',(15.,3.90791289962552,-2.99791696805269));
#41906=CARTESIAN_POINT('Ctrl Pts',(15.,3.98581952259522,-2.87888650317557));
#41907=CARTESIAN_POINT('Ctrl Pts',(15.,4.05811156137618,-2.75649539075295));
#41908=CARTESIAN_POINT('Ctrl Pts',(15.,4.13173944465282,-2.63184268083483));
#41909=CARTESIAN_POINT('Ctrl Pts',(15.,4.19954353035942,-2.50370321513495));
#41910=CARTESIAN_POINT('Ctrl Pts',(15.,4.26148524515888,-2.37253157027713));
#41911=CARTESIAN_POINT('Ctrl Pts',(15.,4.32381499703478,-2.24053819386494));
#41912=CARTESIAN_POINT('Ctrl Pts',(15.,4.38020882026663,-2.10547368153064));
#41913=CARTESIAN_POINT('Ctrl Pts',(15.,4.43057619978867,-1.96779009730298));
#41914=CARTESIAN_POINT('Ctrl Pts',(15.,4.45655213569676,-1.8967826318872));
#41915=CARTESIAN_POINT('Ctrl Pts',(15.,4.48092433553813,-1.8250784529312));
#41916=CARTESIAN_POINT('Ctrl Pts',(15.,4.50367494257293,-1.75273956196209));
#41917=CARTESIAN_POINT('Ctrl Pts',(15.,4.51067738059232,-1.730474283518));
#41918=CARTESIAN_POINT('Ctrl Pts',(15.,4.51752691038149,-1.70814614040682));
#41919=CARTESIAN_POINT('Ctrl Pts',(15.,4.52421615574277,-1.68578041462856));
#41920=CARTESIAN_POINT('Ctrl Pts',(15.,4.56556142875004,-1.54754104854681));
#41921=CARTESIAN_POINT('Ctrl Pts',(15.,4.6008467478143,-1.40768448094355));
#41922=CARTESIAN_POINT('Ctrl Pts',(15.,4.63006598166419,-1.26666139036611));
#41923=CARTESIAN_POINT('Ctrl Pts',(15.,4.65937480607125,-1.1252059018236));
#41924=CARTESIAN_POINT('Ctrl Pts',(15.,4.68258035315745,-0.982575874006902));
#41925=CARTESIAN_POINT('Ctrl Pts',(15.,4.69962490113214,-0.83921597561456));
#41926=CARTESIAN_POINT('Ctrl Pts',(15.,4.71652107743951,-0.697104015694111));
#41927=CARTESIAN_POINT('Ctrl Pts',(15.,4.72736302542697,-0.554274021959568));
#41928=CARTESIAN_POINT('Ctrl Pts',(15.,4.73204381389164,-0.41116162127756));
#41929=CARTESIAN_POINT('Ctrl Pts',(15.,4.73664109518138,-0.270602404181739));
#41930=CARTESIAN_POINT('Ctrl Pts',(15.,4.73529500312457,-0.129770054420742));
#41931=CARTESIAN_POINT('Ctrl Pts',(15.,4.72785605002238,0.010909094154732));
#41932=CARTESIAN_POINT('Ctrl Pts',(15.,4.72644560501024,0.037582229566991));
#41933=CARTESIAN_POINT('Ctrl Pts',(15.,4.72481598741633,0.0642497999003566));
#41934=CARTESIAN_POINT('Ctrl Pts',(15.,4.72296598198155,0.0909088105373209));
#41935=CARTESIAN_POINT('Ctrl Pts',(15.,4.72160216103772,0.110561789044773));
#41936=CARTESIAN_POINT('Ctrl Pts',(15.,4.72011835426907,0.130212130596743));
#41937=CARTESIAN_POINT('Ctrl Pts',(15.,4.71851563947719,0.149840943089536));
#41938=CARTESIAN_POINT('Ctrl Pts',(15.,4.70701478457874,0.290694528176004));
#41939=CARTESIAN_POINT('Ctrl Pts',(15.,4.68938349296752,0.430628932810751));
#41940=CARTESIAN_POINT('Ctrl Pts',(15.,4.66556557715506,0.569230026091733));
#41941=CARTESIAN_POINT('Ctrl Pts',(15.,4.64202084297191,0.706241422239518));
#41942=CARTESIAN_POINT('Ctrl Pts',(15.,4.61243051523659,0.841950655426112));
#41943=CARTESIAN_POINT('Ctrl Pts',(15.,4.57669086926763,0.975947063455624));
#41944=CARTESIAN_POINT('Ctrl Pts',(15.,4.54180219894916,1.10675296197131));
#41945=CARTESIAN_POINT('Ctrl Pts',(15.,4.50105340728844,1.23592722645281));
#41946=CARTESIAN_POINT('Ctrl Pts',(15.,4.45430240519226,1.36306795813444));
#41947=CARTESIAN_POINT('Ctrl Pts',(15.,4.44403793093735,1.39098249918347));
#41948=CARTESIAN_POINT('Ctrl Pts',(15.,4.43348394709866,1.41879891703032));
#41949=CARTESIAN_POINT('Ctrl Pts',(15.,4.42263865647625,1.44651278257324));
#41950=CARTESIAN_POINT('Ctrl Pts',(15.,4.38789959528659,1.53528437057554));
#41951=CARTESIAN_POINT('Ctrl Pts',(15.,4.35017225985734,1.62300434398871));
#41952=CARTESIAN_POINT('Ctrl Pts',(15.,4.30955405365424,1.70955383489484));
#41953=CARTESIAN_POINT('Ctrl Pts',(15.,4.28785544355993,1.75578934927581));
#41954=CARTESIAN_POINT('Ctrl Pts',(15.,4.26533170166485,1.80169070105758));
#41955=CARTESIAN_POINT('Ctrl Pts',(15.,4.24199681605842,1.84723878333485));
#41956=CARTESIAN_POINT('Ctrl Pts',(15.,4.23276596498054,1.86525676600147));
#41957=CARTESIAN_POINT('Ctrl Pts',(15.,4.22341148066082,1.8832129271299));
#41958=CARTESIAN_POINT('Ctrl Pts',(15.,4.21393845086224,1.9010989158475));
#41959=CARTESIAN_POINT('Ctrl Pts',(15.,4.15009794689424,2.02163590960511));
#41960=CARTESIAN_POINT('Ctrl Pts',(15.,4.08082383939265,2.13909255365038));
#41961=CARTESIAN_POINT('Ctrl Pts',(15.,4.00648273399672,2.25317473996996));
#41962=CARTESIAN_POINT('Ctrl Pts',(15.,3.93094927503506,2.36908668522197));
#41963=CARTESIAN_POINT('Ctrl Pts',(15.,3.85018442561141,2.48151572963273));
#41964=CARTESIAN_POINT('Ctrl Pts',(15.,3.76452857661151,2.59012356957856));
#41965=CARTESIAN_POINT('Ctrl Pts',(15.,3.67917632204047,2.69834646517415));
#41966=CARTESIAN_POINT('Ctrl Pts',(15.,3.58896700611038,2.80277576926211));
#41967=CARTESIAN_POINT('Ctrl Pts',(15.,3.49420334350769,2.90303817573571));
#41968=CARTESIAN_POINT('Ctrl Pts',(15.,3.43040339532139,2.97054017135684));
#41969=CARTESIAN_POINT('Ctrl Pts',(15.,3.36453840688444,3.03615263398548));
#41970=CARTESIAN_POINT('Ctrl Pts',(15.,3.29669428988104,3.09974975199444));
#41971=CARTESIAN_POINT('Ctrl Pts',(15.,3.2611435518308,3.13307503623351));
#41972=CARTESIAN_POINT('Ctrl Pts',(15.,3.2250493045892,3.16584677269137));
#41973=CARTESIAN_POINT('Ctrl Pts',(15.,3.18842348307835,3.19804567312667));
#41974=CARTESIAN_POINT('Ctrl Pts',(15.,3.17313594847647,3.2114854209396));
#41975=CARTESIAN_POINT('Ctrl Pts',(15.,3.15775579949857,3.22482535854092));
#41976=CARTESIAN_POINT('Ctrl Pts',(15.,3.14228389185458,3.23806403845506));
#41977=CARTESIAN_POINT('Ctrl Pts',(15.,3.12716082301245,3.25100423124363));
#41978=CARTESIAN_POINT('Ctrl Pts',(15.,3.1119569353217,3.26384180774895));
#41979=CARTESIAN_POINT('Ctrl Pts',(15.,3.09667494792814,3.276574287178));
#41980=CARTESIAN_POINT('Ctrl Pts',(15.,3.09356639373681,3.27916423842426));
#41981=CARTESIAN_POINT('Ctrl Pts',(15.,3.09045458489432,3.28174986078853));
#41982=CARTESIAN_POINT('Ctrl Pts',(15.,3.08733952984974,3.28433114559335));
#41983=CARTESIAN_POINT('Ctrl Pts',(15.,2.98213805185187,3.37150616263602));
#41984=CARTESIAN_POINT('Ctrl Pts',(15.,2.87323649961196,3.45373767302407));
#41985=CARTESIAN_POINT('Ctrl Pts',(15.,2.76096821108068,3.53084903830942));
#41986=CARTESIAN_POINT('Ctrl Pts',(15.,2.64885274757775,3.607855435872));
#41987=CARTESIAN_POINT('Ctrl Pts',(15.,2.53337902731004,3.67975592914996));
#41988=CARTESIAN_POINT('Ctrl Pts',(15.,2.41485687951612,3.74632782212485));
#41989=CARTESIAN_POINT('Ctrl Pts',(15.,2.36383379103652,3.77498663103725));
#41990=CARTESIAN_POINT('Ctrl Pts',(15.,2.31224553332968,3.80265729945555));
#41991=CARTESIAN_POINT('Ctrl Pts',(15.,2.26011603649344,3.82931916305926));
#41992=CARTESIAN_POINT('Ctrl Pts',(15.,2.23334563507941,3.8430110042324));
#41993=CARTESIAN_POINT('Ctrl Pts',(15.,2.20643249237716,3.85643677448972));
#41994=CARTESIAN_POINT('Ctrl Pts',(15.,2.17937981938905,3.8695934871651));
#41995=CARTESIAN_POINT('Ctrl Pts',(15.,2.15885041590124,3.87957769328051));
#41996=CARTESIAN_POINT('Ctrl Pts',(15.,2.13824932722211,3.889402721209));
#41997=CARTESIAN_POINT('Ctrl Pts',(15.,2.11758052897823,3.89906654384036));
#41998=CARTESIAN_POINT('Ctrl Pts',(15.,1.99606455224882,3.95588207961238));
#41999=CARTESIAN_POINT('Ctrl Pts',(15.,1.87218227454613,4.00714279893364));
#42000=CARTESIAN_POINT('Ctrl Pts',(15.,1.74623943949728,4.05264771511785));
#42001=CARTESIAN_POINT('Ctrl Pts',(15.,1.62228293761301,4.09743494121565));
#42002=CARTESIAN_POINT('Ctrl Pts',(15.,1.49632971967395,4.13664664515206));
#42003=CARTESIAN_POINT('Ctrl Pts',(15.,1.36866090588019,4.17004234853293));
#42004=CARTESIAN_POINT('Ctrl Pts',(15.,1.28087501187527,4.19300544805659));
#42005=CARTESIAN_POINT('Ctrl Pts',(15.,1.19227776673793,4.21321772214408));
#42006=CARTESIAN_POINT('Ctrl Pts',(15.,1.10295997362678,4.23058663740352));
#42007=CARTESIAN_POINT('Ctrl Pts',(14.6196795453431,-4.93380912478971,-0.000781869070653209));
#42008=CARTESIAN_POINT('Ctrl Pts',(14.6440164183552,-4.93522618578535,-0.759185507612087));
#42009=CARTESIAN_POINT('Ctrl Pts',(14.6683532913673,-4.77108836500343,-1.5170353890311));
#42010=CARTESIAN_POINT('Ctrl Pts',(14.6926901643794,-4.43811057180526,-2.19164729176556));
#42011=CARTESIAN_POINT('Ctrl Pts',(14.7457234551343,-3.71250756961112,-3.66171656346831));
#42012=CARTESIAN_POINT('Ctrl Pts',(14.7987567458892,-2.18514735941808,-4.7365201381057));
#42013=CARTESIAN_POINT('Ctrl Pts',(14.8517900366441,-0.555787191338123,
-4.91967375502775));
#42014=CARTESIAN_POINT('Ctrl Pts',(14.9011933577627,0.962048161810347,-5.09029105638777));
#42015=CARTESIAN_POINT('Ctrl Pts',(14.9505966788814,2.56839815963549,-4.48714255609281));
#42016=CARTESIAN_POINT('Ctrl Pts',(15.,3.61714728420828,-3.37770697643486));
#42017=CARTESIAN_POINT('',(2.442,-2.53835875722685,-3.55965150255047));
#42018=CARTESIAN_POINT('Ctrl Pts',(2.442,-2.54476592700513,-3.5626931430771));
#42019=CARTESIAN_POINT('Ctrl Pts',(2.442,-2.62978545394211,-3.51047303783495));
#42020=CARTESIAN_POINT('Ctrl Pts',(2.442,-2.71273826723953,-3.45525941651742));
#42021=CARTESIAN_POINT('Ctrl Pts',(2.442,-2.79343800990703,-3.3970840011207));
#42022=CARTESIAN_POINT('Ctrl Pts',(2.442,-2.89895370622653,-3.32101908119211));
#42023=CARTESIAN_POINT('Ctrl Pts',(2.442,-3.00061904678095,-3.23989255120093));
#42024=CARTESIAN_POINT('Ctrl Pts',(2.442,-3.09834171154448,-3.15412282181048));
#42025=CARTESIAN_POINT('Ctrl Pts',(2.442,-3.1628382401109,-3.09751517797319));
#42026=CARTESIAN_POINT('Ctrl Pts',(2.442,-3.2256168811051,-3.03888395058717));
#42027=CARTESIAN_POINT('Ctrl Pts',(2.442,-3.28664452788624,-2.97833910745001));
#42028=CARTESIAN_POINT('Ctrl Pts',(2.442,-3.32011196664812,-2.94513643723554));
#42029=CARTESIAN_POINT('Ctrl Pts',(2.442,-3.35305271398046,-2.91135813117016));
#42030=CARTESIAN_POINT('Ctrl Pts',(2.442,-3.3854605609159,-2.8770214217979));
#42031=CARTESIAN_POINT('Ctrl Pts',(2.442,-3.40589909658775,-2.85536641766396));
#42032=CARTESIAN_POINT('Ctrl Pts',(2.442,-3.42612869710155,-2.83348579784071));
#42033=CARTESIAN_POINT('Ctrl Pts',(2.442,-3.44612818959239,-2.81140576655678));
#42034=CARTESIAN_POINT('Ctrl Pts',(2.442,-3.53547878676924,-2.71276006433175));
#42035=CARTESIAN_POINT('Ctrl Pts',(2.442,-3.62031028150167,-2.61006461635602));
#42036=CARTESIAN_POINT('Ctrl Pts',(2.442,-3.70052458494235,-2.50375047198745));
#42037=CARTESIAN_POINT('Ctrl Pts',(2.442,-3.7820321149224,-2.39572231568946));
#42038=CARTESIAN_POINT('Ctrl Pts',(2.442,-3.85877282818418,-2.28395727639001));
#42039=CARTESIAN_POINT('Ctrl Pts',(2.442,-3.93061046973195,-2.16886637126524));
#42040=CARTESIAN_POINT('Ctrl Pts',(2.442,-3.9620394379091,-2.11851410027316));
#42041=CARTESIAN_POINT('Ctrl Pts',(2.442,-3.9925294608403,-2.06752476305505));
#42042=CARTESIAN_POINT('Ctrl Pts',(2.442,-4.02206682291391,-2.01593079161707));
#42043=CARTESIAN_POINT('Ctrl Pts',(2.442,-4.03680819585422,-1.99018150593124));
#42044=CARTESIAN_POINT('Ctrl Pts',(2.442,-4.05131226051438,-1.96428160335949));
#42045=CARTESIAN_POINT('Ctrl Pts',(2.442,-4.06557717039628,-1.93823502190503));
#42046=CARTESIAN_POINT('Ctrl Pts',(2.442,-4.07800796634773,-1.91553738539882));
#42047=CARTESIAN_POINT('Ctrl Pts',(2.442,-4.09025879764027,-1.89272505333989));
#42048=CARTESIAN_POINT('Ctrl Pts',(2.442,-4.10231620390219,-1.86982427382633));
#42049=CARTESIAN_POINT('Ctrl Pts',(2.442,-4.16671595836278,-1.74750903076393));
#42050=CARTESIAN_POINT('Ctrl Pts',(2.442,-4.22567136107007,-1.62254840773803));
#42051=CARTESIAN_POINT('Ctrl Pts',(2.442,-4.27907565912676,-1.49538917481992));
#42052=CARTESIAN_POINT('Ctrl Pts',(2.442,-4.33307972063718,-1.3668018646967));
#42053=CARTESIAN_POINT('Ctrl Pts',(2.442,-4.38140775201378,-1.23596560038919));
#42054=CARTESIAN_POINT('Ctrl Pts',(2.442,-4.4239099749577,-1.10330645426441));
#42055=CARTESIAN_POINT('Ctrl Pts',(2.442,-4.46640455952458,-0.970671149259102));
#42056=CARTESIAN_POINT('Ctrl Pts',(2.442,-4.50307583544893,-0.836212855602582));
#42057=CARTESIAN_POINT('Ctrl Pts',(2.442,-4.53372854767286,-0.700332695469703));
#42058=CARTESIAN_POINT('Ctrl Pts',(2.442,-4.55671808184081,-0.598422575370044));
#42059=CARTESIAN_POINT('Ctrl Pts',(2.442,-4.57632128194439,-0.495712076186221));
#42060=CARTESIAN_POINT('Ctrl Pts',(2.442,-4.59243682756127,-0.392365211825747));
#42061=CARTESIAN_POINT('Ctrl Pts',(2.442,-4.59910320879343,-0.349614589950796));
#42062=CARTESIAN_POINT('Ctrl Pts',(2.442,-4.60517259456302,-0.306755042017714));
#42063=CARTESIAN_POINT('Ctrl Pts',(2.442,-4.61063692900446,-0.263798081557451));
#42064=CARTESIAN_POINT('Ctrl Pts',(2.442,-4.61410845547613,-0.236507250994499));
#42065=CARTESIAN_POINT('Ctrl Pts',(2.442,-4.61733639162291,-0.209170445649368));
#42066=CARTESIAN_POINT('Ctrl Pts',(2.442,-4.62031493224596,-0.18182658773287));
#42067=CARTESIAN_POINT('Ctrl Pts',(2.442,-4.63566282271897,-0.0409285475431649));
#42068=CARTESIAN_POINT('Ctrl Pts',(2.442,-4.64441339445427,0.100293053460323));
#42069=CARTESIAN_POINT('Ctrl Pts',(2.442,-4.64641666149764,0.241410427951467));
#42070=CARTESIAN_POINT('Ctrl Pts',(2.442,-4.64785067414324,0.34242746419886));
#42071=CARTESIAN_POINT('Ctrl Pts',(2.442,-4.64582632158149,0.44339171925975));
#42072=CARTESIAN_POINT('Ctrl Pts',(2.442,-4.64027315559012,0.544151909983444));
#42073=CARTESIAN_POINT('Ctrl Pts',(2.442,-4.63271766788419,0.681243504839959));
#42074=CARTESIAN_POINT('Ctrl Pts',(2.442,-4.61863213421743,0.817957532855541));
#42075=CARTESIAN_POINT('Ctrl Pts',(2.442,-4.59828444891196,0.953915700962727));
#42076=CARTESIAN_POINT('Ctrl Pts',(2.442,-4.57764456106668,1.09182629370359));
#42077=CARTESIAN_POINT('Ctrl Pts',(2.442,-4.55056120109121,1.22895990852911));
#42078=CARTESIAN_POINT('Ctrl Pts',(2.442,-4.51726046982246,1.36491871255982));
#42079=CARTESIAN_POINT('Ctrl Pts',(2.442,-4.50842331151333,1.40099868524999));
#42080=CARTESIAN_POINT('Ctrl Pts',(2.442,-4.49914802401335,1.43699587249988));
#42081=CARTESIAN_POINT('Ctrl Pts',(2.442,-4.48943823757219,1.47290269877862));
#42082=CARTESIAN_POINT('Ctrl Pts',(2.442,-4.48092388288684,1.50438881398979));
#42083=CARTESIAN_POINT('Ctrl Pts',(2.442,-4.47207542720719,1.53580544774456));
#42084=CARTESIAN_POINT('Ctrl Pts',(2.442,-4.46289516701416,1.56714743748963));
#42085=CARTESIAN_POINT('Ctrl Pts',(2.442,-4.4581432952735,1.58337062857943));
#42086=CARTESIAN_POINT('Ctrl Pts',(2.442,-4.453303331417,1.59957094704679));
#42087=CARTESIAN_POINT('Ctrl Pts',(2.442,-4.44837819999916,1.61573970578171));
#42088=CARTESIAN_POINT('Ctrl Pts',(2.442,-4.40742424060596,1.75018783162665));
#42089=CARTESIAN_POINT('Ctrl Pts',(2.442,-4.36053854645612,1.8826158785883));
#42090=CARTESIAN_POINT('Ctrl Pts',(2.442,-4.30802922843631,2.01263872476853));
#42091=CARTESIAN_POINT('Ctrl Pts',(2.442,-4.25424635130186,2.1458151403934));
#42092=CARTESIAN_POINT('Ctrl Pts',(2.442,-4.19456362122613,2.2764690547453));
#42093=CARTESIAN_POINT('Ctrl Pts',(2.442,-4.12925671054388,2.40418379216483));
#42094=CARTESIAN_POINT('Ctrl Pts',(2.442,-4.06394979986163,2.53189852958436));
#42095=CARTESIAN_POINT('Ctrl Pts',(2.442,-3.99301835733987,2.65667490140106));
#42096=CARTESIAN_POINT('Ctrl Pts',(2.442,-3.91668729343188,2.77808134282536));
#42097=CARTESIAN_POINT('Ctrl Pts',(2.442,-3.86260196243339,2.86410539690767));
#42098=CARTESIAN_POINT('Ctrl Pts',(2.442,-3.80580461723952,2.94843722848745));
#42099=CARTESIAN_POINT('Ctrl Pts',(2.442,-3.74638249061058,3.03097790114148));
#42100=CARTESIAN_POINT('Ctrl Pts',(2.442,-3.71992510293393,3.06772869919243));
#42101=CARTESIAN_POINT('Ctrl Pts',(2.442,-3.69294722628387,3.10412431349132));
#42102=CARTESIAN_POINT('Ctrl Pts',(2.442,-3.66545589048721,3.14015549455613));
#42103=CARTESIAN_POINT('Ctrl Pts',(2.442,-3.65033714917244,3.15997068687031));
#42104=CARTESIAN_POINT('Ctrl Pts',(2.442,-3.63506311013638,3.17967565396125));
#42105=CARTESIAN_POINT('Ctrl Pts',(2.442,-3.61963489260881,3.19926881184803));
#42106=CARTESIAN_POINT('Ctrl Pts',(2.442,-3.60720401841877,3.21505547548825));
#42107=CARTESIAN_POINT('Ctrl Pts',(2.442,-3.59467227033619,3.23077043036965));
#42108=CARTESIAN_POINT('Ctrl Pts',(2.442,-3.58205135250517,3.24639931681853));
#42109=CARTESIAN_POINT('Ctrl Pts',(2.442,-3.49134773591549,3.35872050796831));
#42110=CARTESIAN_POINT('Ctrl Pts',(2.442,-3.39591563875028,3.46676085122522));
#42111=CARTESIAN_POINT('Ctrl Pts',(2.442,-3.29608057910503,3.57028822611568));
#42112=CARTESIAN_POINT('Ctrl Pts',(2.442,-3.19517230794316,3.67492850434302));
#42113=CARTESIAN_POINT('Ctrl Pts',(2.442,-3.0897655304088,3.77495887254834));
#42114=CARTESIAN_POINT('Ctrl Pts',(2.442,-2.98014938690035,3.87011544671376));
#42115=CARTESIAN_POINT('Ctrl Pts',(2.442,-2.87082805651637,3.96501609683327));
#42116=CARTESIAN_POINT('Ctrl Pts',(2.442,-2.75731950265513,4.0550696988635));
#42117=CARTESIAN_POINT('Ctrl Pts',(2.442,-2.63987053755491,4.13998182739019));
#42118=CARTESIAN_POINT('Ctrl Pts',(2.442,-2.52418958462514,4.22361573540189));
#42119=CARTESIAN_POINT('Ctrl Pts',(2.442,-2.40468545676967,4.30226226485196));
#42120=CARTESIAN_POINT('Ctrl Pts',(2.442,-2.28156245177909,4.37560083866042));
#42121=CARTESIAN_POINT('Ctrl Pts',(2.442,-2.24442645244809,4.39772100400316));
#42122=CARTESIAN_POINT('Ctrl Pts',(2.442,-2.20696104153711,4.41935798923143));
#42123=CARTESIAN_POINT('Ctrl Pts',(2.442,-2.16917135428609,4.440502182833));
#42124=CARTESIAN_POINT('Ctrl Pts',(2.442,-2.54476592700512,-3.56269314307711));
#42125=CARTESIAN_POINT('Ctrl Pts',(2.49140332111864,-1.44097312181521,-4.34097806869132));
#42126=CARTESIAN_POINT('Ctrl Pts',(2.59383993299217,1.66634742138771,-4.84186302574293));
#42127=CARTESIAN_POINT('Ctrl Pts',(2.74930983562058,4.99693901203929,-1.32514448694853));
#42128=CARTESIAN_POINT('Ctrl Pts',(2.90840970788525,3.81836490750785,3.48733811875686));
#42129=CARTESIAN_POINT('Ctrl Pts',(3.06750958014992,-0.870820132749773,
5.09763547084385));
#42130=CARTESIAN_POINT('Ctrl Pts',(3.19490297482318,-3.98390803658994,2.63581590170141));
#42131=CARTESIAN_POINT('Ctrl Pts',(3.26926307874154,-4.36855469401081,0.589937737338669));
#42132=CARTESIAN_POINT('Ctrl Pts',(3.29058989190502,-4.36585073597542,0.00220040158241119));
#42133=CARTESIAN_POINT('Origin',(2.442,-4.51336705371395E-16,0.));
#42134=CARTESIAN_POINT('',(2.442,-4.942,-6.05220448138622E-16));
#42135=CARTESIAN_POINT('Origin',(2.442,0.,0.));
#42136=CARTESIAN_POINT('Origin',(2.442,0.,0.));
#42137=CARTESIAN_POINT('',(2.442,2.53835875722685,-3.55965150255046));
#42138=CARTESIAN_POINT('Ctrl Pts',(2.442,2.17574915139363,4.44508346536535));
#42139=CARTESIAN_POINT('Ctrl Pts',(2.442,2.27393842303551,4.39078104776067));
#42140=CARTESIAN_POINT('Ctrl Pts',(2.442,2.36998244314937,4.3330049458102));
#42141=CARTESIAN_POINT('Ctrl Pts',(2.442,2.46367187398648,4.27174666136024));
#42142=CARTESIAN_POINT('Ctrl Pts',(2.442,2.5844170631878,4.19279812810554));
#42143=CARTESIAN_POINT('Ctrl Pts',(2.442,2.70125282028097,4.10806686721375));
#42144=CARTESIAN_POINT('Ctrl Pts',(2.442,2.81399829649834,4.0179742426192));
#42145=CARTESIAN_POINT('Ctrl Pts',(2.442,2.88459899475852,3.96155865577824));
#42146=CARTESIAN_POINT('Ctrl Pts',(2.442,2.95359512383052,3.90303992936404));
#42147=CARTESIAN_POINT('Ctrl Pts',(2.442,3.02093464599862,3.84251467551746));
#42148=CARTESIAN_POINT('Ctrl Pts',(2.442,3.05981425658111,3.80756939785292));
#42149=CARTESIAN_POINT('Ctrl Pts',(2.442,3.09814151990465,3.77195515070165));
#42150=CARTESIAN_POINT('Ctrl Pts',(2.442,3.13590544710532,3.73568989784483));
#42151=CARTESIAN_POINT('Ctrl Pts',(2.442,3.15300708404911,3.71926694520179));
#42152=CARTESIAN_POINT('Ctrl Pts',(2.442,3.16999457279843,3.70270910164703));
#42153=CARTESIAN_POINT('Ctrl Pts',(2.442,3.18686241961533,3.68602239183288));
#42154=CARTESIAN_POINT('Ctrl Pts',(2.442,3.28923141842677,3.58475269240563));
#42155=CARTESIAN_POINT('Ctrl Pts',(2.442,3.38701377017835,3.47892244063486));
#42156=CARTESIAN_POINT('Ctrl Pts',(2.442,3.48003362886399,3.36895094136753));
#42157=CARTESIAN_POINT('Ctrl Pts',(2.442,3.57217417702745,3.26001899535055));
#42158=CARTESIAN_POINT('Ctrl Pts',(2.442,3.65964211140465,3.14702295122995));
#42159=CARTESIAN_POINT('Ctrl Pts',(2.442,3.7422262628366,3.03034212452304));
#42160=CARTESIAN_POINT('Ctrl Pts',(2.442,3.78089446668873,2.97570890598769));
#42161=CARTESIAN_POINT('Ctrl Pts',(2.442,3.81849136080162,2.92026751227786));
#42162=CARTESIAN_POINT('Ctrl Pts',(2.442,3.85499193604736,2.86405544490254));
#42163=CARTESIAN_POINT('Ctrl Pts',(2.442,3.87362735212517,2.83535630092795));
#42164=CARTESIAN_POINT('Ctrl Pts',(2.442,3.89197696341109,2.80645625920063));
#42165=CARTESIAN_POINT('Ctrl Pts',(2.442,3.91003721456594,2.77736024690742));
#42166=CARTESIAN_POINT('Ctrl Pts',(2.442,3.92205565721194,2.75799790515617));
#42167=CARTESIAN_POINT('Ctrl Pts',(2.442,3.93394595584916,2.73854877858126));
#42168=CARTESIAN_POINT('Ctrl Pts',(2.442,3.94570702391603,2.71901431104455));
#42169=CARTESIAN_POINT('Ctrl Pts',(2.442,3.95577364652109,2.70229422139244));
#42170=CARTESIAN_POINT('Ctrl Pts',(2.442,3.96574336530622,2.68551524968513));
#42171=CARTESIAN_POINT('Ctrl Pts',(2.442,3.97561165866684,2.66868529315884));
#42172=CARTESIAN_POINT('Ctrl Pts',(2.442,4.0484785180189,2.54441394954467));
#42173=CARTESIAN_POINT('Ctrl Pts',(2.442,4.11588703074174,2.417252482731));
#42174=CARTESIAN_POINT('Ctrl Pts',(2.442,4.17765759536301,2.28760379752714));
#42175=CARTESIAN_POINT('Ctrl Pts',(2.442,4.23930632062562,2.1582108378902));
#42176=CARTESIAN_POINT('Ctrl Pts',(2.442,4.29533963180827,2.02633968480384));
#42177=CARTESIAN_POINT('Ctrl Pts',(2.442,4.34553172404092,1.89237006930549));
#42178=CARTESIAN_POINT('Ctrl Pts',(2.442,4.3954097927595,1.75923862586906));
#42179=CARTESIAN_POINT('Ctrl Pts',(2.442,4.43951977998791,1.62403415245028));
#42180=CARTESIAN_POINT('Ctrl Pts',(2.442,4.47758902444189,1.48712008745362));
#42181=CARTESIAN_POINT('Ctrl Pts',(2.442,4.50614095778236,1.38443453870612));
#42182=CARTESIAN_POINT('Ctrl Pts',(2.442,4.53129396154129,1.28078709139831));
#42183=CARTESIAN_POINT('Ctrl Pts',(2.442,4.55291251756889,1.17633139028504));
#42184=CARTESIAN_POINT('Ctrl Pts',(2.442,4.56133538043379,1.13563412795118));
#42185=CARTESIAN_POINT('Ctrl Pts',(2.442,4.56922152498248,1.09481419371376));
#42186=CARTESIAN_POINT('Ctrl Pts',(2.442,4.57656216912564,1.05388078213205));
#42187=CARTESIAN_POINT('Ctrl Pts',(2.442,4.57999850661446,1.03471883748249));
#42188=CARTESIAN_POINT('Ctrl Pts',(2.442,4.58331529642097,1.0155320264721));
#42189=CARTESIAN_POINT('Ctrl Pts',(2.442,4.58651160414136,0.996321299140574));
#42190=CARTESIAN_POINT('Ctrl Pts',(2.442,4.58947907947802,0.978485920152514));
#42191=CARTESIAN_POINT('Ctrl Pts',(2.442,4.59234189163767,0.96063463462557));
#42192=CARTESIAN_POINT('Ctrl Pts',(2.442,4.5950983362346,0.942776006748339));
#42193=CARTESIAN_POINT('Ctrl Pts',(2.442,4.61625709495595,0.80569130032306));
#42194=CARTESIAN_POINT('Ctrl Pts',(2.442,4.63117586815545,0.668035160277971));
#42195=CARTESIAN_POINT('Ctrl Pts',(2.442,4.63964588153731,0.530152019773935));
#42196=CARTESIAN_POINT('Ctrl Pts',(2.442,4.64589434249683,0.428433476771435));
#42197=CARTESIAN_POINT('Ctrl Pts',(2.442,4.64863225146208,0.326591103300644));
#42198=CARTESIAN_POINT('Ctrl Pts',(2.442,4.64775755650822,0.224762372538238));
#42199=CARTESIAN_POINT('Ctrl Pts',(2.442,4.64656482049337,0.0859084852581371));
#42200=CARTESIAN_POINT('Ctrl Pts',(2.442,4.63865657058669,-0.0529208546614462));
#42201=CARTESIAN_POINT('Ctrl Pts',(2.442,4.62423104198867,-0.191283307402043));
#42202=CARTESIAN_POINT('Ctrl Pts',(2.442,4.60977115054211,-0.329975351392945));
#42203=CARTESIAN_POINT('Ctrl Pts',(2.442,4.58876252367756,-0.46819910089437));
#42204=CARTESIAN_POINT('Ctrl Pts',(2.442,4.56135630357545,-0.605490145703256));
#42205=CARTESIAN_POINT('Ctrl Pts',(2.442,4.55350762775731,-0.644807968424675));
#42206=CARTESIAN_POINT('Ctrl Pts',(2.442,4.54513396735176,-0.684049133988946));
#42207=CARTESIAN_POINT('Ctrl Pts',(2.442,4.53623820728588,-0.723202303446103));
#42208=CARTESIAN_POINT('Ctrl Pts',(2.442,4.5313324340908,-0.744794226767168));
#42209=CARTESIAN_POINT('Ctrl Pts',(2.442,4.52626787353334,-0.766359384643764));
#42210=CARTESIAN_POINT('Ctrl Pts',(2.442,4.52104497323125,-0.787895845429721));
#42211=CARTESIAN_POINT('Ctrl Pts',(2.442,4.5172361488522,-0.8036014097973));
#42212=CARTESIAN_POINT('Ctrl Pts',(2.442,4.51334341520424,-0.819290338968791));
#42213=CARTESIAN_POINT('Ctrl Pts',(2.442,4.50936943923919,-0.834952609158587));
#42214=CARTESIAN_POINT('Ctrl Pts',(2.442,4.47555821798973,-0.968209701630727));
#42215=CARTESIAN_POINT('Ctrl Pts',(2.442,4.43582542541766,-1.09972449252871));
#42216=CARTESIAN_POINT('Ctrl Pts',(2.442,4.39039730266716,-1.22908266281593));
#42217=CARTESIAN_POINT('Ctrl Pts',(2.442,4.34489179137645,-1.3586611996813));
#42218=CARTESIAN_POINT('Ctrl Pts',(2.442,4.29367113064587,-1.48607655014092));
#42219=CARTESIAN_POINT('Ctrl Pts',(2.442,4.23691420217938,-1.61089379623584));
#42220=CARTESIAN_POINT('Ctrl Pts',(2.442,4.18155469671018,-1.73263789346833));
#42221=CARTESIAN_POINT('Ctrl Pts',(2.442,4.12092766181959,-1.85191084354222));
#42222=CARTESIAN_POINT('Ctrl Pts',(2.442,4.05516007761845,-1.96828148190162));
#42223=CARTESIAN_POINT('Ctrl Pts',(2.442,4.00954370013694,-2.04899612318953));
#42224=CARTESIAN_POINT('Ctrl Pts',(2.442,3.96145346076867,-2.12831387894083));
#42225=CARTESIAN_POINT('Ctrl Pts',(2.442,3.91094915975807,-2.20613095532952));
#42226=CARTESIAN_POINT('Ctrl Pts',(2.442,3.88614906048688,-2.24434297254026));
#42227=CARTESIAN_POINT('Ctrl Pts',(2.442,3.86076675497426,-2.282193003155));
#42228=CARTESIAN_POINT('Ctrl Pts',(2.442,3.83480875614052,-2.31966796647033));
#42229=CARTESIAN_POINT('Ctrl Pts',(2.442,3.81920063335576,-2.34220105280439));
#42230=CARTESIAN_POINT('Ctrl Pts',(2.442,3.80338436629605,-2.36459852612736));
#42231=CARTESIAN_POINT('Ctrl Pts',(2.442,3.7873613119109,-2.38685744513759));
#42232=CARTESIAN_POINT('Ctrl Pts',(2.442,3.7758201780042,-2.4028901664116));
#42233=CARTESIAN_POINT('Ctrl Pts',(2.442,3.76417601821905,-2.41884502890004));
#42234=CARTESIAN_POINT('Ctrl Pts',(2.442,3.75243436377876,-2.43471475864026));
#42235=CARTESIAN_POINT('Ctrl Pts',(2.442,3.66960454851416,-2.54666548835777));
#42236=CARTESIAN_POINT('Ctrl Pts',(2.442,3.58185449040889,-2.65448334060622));
#42237=CARTESIAN_POINT('Ctrl Pts',(2.442,3.48945737545467,-2.75787873450307));
#42238=CARTESIAN_POINT('Ctrl Pts',(2.442,3.4000952056859,-2.85787792546587));
#42239=CARTESIAN_POINT('Ctrl Pts',(2.442,3.30638549610641,-2.9537407482109));
#42240=CARTESIAN_POINT('Ctrl Pts',(2.442,3.2085383796773,-3.0451683648695));
#42241=CARTESIAN_POINT('Ctrl Pts',(2.442,3.11163722459243,-3.13571208229519));
#42242=CARTESIAN_POINT('Ctrl Pts',(2.442,3.01067774999476,-3.2219063667006));
#42243=CARTESIAN_POINT('Ctrl Pts',(2.442,2.90583625254343,-3.3034183821363));
#42244=CARTESIAN_POINT('Ctrl Pts',(2.442,2.80312546231272,-3.38327381841128));
#42245=CARTESIAN_POINT('Ctrl Pts',(2.442,2.69668833862294,-3.45863567293516));
#42246=CARTESIAN_POINT('Ctrl Pts',(2.442,2.58667139778511,-3.52914465758715));
#42247=CARTESIAN_POINT('Ctrl Pts',(2.442,2.57064305173904,-3.53941709742008));
#42248=CARTESIAN_POINT('Ctrl Pts',(2.442,2.55453869568167,-3.54958644617886));
#42249=CARTESIAN_POINT('Ctrl Pts',(2.442,2.53835875722688,-3.55965150255044));
#42250=CARTESIAN_POINT('Origin',(2.442,0.,0.));
#42251=CARTESIAN_POINT('Origin',(0.59341010809499,0.,0.));
#42252=CARTESIAN_POINT('Ctrl Pts',(2.442,2.53835875722685,-3.55965150255046));
#42253=CARTESIAN_POINT('Ctrl Pts',(2.46851664537744,3.13142872242371,-3.13673809691875));
#42254=CARTESIAN_POINT('Ctrl Pts',(2.52154993613233,4.09225274784706,-1.99049633126479));
#42255=CARTESIAN_POINT('Ctrl Pts',(2.62761651764211,4.7260019639421,0.960791047637318));
#42256=CARTESIAN_POINT('Ctrl Pts',(2.76019974452934,2.58737835299157,4.47689474139548));
#42257=CARTESIAN_POINT('Ctrl Pts',(2.919299616794,-2.37603566784794,4.59603588578678));
#42258=CARTESIAN_POINT('Ctrl Pts',(3.03036973798255,-4.31032048543761,1.72682559663222));
#42259=CARTESIAN_POINT('Ctrl Pts',(3.08840656841621,-4.37812303221146,0.139072831115389));
#42260=CARTESIAN_POINT('Ctrl Pts',(3.09341010809498,-4.3772103018885,0.00211459834950896));
#42261=CARTESIAN_POINT('Ctrl Pts',(2.11291034656191,2.86929757049747,-4.02374147429197));
#42262=CARTESIAN_POINT('Ctrl Pts',(2.13942699193936,3.53968910023281,-3.5456906850349));
#42263=CARTESIAN_POINT('Ctrl Pts',(2.19246028269425,4.62578066785455,-2.25000751809486));
#42264=CARTESIAN_POINT('Ctrl Pts',(2.29852686420402,5.34215501047619,1.08605429035303));
#42265=CARTESIAN_POINT('Ctrl Pts',(2.43111009109125,2.92470810166618,5.06057040530109));
#42266=CARTESIAN_POINT('Ctrl Pts',(2.59020996335591,-2.68581158977685,5.19524459001793));
#42267=CARTESIAN_POINT('Ctrl Pts',(2.74930983562059,-5.81776718514297,0.549476222463121));
#42268=CARTESIAN_POINT('Ctrl Pts',(2.90840970788525,-3.60982419207306,-4.59760538215123));
#42269=CARTESIAN_POINT('Ctrl Pts',(3.06750958014992,1.91775327909424,-5.52219013742084));
#42270=CARTESIAN_POINT('Ctrl Pts',(3.22660945241459,5.68177238095773,-1.37195370543713));
#42271=CARTESIAN_POINT('Ctrl Pts',(3.38570932467925,4.22608756769742,4.03835092191338));
#42272=CARTESIAN_POINT('Ctrl Pts',(3.54480919694392,-1.11299042776881,5.73842699095229));
#42273=CARTESIAN_POINT('Ctrl Pts',(3.70390906920859,-5.4292251435763,2.16582476905545));
#42274=CARTESIAN_POINT('Ctrl Pts',(3.86300894147326,-4.75712770456746,-3.39669458215663));
#42275=CARTESIAN_POINT('Ctrl Pts',(4.02210881373792,0.285939063906139,-5.83832346391982));
#42276=CARTESIAN_POINT('Ctrl Pts',(4.18120868600259,5.06625102656692,-2.91560479978825));
#42277=CARTESIAN_POINT('Ctrl Pts',(4.34030855826727,5.19164084677873,2.6859997205203));
#42278=CARTESIAN_POINT('Ctrl Pts',(4.49940843053192,0.54687470849627,5.81967771757739));
#42279=CARTESIAN_POINT('Ctrl Pts',(4.6585083027966,-4.60036279511536,3.60615672221117));
#42280=CARTESIAN_POINT('Ctrl Pts',(4.81760817506126,-5.52072884012978,-1.92074695394265));
#42281=CARTESIAN_POINT('Ctrl Pts',(4.97670804732594,-1.36857562124414,-5.68284387364681));
#42282=CARTESIAN_POINT('Ctrl Pts',(5.1358079195906,4.04104222632025,-4.2234688878305));
#42283=CARTESIAN_POINT('Ctrl Pts',(5.29490779185526,5.73769777151174,1.11648452511799));
#42284=CARTESIAN_POINT('Ctrl Pts',(5.45400766411994,2.16248115397357,5.4305974129897));
#42285=CARTESIAN_POINT('Ctrl Pts',(5.61310753638461,-3.39965143533879,4.75500608748046));
#42286=CARTESIAN_POINT('Ctrl Pts',(5.77220740864926,-5.83813972404732,-0.289547192923355));
#42287=CARTESIAN_POINT('Ctrl Pts',(5.93130728091394,-2.91246860837872,-5.0680607283612));
#42288=CARTESIAN_POINT('Ctrl Pts',(6.0904071531786,2.68921686697644,-5.1899735605652));
#42289=CARTESIAN_POINT('Ctrl Pts',(6.24950702544328,5.82001460606655,-0.543270591629312));
#42290=CARTESIAN_POINT('Ctrl Pts',(6.40860689770793,3.60330655718976,4.60259652730006));
#42291=CARTESIAN_POINT('Ctrl Pts',(6.56770676997262,-1.92416683377643,5.51953756503503));
#42292=CARTESIAN_POINT('Ctrl Pts',(6.72680664223726,-5.68369049173104,1.3650550665912));
#42293=CARTESIAN_POINT('Ctrl Pts',(6.88590651450195,-4.22096474954825,-4.04365793826525));
#42294=CARTESIAN_POINT('Ctrl Pts',(7.04500638676661,1.12003878766801,-5.73700497233726));
#42295=CARTESIAN_POINT('Ctrl Pts',(7.20410625903129,5.43193599084382,-2.15911656250658));
#42296=CARTESIAN_POINT('Ctrl Pts',(7.36320613129594,4.75289913298194,3.4025964748266));
#42297=CARTESIAN_POINT('Ctrl Pts',(7.52230600356062,-0.293163811150279,
5.83795922550374));
#42298=CARTESIAN_POINT('Ctrl Pts',(7.68140587582529,-5.06986399900541,2.90932843977449));
#42299=CARTESIAN_POINT('Ctrl Pts',(7.84050574808994,-5.18830662273838,-2.69243148980496));
#42300=CARTESIAN_POINT('Ctrl Pts',(7.99960562035463,-0.539665045588934,
-5.82035003908004));
#42301=CARTESIAN_POINT('Ctrl Pts',(8.15870549261927,4.6048278564103,-3.6004546034754));
#42302=CARTESIAN_POINT('Ctrl Pts',(8.31780536488397,5.51834450386409,1.92758576346817));
#42303=CARTESIAN_POINT('Ctrl Pts',(8.47690523714861,1.3615338148167,5.68453503903047));
#42304=CARTESIAN_POINT('Ctrl Pts',(8.6360051094133,-4.04627200800777,4.21845893378935));
#42305=CARTESIAN_POINT('Ctrl Pts',(8.79510498167795,-5.73631001862683,-1.12359259033407));
#42306=CARTESIAN_POINT('Ctrl Pts',(8.95420485394264,-2.15575111784886,-5.43327249976962));
#42307=CARTESIAN_POINT('Ctrl Pts',(9.11330472620728,3.40554019567974,-4.75079034629598));
#42308=CARTESIAN_POINT('Ctrl Pts',(9.27240459847197,5.83777649322883,0.29678031260383));
#42309=CARTESIAN_POINT('Ctrl Pts',(9.43150447073662,2.90618715117436,5.07166532622579));
#42310=CARTESIAN_POINT('Ctrl Pts',(9.5906043430013,-2.69564507754667,5.18663769263969));
#42311=CARTESIAN_POINT('Ctrl Pts',(9.74970421526597,-5.82068323937394,0.536059293058277));
#42312=CARTESIAN_POINT('Ctrl Pts',(9.90880408753062,-3.59760126753682,-4.60705741867106));
#42313=CARTESIAN_POINT('Ctrl Pts',(10.0679039597953,1.93100395317568,-5.51714932472587));
#42314=CARTESIAN_POINT('Ctrl Pts',(10.22700383206,5.68537740488418,-1.35801204068925));
#42315=CARTESIAN_POINT('Ctrl Pts',(10.3861037043246,4.21595149912367,4.04888452510772));
#42316=CARTESIAN_POINT('Ctrl Pts',(10.5452035765893,-1.12714596190438,5.7356128632083));
#42317=CARTESIAN_POINT('Ctrl Pts',(10.704303448854,-5.43460692333051,2.15238484641792));
#42318=CARTESIAN_POINT('Ctrl Pts',(10.8634033211186,-4.74867973691283,-3.40848261060413));
#42319=CARTESIAN_POINT('Ctrl Pts',(11.0225031933833,0.300396701142615,-5.83759151867781));
#42320=CARTESIAN_POINT('Ctrl Pts',(11.181603065648,5.07346470521744,-2.90304475095743));
#42321=CARTESIAN_POINT('Ctrl Pts',(11.3407029379127,5.18496677569499,2.6988576378476));
#42322=CARTESIAN_POINT('Ctrl Pts',(11.4998028101773,0.532453327864645,5.82101419233996));
#42323=CARTESIAN_POINT('Ctrl Pts',(11.658902682442,-4.60928519958409,3.59474657690306));
#42324=CARTESIAN_POINT('Ctrl Pts',(11.8180025547066,-5.51595205379273,-1.93442145157114));
#42325=CARTESIAN_POINT('Ctrl Pts',(11.9771024269713,-1.35448969649516,-5.68621749350692));
#42326=CARTESIAN_POINT('Ctrl Pts',(12.136202299236,4.0514953946209,-4.21344262933229));
#42327=CARTESIAN_POINT('Ctrl Pts',(12.2953021715007,5.73491368637922,1.13069925139314));
#42328=CARTESIAN_POINT('Ctrl Pts',(12.4544020437653,2.14901740440843,5.435938589368));
#42329=CARTESIAN_POINT('Ctrl Pts',(12.61350191603,-3.41142305691351,4.74656859320694));
#42330=CARTESIAN_POINT('Ctrl Pts',(12.7726017882947,-5.83740557016221,-0.304015443712614));
#42331=CARTESIAN_POINT('Ctrl Pts',(12.9317016605593,-2.89989880903194,-5.0752574033357));
#42332=CARTESIAN_POINT('Ctrl Pts',(13.090801532824,2.70206450851665,-5.18330294401542));
#42333=CARTESIAN_POINT('Ctrl Pts',(13.2499014050887,5.82135183321988,-0.528829760776661));
#42334=CARTESIAN_POINT('Ctrl Pts',(13.4090012773533,3.5918734029674,4.61147785931481));
#42335=CARTESIAN_POINT('Ctrl Pts',(13.568101149618,-1.93780541854324,5.51481660462604));
#42336=CARTESIAN_POINT('Ctrl Pts',(13.7272010218827,-5.68711825886611,1.35084425750601));
#42337=CARTESIAN_POINT('Ctrl Pts',(13.8863008941473,-4.21081163680671,-4.05386972141555));
#42338=CARTESIAN_POINT('Ctrl Pts',(14.045400766412,1.13402108049327,-5.73466282725512));
#42339=CARTESIAN_POINT('Ctrl Pts',(14.2045006386766,5.43771114302852,-2.14478518100188));
#42340=CARTESIAN_POINT('Ctrl Pts',(14.3636005109413,4.74360568499834,3.41270336314633));
#42341=CARTESIAN_POINT('Ctrl Pts',(14.522700383206,-0.305998010418999,5.84042082931615));
#42342=CARTESIAN_POINT('Ctrl Pts',(14.6818002554707,-5.08024498950095,2.89039809604342));
#42343=CARTESIAN_POINT('Ctrl Pts',(14.8143834823579,-5.15920127145973,-1.76090213189674));
#42344=CARTESIAN_POINT('Ctrl Pts',(14.9204500638677,-2.85592546693168,-4.27832564748306));
#42345=CARTESIAN_POINT('Ctrl Pts',(14.9734833546226,-1.26412269067526,-4.84802178039354));
#42346=CARTESIAN_POINT('Ctrl Pts',(15.,-0.444071852043585,-4.9220081460947));
#42347=CARTESIAN_POINT('Ctrl Pts',(2.22260689770794,2.7589846327406,-3.8690448170448));
#42348=CARTESIAN_POINT('Ctrl Pts',(2.24912354308539,3.40360230762978,-3.40937315566285));
#42349=CARTESIAN_POINT('Ctrl Pts',(2.30215683384028,4.44793802785205,-2.16350378915151));
#42350=CARTESIAN_POINT('Ctrl Pts',(2.40822341535005,5.13677066163149,1.04429987611446));
#42351=CARTESIAN_POINT('Ctrl Pts',(2.54080664223728,2.81226485210798,4.86601185066588));
#42352=CARTESIAN_POINT('Ctrl Pts',(2.69990651450194,-2.58255294913388,4.99550835527422));
#42353=CARTESIAN_POINT('Ctrl Pts',(2.85900638676662,-5.59409746333456,0.528351074290705));
#42354=CARTESIAN_POINT('Ctrl Pts',(3.01810625903128,-3.47104098760242,-4.42084596843032));
#42355=CARTESIAN_POINT('Ctrl Pts',(3.17720613129595,1.84402338774907,-5.30988416289433));
#42356=CARTESIAN_POINT('Ctrl Pts',(3.33630600356061,5.46333111175862,-1.31920760992254));
#42357=CARTESIAN_POINT('Ctrl Pts',(3.49540587582529,4.06361151794782,3.88309259023319));
#42358=CARTESIAN_POINT('Ctrl Pts',(3.65450574808995,-1.07020042751062,5.51780758013057));
#42359=CARTESIAN_POINT('Ctrl Pts',(3.81360562035462,-5.22049329872007,2.08255752783316));
#42360=CARTESIAN_POINT('Ctrl Pts',(3.97270549261928,-4.57423529989974,-3.2661053529762));
#42361=CARTESIAN_POINT('Ctrl Pts',(4.13180536488396,0.274945858292602,-5.6138634359666));
#42362=CARTESIAN_POINT('Ctrl Pts',(4.29090523714862,4.87147407491826,-2.8035115355309));
#42363=CARTESIAN_POINT('Ctrl Pts',(4.45000510941329,4.99204316145134,2.5827338470078));
#42364=CARTESIAN_POINT('Ctrl Pts',(4.60910498167796,0.525849578060337,5.59593454349003));
#42365=CARTESIAN_POINT('Ctrl Pts',(4.76820485394263,-4.42349736996929,3.46751451718887));
#42366=CARTESIAN_POINT('Ctrl Pts',(4.92730472620729,-5.30847904659991,-1.84690196785421));
#42367=CARTESIAN_POINT('Ctrl Pts',(5.08640459847196,-1.3159593994642,-5.46436140986841));
#42368=CARTESIAN_POINT('Ctrl Pts',(5.24550447073663,3.88568042482271,-4.06109351577712));
#42369=CARTESIAN_POINT('Ctrl Pts',(5.40460434300129,5.51710639624116,1.07356019088643));
#42370=CARTESIAN_POINT('Ctrl Pts',(5.56370421526597,2.0793424612874,5.22181280990026));
#42371=CARTESIAN_POINT('Ctrl Pts',(5.72280408753062,-3.26894852705989,4.57219525044661));
#42372=CARTESIAN_POINT('Ctrl Pts',(5.8819039597953,-5.61368676015234,-0.278415269277996));
#42373=CARTESIAN_POINT('Ctrl Pts',(6.04100383205997,-2.80049591805253,-4.87321420096569));
#42374=CARTESIAN_POINT('Ctrl Pts',(6.20010370432464,2.58582730713721,-4.99043997567904));
#42375=CARTESIAN_POINT('Ctrl Pts',(6.35920357658931,5.59625847997334,-0.522384024974179));
#42376=CARTESIAN_POINT('Ctrl Pts',(6.51830344885396,3.46477392953576,4.42564522414607));
#42377=CARTESIAN_POINT('Ctrl Pts',(6.67740332111864,-1.85019036707925,5.30733357123562));
#42378=CARTESIAN_POINT('Ctrl Pts',(6.83650319338331,-5.46517547889638,1.31257419596142));
#42379=CARTESIAN_POINT('Ctrl Pts',(6.99560306564797,-4.05868565152838,-3.88819557317615));
#42380=CARTESIAN_POINT('Ctrl Pts',(7.15470293791265,1.07697780635339,-5.51644023240523));
#42381=CARTESIAN_POINT('Ctrl Pts',(7.3138028101773,5.22309992482595,-2.07610722481408));
#42382=CARTESIAN_POINT('Ctrl Pts',(7.47290268244198,4.57016929986445,3.27178034163821));
#42383=CARTESIAN_POINT('Ctrl Pts',(7.63200255470663,-0.281892843097165,
5.61351320105094));
#42384=CARTESIAN_POINT('Ctrl Pts',(7.79110242697132,-4.87494814311488,2.79747647628658));
#42385=CARTESIAN_POINT('Ctrl Pts',(7.95020229923598,-4.98883712489937,-2.58891834066233));
#42386=CARTESIAN_POINT('Ctrl Pts',(8.10930217150065,-0.518917097660577,
-5.59658101693815));
#42387=CARTESIAN_POINT('Ctrl Pts',(8.26840204376531,4.42779076763695,-3.46203162195772));
#42388=CARTESIAN_POINT('Ctrl Pts',(8.42750191602998,5.30618637846259,1.85347785269139));
#42389=CARTESIAN_POINT('Ctrl Pts',(8.58660178829465,1.30918832213859,5.4659875567529));
#42390=CARTESIAN_POINT('Ctrl Pts',(8.74570166055931,-3.89070914246317,4.05627617429522));
#42391=CARTESIAN_POINT('Ctrl Pts',(8.90480153282399,-5.51577199686659,-1.08039497961707));
#42392=CARTESIAN_POINT('Ctrl Pts',(9.06390140508865,-2.07287116795179,-5.22438505036529));
#42393=CARTESIAN_POINT('Ctrl Pts',(9.22300127735332,3.27461088827806,-4.5681415875351));
#42394=CARTESIAN_POINT('Ctrl Pts',(9.38210114961799,5.6133374940962,0.285370304632429));
#42395=CARTESIAN_POINT('Ctrl Pts',(9.54120102188265,2.79445595758408,4.87668021655706));
#42396=CARTESIAN_POINT('Ctrl Pts',(9.70030089414733,-2.59200837889555,4.98723235844268));
#42397=CARTESIAN_POINT('Ctrl Pts',(9.85940076641198,-5.59690140702245,0.515449971795401));
#42398=CARTESIAN_POINT('Ctrl Pts',(10.0185006386767,-3.45928798529643,-4.42993461220659));
#42399=CARTESIAN_POINT('Ctrl Pts',(10.1776005109413,1.8567646267687,-5.30503714914959));
#42400=CARTESIAN_POINT('Ctrl Pts',(10.336700383206,5.46679753703149,-1.30580194604518));
#42401=CARTESIAN_POINT('Ctrl Pts',(10.4958002554707,4.05386514039572,3.89322121880048));
#42402=CARTESIAN_POINT('Ctrl Pts',(10.6549001277353,-1.0838117383589,5.51510164426666));
#42403=CARTESIAN_POINT('Ctrl Pts',(10.814,-5.2256681707136,2.06963431610236));
#42404=CARTESIAN_POINT('Ctrl Pts',(10.9730998722647,-4.56611212258392,-3.27744017919686));
#42405=CARTESIAN_POINT('Ctrl Pts',(11.1321997445293,0.288847657594046,-5.61315963107182));
#42406=CARTESIAN_POINT('Ctrl Pts',(11.291299616794,4.87841041667205,-2.79143437000195));
#42407=CARTESIAN_POINT('Ctrl Pts',(11.4503994890586,4.98562568152621,2.59509742918897));
#42408=CARTESIAN_POINT('Ctrl Pts',(11.6094993613234,0.511982641443287,5.59721963617958));
#42409=CARTESIAN_POINT('Ctrl Pts',(11.768599233588,-4.43207674391413,3.45654304602252));
#42410=CARTESIAN_POINT('Ctrl Pts',(11.9276991058527,-5.30388590846277,-1.86005073611213));
#42411=CARTESIAN_POINT('Ctrl Pts',(12.0867989781173,-1.3024150218019,-5.46760532762948));
#42412=CARTESIAN_POINT('Ctrl Pts',(12.245898850382,3.89573171089409,-4.05145272654532));
#42413=CARTESIAN_POINT('Ctrl Pts',(12.4049987226467,5.51442934797128,1.08722841817489));
#42414=CARTESIAN_POINT('Ctrl Pts',(12.5640985949113,2.06639633867842,5.22694863955418));
#42415=CARTESIAN_POINT('Ctrl Pts',(12.723198467176,-3.28026757718596,4.56408214385256));
#42416=CARTESIAN_POINT('Ctrl Pts',(12.8822983394407,-5.61298083152789,-0.292327274083852));
#42417=CARTESIAN_POINT('Ctrl Pts',(13.0413982117053,-2.7884093768757,-4.88013419276635));
#42418=CARTESIAN_POINT('Ctrl Pts',(13.20049808397,2.59818100859393,-4.98402581747495));
#42419=CARTESIAN_POINT('Ctrl Pts',(13.3595979562347,5.59754429612724,-0.508498385918783));
#42420=CARTESIAN_POINT('Ctrl Pts',(13.5186978284993,3.45378033405525,4.43418510470741));
#42421=CARTESIAN_POINT('Ctrl Pts',(13.677797700764,-1.8633046031804,5.30279411274442));
#42422=CARTESIAN_POINT('Ctrl Pts',(13.8368975730287,-5.46847146218773,1.29890973526275));
#42423=CARTESIAN_POINT('Ctrl Pts',(13.9959974452934,-4.04892288508812,-3.89801475438421));
#42424=CARTESIAN_POINT('Ctrl Pts',(14.155097317558,1.09042253632216,-5.51418813337035));
#42425=CARTESIAN_POINT('Ctrl Pts',(14.3141971898227,5.22865304566401,-2.06232682721993));
#42426=CARTESIAN_POINT('Ctrl Pts',(14.4732970620873,4.56123314753381,3.28149866079956));
#42427=CARTESIAN_POINT('Ctrl Pts',(14.632396934352,-0.294233619083599,5.61588016610892));
#42428=CARTESIAN_POINT('Ctrl Pts',(14.7914968066167,-4.8849300263271,2.77927392804497));
#42429=CARTESIAN_POINT('Ctrl Pts',(14.9240800335039,-4.9608507571786,-1.69320253556725));
#42430=CARTESIAN_POINT('Ctrl Pts',(15.0301466150137,-2.74612663271131,-4.1138412539133));
#42431=CARTESIAN_POINT('Ctrl Pts',(15.0831799057686,-1.21552226347405,-4.66163486451439));
#42432=CARTESIAN_POINT('Ctrl Pts',(15.109696551146,-0.426999077480991,-4.73277675237597));
#42433=CARTESIAN_POINT('Ctrl Pts',(2.33230344885397,2.64867169498373,-3.71434815979763));
#42434=CARTESIAN_POINT('Ctrl Pts',(2.35882009423141,3.26751551502674,-3.2730556262908));
#42435=CARTESIAN_POINT('Ctrl Pts',(2.41185338498631,4.27009538784955,-2.07700006020815));
#42436=CARTESIAN_POINT('Ctrl Pts',(2.51791996649608,4.9313863127868,1.00254546187589));
#42437=CARTESIAN_POINT('Ctrl Pts',(2.65050319338331,2.69982160254977,4.67145329603068));
#42438=CARTESIAN_POINT('Ctrl Pts',(2.80960306564797,-2.47929430849091,4.7957721205305));
#42439=CARTESIAN_POINT('Ctrl Pts',(2.96870293791264,-5.37042774152615,0.507225926118294));
#42440=CARTESIAN_POINT('Ctrl Pts',(3.12780281017731,-3.33225778313177,-4.24408655470942));
#42441=CARTESIAN_POINT('Ctrl Pts',(3.28690268244198,1.7702934964039,-5.09757818836783));
#42442=CARTESIAN_POINT('Ctrl Pts',(3.44600255470665,5.24488984255953,-1.26646151440794));
#42443=CARTESIAN_POINT('Ctrl Pts',(3.60510242697131,3.90113546819821,3.727834258553));
#42444=CARTESIAN_POINT('Ctrl Pts',(3.76420229923598,-1.02741042725242,5.29718816930885));
#42445=CARTESIAN_POINT('Ctrl Pts',(3.92330217150065,-5.01176145386385,1.99929028661086));
#42446=CARTESIAN_POINT('Ctrl Pts',(4.08240204376532,-4.39134289523202,-3.13551612379576));
#42447=CARTESIAN_POINT('Ctrl Pts',(4.24150191602998,0.263952652679065,-5.38940340801339));
#42448=CARTESIAN_POINT('Ctrl Pts',(4.40060178829465,4.6766971232696,-2.69141827127356));
#42449=CARTESIAN_POINT('Ctrl Pts',(4.55970166055932,4.79244547612395,2.4794679734953));
#42450=CARTESIAN_POINT('Ctrl Pts',(4.71880153282398,0.504824447624409,5.37219136940268));
#42451=CARTESIAN_POINT('Ctrl Pts',(4.87790140508866,-4.24663194482322,3.32887231216658));
#42452=CARTESIAN_POINT('Ctrl Pts',(5.03700127735332,-5.09622925307003,-1.77305698176578));
#42453=CARTESIAN_POINT('Ctrl Pts',(5.196101149618,-1.26334317768426,-5.24587894609));
#42454=CARTESIAN_POINT('Ctrl Pts',(5.35520102188265,3.73031862332518,-3.89871814372373));
#42455=CARTESIAN_POINT('Ctrl Pts',(5.51430089414733,5.29651502097057,1.03063585665488));
#42456=CARTESIAN_POINT('Ctrl Pts',(5.67340076641199,1.99620376860123,5.01302820681081));
#42457=CARTESIAN_POINT('Ctrl Pts',(5.83250063867667,-3.13824561878099,4.38938441341275));
#42458=CARTESIAN_POINT('Ctrl Pts',(5.99160051094132,-5.38923379625736,-0.267283345632638));
#42459=CARTESIAN_POINT('Ctrl Pts',(6.15070038320601,-2.68852322772634,-4.67836767357019));
#42460=CARTESIAN_POINT('Ctrl Pts',(6.30980025547066,2.48243774729798,-4.79090639079288));
#42461=CARTESIAN_POINT('Ctrl Pts',(6.46890012773534,5.37250235388013,-0.501497458319054));
#42462=CARTESIAN_POINT('Ctrl Pts',(6.62799999999999,3.32624130188175,4.24869392099209));
#42463=CARTESIAN_POINT('Ctrl Pts',(6.78709987226468,-1.77621390038207,5.09512957743621));
#42464=CARTESIAN_POINT('Ctrl Pts',(6.94619974452933,-5.24666046606172,1.26009332533163));
#42465=CARTESIAN_POINT('Ctrl Pts',(7.10529961679401,-3.89640655350851,-3.73273320808705));
#42466=CARTESIAN_POINT('Ctrl Pts',(7.26439948905867,1.03391682503877,-5.2958754924732));
#42467=CARTESIAN_POINT('Ctrl Pts',(7.42349936132334,5.01426385880808,-1.99309788712159));
#42468=CARTESIAN_POINT('Ctrl Pts',(7.582599233588,4.38743946674697,3.14096420844982));
#42469=CARTESIAN_POINT('Ctrl Pts',(7.74169910585268,-0.270621875044055,
5.38906717659815));
#42470=CARTESIAN_POINT('Ctrl Pts',(7.90079897811734,-4.68003228722435,2.68562451279868));
#42471=CARTESIAN_POINT('Ctrl Pts',(8.05989885038201,-4.78936762706038,-2.4854051915197));
#42472=CARTESIAN_POINT('Ctrl Pts',(8.21899872264668,-0.498169149732212,
-5.37281199479628));
#42473=CARTESIAN_POINT('Ctrl Pts',(8.37809859491134,4.25075367886359,-3.32360864044003));
#42474=CARTESIAN_POINT('Ctrl Pts',(8.53719846717601,5.0940282530611,1.77936994191459));
#42475=CARTESIAN_POINT('Ctrl Pts',(8.69629833944068,1.25684282946048,5.24744007447532));
#42476=CARTESIAN_POINT('Ctrl Pts',(8.85539821170534,-3.73514627691857,3.89409341480108));
#42477=CARTESIAN_POINT('Ctrl Pts',(9.01449808397002,-5.29523397510635,-1.03719736890007));
#42478=CARTESIAN_POINT('Ctrl Pts',(9.17359795623469,-1.98999121805471,-5.01549760096096));
#42479=CARTESIAN_POINT('Ctrl Pts',(9.33269782849935,3.14368158087639,-4.38549282877422));
#42480=CARTESIAN_POINT('Ctrl Pts',(9.49179770076402,5.38889849496356,0.273960296661032));
#42481=CARTESIAN_POINT('Ctrl Pts',(9.65089757302868,2.68272476399379,4.68169510688832));
#42482=CARTESIAN_POINT('Ctrl Pts',(9.80999744529335,-2.48837168024444,4.78782702424569));
#42483=CARTESIAN_POINT('Ctrl Pts',(9.96909731755802,-5.37311957467096,0.494840650532518));
#42484=CARTESIAN_POINT('Ctrl Pts',(10.1281971898227,-3.32097470305603,-4.2528118057421));
#42485=CARTESIAN_POINT('Ctrl Pts',(10.2872970620874,1.78252530036171,-5.09292497357333));
#42486=CARTESIAN_POINT('Ctrl Pts',(10.446396934352,5.24821766917881,-1.2535918514011));
#42487=CARTESIAN_POINT('Ctrl Pts',(10.6054968066167,3.89177878166777,3.73755791249323));
#42488=CARTESIAN_POINT('Ctrl Pts',(10.7645966788814,-1.04047751481342,5.29459042532502));
#42489=CARTESIAN_POINT('Ctrl Pts',(10.923696551146,-5.01672941809669,1.98688378578681));
#42490=CARTESIAN_POINT('Ctrl Pts',(11.0827964234107,-4.383544508255,-3.14639774778959));
#42491=CARTESIAN_POINT('Ctrl Pts',(11.2418962956754,0.277298614045473,-5.38872774346583));
#42492=CARTESIAN_POINT('Ctrl Pts',(11.40099616794,4.68335612812668,-2.67982398904647));
#42493=CARTESIAN_POINT('Ctrl Pts',(11.5600960402047,4.78628458735744,2.49133722053032));
#42494=CARTESIAN_POINT('Ctrl Pts',(11.7191959124694,0.491511955021929,5.37342508001921));
#42495=CARTESIAN_POINT('Ctrl Pts',(11.878295784734,-4.25486828824417,3.31833951514198));
#42496=CARTESIAN_POINT('Ctrl Pts',(12.0373956569987,-5.09181976313282,-1.78568002065311));
#42497=CARTESIAN_POINT('Ctrl Pts',(12.1964955292634,-1.25034034710862,-5.24899316175204));
#42498=CARTESIAN_POINT('Ctrl Pts',(12.355595401528,3.73996802716727,-3.88946282375836));
#42499=CARTESIAN_POINT('Ctrl Pts',(12.5146952737927,5.29394500956333,1.04375758495663));
#42500=CARTESIAN_POINT('Ctrl Pts',(12.6737951460574,1.98377527294843,5.01795868974035));
#42501=CARTESIAN_POINT('Ctrl Pts',(12.832895018322,-3.14911209745843,4.38159569449818));
#42502=CARTESIAN_POINT('Ctrl Pts',(12.9919948905867,-5.38855609289356,-0.280639104455098));
#42503=CARTESIAN_POINT('Ctrl Pts',(13.1510947628514,-2.67691994471947,-4.68501098219699));
#42504=CARTESIAN_POINT('Ctrl Pts',(13.310194635116,2.4942975086712,-4.7847486909345));
#42505=CARTESIAN_POINT('Ctrl Pts',(13.4692945073807,5.37373675903462,-0.488167011060903));
#42506=CARTESIAN_POINT('Ctrl Pts',(13.6283943796454,3.31568726514309,4.25689235010001));
#42507=CARTESIAN_POINT('Ctrl Pts',(13.78749425191,-1.78880378781756,5.0907716208628));
#42508=CARTESIAN_POINT('Ctrl Pts',(13.9465941241747,-5.24982466550936,1.24697521301949));
#42509=CARTESIAN_POINT('Ctrl Pts',(14.1056939964394,-3.88703413336951,-3.74215978735286));
#42510=CARTESIAN_POINT('Ctrl Pts',(14.2647938687041,1.04682399215104,-5.2937134394856));
#42511=CARTESIAN_POINT('Ctrl Pts',(14.4238937409687,5.01959494829951,-1.97986847343797));
#42512=CARTESIAN_POINT('Ctrl Pts',(14.5829936132334,4.37886061006927,3.15029395845279));
#42513=CARTESIAN_POINT('Ctrl Pts',(14.742093485498,-0.282469227748196,5.39133950290171));
#42514=CARTESIAN_POINT('Ctrl Pts',(14.9011933577627,-4.68961506315326,2.66814976004653));
#42515=CARTESIAN_POINT('Ctrl Pts',(15.0337765846499,-4.76250024289745,-1.62550293923777));
#42516=CARTESIAN_POINT('Ctrl Pts',(15.1398431661597,-2.63632779849094,-3.94935686034355));
#42517=CARTESIAN_POINT('Ctrl Pts',(15.1928764569146,-1.16692183627285,-4.47524794863524));
#42518=CARTESIAN_POINT('Ctrl Pts',(15.2193931022921,-0.409926302918398,
-4.54354535865723));
#42519=CARTESIAN_POINT('Ctrl Pts',(2.442,2.53835875722685,-3.55965150255046));
#42520=CARTESIAN_POINT('Ctrl Pts',(2.46851664537744,3.13142872242371,-3.13673809691875));
#42521=CARTESIAN_POINT('Ctrl Pts',(2.52154993613233,4.09225274784706,-1.99049633126479));
#42522=CARTESIAN_POINT('Ctrl Pts',(2.62761651764211,4.7260019639421,0.960791047637318));
#42523=CARTESIAN_POINT('Ctrl Pts',(2.76019974452934,2.58737835299157,4.47689474139548));
#42524=CARTESIAN_POINT('Ctrl Pts',(2.919299616794,-2.37603566784794,4.59603588578678));
#42525=CARTESIAN_POINT('Ctrl Pts',(3.07839948905867,-5.14675801971775,0.48610077794589));
#42526=CARTESIAN_POINT('Ctrl Pts',(3.23749936132335,-3.19347457866112,-4.06732714098853));
#42527=CARTESIAN_POINT('Ctrl Pts',(3.396599233588,1.69656360505873,-4.88527221384132));
#42528=CARTESIAN_POINT('Ctrl Pts',(3.55569910585268,5.02644857336042,-1.21371541889335));
#42529=CARTESIAN_POINT('Ctrl Pts',(3.71479897811734,3.73865941844861,3.57257592687282));
#42530=CARTESIAN_POINT('Ctrl Pts',(3.87389885038201,-0.984620426994229,
5.07656875848712));
#42531=CARTESIAN_POINT('Ctrl Pts',(4.03299872264668,-4.80302960900762,1.91602304538856));
#42532=CARTESIAN_POINT('Ctrl Pts',(4.19209859491134,-4.2084504905643,-3.00492689461532));
#42533=CARTESIAN_POINT('Ctrl Pts',(4.35119846717601,0.252959447065525,-5.16494338006019));
#42534=CARTESIAN_POINT('Ctrl Pts',(4.51029833944068,4.48192017162094,-2.5793250070162));
#42535=CARTESIAN_POINT('Ctrl Pts',(4.66939821170534,4.59284779079654,2.37620209998279));
#42536=CARTESIAN_POINT('Ctrl Pts',(4.82849808397002,0.483799317188488,5.14844819531533));
#42537=CARTESIAN_POINT('Ctrl Pts',(4.98759795623468,-4.06976651967716,3.19023010714429));
#42538=CARTESIAN_POINT('Ctrl Pts',(5.14669782849936,-4.88397945954014,-1.69921199567735));
#42539=CARTESIAN_POINT('Ctrl Pts',(5.30579770076401,-1.21072695590433,-5.0273964823116));
#42540=CARTESIAN_POINT('Ctrl Pts',(5.46489757302869,3.57495682182765,-3.73634277167034));
#42541=CARTESIAN_POINT('Ctrl Pts',(5.62399744529335,5.07592364569998,0.98771152242332));
#42542=CARTESIAN_POINT('Ctrl Pts',(5.78309731755802,1.91306507591506,4.80424360372137));
#42543=CARTESIAN_POINT('Ctrl Pts',(5.94219718982269,-3.00754271050209,4.20657357637889));
#42544=CARTESIAN_POINT('Ctrl Pts',(6.10129706208735,-5.16478083236238,-0.256151421987276));
#42545=CARTESIAN_POINT('Ctrl Pts',(6.26039693435203,-2.57655053740016,-4.48352114617468));
#42546=CARTESIAN_POINT('Ctrl Pts',(6.41949680661669,2.37904818745876,-4.59137280590671));
#42547=CARTESIAN_POINT('Ctrl Pts',(6.57859667888136,5.14874622778692,-0.48061089166393));
#42548=CARTESIAN_POINT('Ctrl Pts',(6.73769655114603,3.18770867422774,4.07174261783812));
#42549=CARTESIAN_POINT('Ctrl Pts',(6.8967964234107,-1.70223743368489,4.8829255836368));
#42550=CARTESIAN_POINT('Ctrl Pts',(7.05589629567536,-5.02814545322706,1.20761245470185));
#42551=CARTESIAN_POINT('Ctrl Pts',(7.21499616794003,-3.73412745548863,-3.57727084299794));
#42552=CARTESIAN_POINT('Ctrl Pts',(7.3740960402047,0.990855843724147,-5.07531075254117));
#42553=CARTESIAN_POINT('Ctrl Pts',(7.53319591246937,4.80542779279021,-1.91008854942909));
#42554=CARTESIAN_POINT('Ctrl Pts',(7.69229578473403,4.20470963362949,3.01014807526144));
#42555=CARTESIAN_POINT('Ctrl Pts',(7.8513956569987,-0.25935090699094,5.16462115214535));
#42556=CARTESIAN_POINT('Ctrl Pts',(8.01049552926338,-4.48511643133383,2.57377254931078));
#42557=CARTESIAN_POINT('Ctrl Pts',(8.16959540152803,-4.58989812922139,-2.38189204237707));
#42558=CARTESIAN_POINT('Ctrl Pts',(8.32869527379272,-0.477421201803847,
-5.14904297265438));
#42559=CARTESIAN_POINT('Ctrl Pts',(8.48779514605736,4.07371659009023,-3.18518565892236));
#42560=CARTESIAN_POINT('Ctrl Pts',(8.64689501832206,4.8818701276596,1.70526203113781));
#42561=CARTESIAN_POINT('Ctrl Pts',(8.8059948905867,1.20449733678236,5.02889259219775));
#42562=CARTESIAN_POINT('Ctrl Pts',(8.96509476285138,-3.57958341137396,3.73191065530694));
#42563=CARTESIAN_POINT('Ctrl Pts',(9.12419463511603,-5.07469595334611,-0.993999758183069));
#42564=CARTESIAN_POINT('Ctrl Pts',(9.28329450738073,-1.90711126815764,-4.80661015155663));
#42565=CARTESIAN_POINT('Ctrl Pts',(9.44239437964536,3.01275227347471,-4.20284407001334));
#42566=CARTESIAN_POINT('Ctrl Pts',(9.60149425191006,5.16445949583093,0.26255028868963));
#42567=CARTESIAN_POINT('Ctrl Pts',(9.76059412417471,2.5709935704035,4.48670999721959));
#42568=CARTESIAN_POINT('Ctrl Pts',(9.91969399643938,-2.38473498159332,4.58842169004869));
#42569=CARTESIAN_POINT('Ctrl Pts',(10.0787938687041,-5.14933774231948,0.474231329269644));
#42570=CARTESIAN_POINT('Ctrl Pts',(10.2378937409687,-3.18266142081563,-4.07568899927763));
#42571=CARTESIAN_POINT('Ctrl Pts',(10.3969936132334,1.70828597395473,-4.88081279799705));
#42572=CARTESIAN_POINT('Ctrl Pts',(10.556093485498,5.02963780132612,-1.20138175675703));
#42573=CARTESIAN_POINT('Ctrl Pts',(10.7151933577627,3.72969242293982,3.58189460618598));
#42574=CARTESIAN_POINT('Ctrl Pts',(10.8742932300274,-0.997143291267936,
5.07407920638337));
#42575=CARTESIAN_POINT('Ctrl Pts',(11.0333931022921,-4.80779066547978,1.90413325547126));
#42576=CARTESIAN_POINT('Ctrl Pts',(11.1924929745567,-4.20097689392609,-3.01535531638232));
#42577=CARTESIAN_POINT('Ctrl Pts',(11.3515928468214,0.265749570496903,-5.16429585585985));
#42578=CARTESIAN_POINT('Ctrl Pts',(11.5106927190861,4.4883018395813,-2.56821360809099));
#42579=CARTESIAN_POINT('Ctrl Pts',(11.6697925913507,4.58694349318866,2.38757701187169));
#42580=CARTESIAN_POINT('Ctrl Pts',(11.8288924636154,0.471041268600573,5.14963052385883));
#42581=CARTESIAN_POINT('Ctrl Pts',(11.9879923358801,-4.07765983257421,3.18013598426144));
#42582=CARTESIAN_POINT('Ctrl Pts',(12.1470922081447,-4.87975361780286,-1.7113093051941));
#42583=CARTESIAN_POINT('Ctrl Pts',(12.3061920804094,-1.19826567241535,-5.0303809958746));
#42584=CARTESIAN_POINT('Ctrl Pts',(12.4652919526741,3.58420434344045,-3.72747292097139));
#42585=CARTESIAN_POINT('Ctrl Pts',(12.6243918249387,5.07346067115539,1.00028675173837));
#42586=CARTESIAN_POINT('Ctrl Pts',(12.7834916972034,1.90115420721842,4.80896873992654));
#42587=CARTESIAN_POINT('Ctrl Pts',(12.9425915694681,-3.01795661773088,4.19910924514379));
#42588=CARTESIAN_POINT('Ctrl Pts',(13.1016914417327,-5.16413135425925,-0.268950934826332));
#42589=CARTESIAN_POINT('Ctrl Pts',(13.2607913139974,-2.56543051256322,-4.48988777162764));
#42590=CARTESIAN_POINT('Ctrl Pts',(13.4198911862621,2.39041400874848,-4.58547156439403));
#42591=CARTESIAN_POINT('Ctrl Pts',(13.5789910585267,5.14992922194199,-0.467835636203029));
#42592=CARTESIAN_POINT('Ctrl Pts',(13.7380909307914,3.17759419623094,4.07959959549261));
#42593=CARTESIAN_POINT('Ctrl Pts',(13.8971908030561,-1.71430297245472,4.87874912898118));
#42594=CARTESIAN_POINT('Ctrl Pts',(14.0562906753207,-5.03117786883098,1.19504069077622));
#42595=CARTESIAN_POINT('Ctrl Pts',(14.2153905475854,-3.72514538165091,-3.58630482032152));
#42596=CARTESIAN_POINT('Ctrl Pts',(14.3744904198501,1.00322544797992,-5.07323874560084));
#42597=CARTESIAN_POINT('Ctrl Pts',(14.5335902921147,4.810536850935,-1.89741011965601));
#42598=CARTESIAN_POINT('Ctrl Pts',(14.6926901643794,4.19648807260473,3.01908925610601));
#42599=CARTESIAN_POINT('Ctrl Pts',(14.8517900366441,-0.270704836412793,
5.16679883969449));
#42600=CARTESIAN_POINT('Ctrl Pts',(15.0108899089087,-4.49430009997942,2.55702559204809));
#42601=CARTESIAN_POINT('Ctrl Pts',(15.143473135796,-4.56414972861631,-1.55780334290828));
#42602=CARTESIAN_POINT('Ctrl Pts',(15.2495397173057,-2.52652896427057,-3.78487246677379));
#42603=CARTESIAN_POINT('Ctrl Pts',(15.3025730080606,-1.11832140907164,-4.28886103275609));
#42604=CARTESIAN_POINT('Ctrl Pts',(15.3290896534381,-0.392853528355804,
-4.3543139649385));
#42605=CARTESIAN_POINT('',(15.,-0.444071852043585,-4.9220081460947));
#42606=CARTESIAN_POINT('Ctrl Pts',(15.,-3.64743349744463,2.4217429795102));
#42607=CARTESIAN_POINT('Ctrl Pts',(15.,-3.7082898637292,2.34260869181596));
#42608=CARTESIAN_POINT('Ctrl Pts',(15.,-3.76611345131222,2.26145305032969));
#42609=CARTESIAN_POINT('Ctrl Pts',(15.,-3.82075032258788,2.17837970357634));
#42610=CARTESIAN_POINT('Ctrl Pts',(15.,-3.89159249211755,2.07066679877978));
#42611=CARTESIAN_POINT('Ctrl Pts',(15.,-3.95707930631556,1.95973124308563));
#42612=CARTESIAN_POINT('Ctrl Pts',(15.,-4.0172930750217,1.84600005851335));
#42613=CARTESIAN_POINT('Ctrl Pts',(15.,-4.07888289152636,1.72966980815403));
#42614=CARTESIAN_POINT('Ctrl Pts',(15.,-4.13495615398629,1.61041413582088));
#42615=CARTESIAN_POINT('Ctrl Pts',(15.,-4.18555885319492,1.48865487734055));
#42616=CARTESIAN_POINT('Ctrl Pts',(15.,-4.23700268046163,1.36487171242361));
#42617=CARTESIAN_POINT('Ctrl Pts',(15.,-4.28279281221221,1.23850035311616));
#42618=CARTESIAN_POINT('Ctrl Pts',(15.,-4.32293081471277,1.10995769229629));
#42619=CARTESIAN_POINT('Ctrl Pts',(15.,-4.33504493319114,1.07116201424341));
#42620=CARTESIAN_POINT('Ctrl Pts',(15.,-4.34664386538786,1.03216841226631));
#42621=CARTESIAN_POINT('Ctrl Pts',(15.,-4.35772678427811,0.992988037261006));
#42622=CARTESIAN_POINT('Ctrl Pts',(15.,-4.36488134209109,0.967695218565394));
#42623=CARTESIAN_POINT('Ctrl Pts',(15.,-4.3718208521776,0.942324563071167));
#42624=CARTESIAN_POINT('Ctrl Pts',(15.,-4.37854500096099,0.916879049181161));
#42625=CARTESIAN_POINT('Ctrl Pts',(15.,-4.38421840264999,0.895409770893104));
#42626=CARTESIAN_POINT('Ctrl Pts',(15.,-4.38973902219339,0.873884734398618));
#42627=CARTESIAN_POINT('Ctrl Pts',(15.,-4.3951011031017,0.852328924497718));
#42628=CARTESIAN_POINT('Ctrl Pts',(15.,-4.42797349404255,0.720180413084934));
#42629=CARTESIAN_POINT('Ctrl Pts',(15.,-4.45494081833527,0.58669596358257));
#42630=CARTESIAN_POINT('Ctrl Pts',(15.,-4.47607666705785,0.452331314099685));
#42631=CARTESIAN_POINT('Ctrl Pts',(15.,-4.49752457608506,0.315982837328957));
#42632=CARTESIAN_POINT('Ctrl Pts',(15.,-4.51296775060728,0.178727229649941));
#42633=CARTESIAN_POINT('Ctrl Pts',(15.,-4.52243514398287,0.0410146220670506));
#42634=CARTESIAN_POINT('Ctrl Pts',(15.,-4.53194192100607,-0.0972708596527243));
#42635=CARTESIAN_POINT('Ctrl Pts',(15.,-4.53542324150019,-0.236017985118476));
#42636=CARTESIAN_POINT('Ctrl Pts',(15.,-4.53285786554154,-0.374785067473027));
#42637=CARTESIAN_POINT('Ctrl Pts',(15.,-4.53031342129,-0.512419905676942));
#42638=CARTESIAN_POINT('Ctrl Pts',(15.,-4.52182060592257,-0.650075216592292));
#42639=CARTESIAN_POINT('Ctrl Pts',(15.,-4.50730773271262,-0.787321336183077));
#42640=CARTESIAN_POINT('Ctrl Pts',(15.,-4.50515840901136,-0.807647176109848));
#42641=CARTESIAN_POINT('Ctrl Pts',(15.,-4.50287695500964,-0.82796403036086));
#42642=CARTESIAN_POINT('Ctrl Pts',(15.,-4.50046304054395,-0.848270488261463));
#42643=CARTESIAN_POINT('Ctrl Pts',(15.,-4.49855407636242,-0.864329176892247));
#42644=CARTESIAN_POINT('Ctrl Pts',(15.,-4.49656237244444,-0.880380229709894));
#42645=CARTESIAN_POINT('Ctrl Pts',(15.,-4.49448916865398,-0.896413081113118));
#42646=CARTESIAN_POINT('Ctrl Pts',(15.,-4.47634947236908,-1.03669405897637));
#42647=CARTESIAN_POINT('Ctrl Pts',(15.,-4.4519508282184,-1.17578554412336));
#42648=CARTESIAN_POINT('Ctrl Pts',(15.,-4.42132243491177,-1.3132290481336));
#42649=CARTESIAN_POINT('Ctrl Pts',(15.,-4.39075380118495,-1.45040438378239));
#42650=CARTESIAN_POINT('Ctrl Pts',(15.,-4.35397977833926,-1.58593903131621));
#42651=CARTESIAN_POINT('Ctrl Pts',(15.,-4.31097798157061,-1.71938254118705));
#42652=CARTESIAN_POINT('Ctrl Pts',(15.,-4.2687043897354,-1.85056627985004));
#42653=CARTESIAN_POINT('Ctrl Pts',(15.,-4.22041211971183,-1.97972990602547));
#42654=CARTESIAN_POINT('Ctrl Pts',(15.,-4.16603015137339,-2.10643831260173));
#42655=CARTESIAN_POINT('Ctrl Pts',(15.,-4.15802001293815,-2.12510170248253));
#42656=CARTESIAN_POINT('Ctrl Pts',(15.,-4.14987766647486,-2.14371179984538));
#42657=CARTESIAN_POINT('Ctrl Pts',(15.,-4.14160279252619,-2.16226718465083));
#42658=CARTESIAN_POINT('Ctrl Pts',(15.,-4.10146980039451,-2.25226047240565));
#42659=CARTESIAN_POINT('Ctrl Pts',(15.,-4.05822043039043,-2.34096727307218));
#42660=CARTESIAN_POINT('Ctrl Pts',(15.,-4.01198020214139,-2.42828555150392));
#42661=CARTESIAN_POINT('Ctrl Pts',(15.,-3.99642623237433,-2.45765707310465));
#42662=CARTESIAN_POINT('Ctrl Pts',(15.,-3.98053375519778,-2.48687143593773));
#42663=CARTESIAN_POINT('Ctrl Pts',(15.,-3.96430725035697,-2.51592458767279));
#42664=CARTESIAN_POINT('Ctrl Pts',(15.,-3.95490325737157,-2.53276220229163));
#42665=CARTESIAN_POINT('Ctrl Pts',(15.,-3.94538617715611,-2.54954721951204));
#42666=CARTESIAN_POINT('Ctrl Pts',(15.,-3.93575967760122,-2.56627394730149));
#42667=CARTESIAN_POINT('Ctrl Pts',(15.,-3.86759024667037,-2.68472318300139));
#42668=CARTESIAN_POINT('Ctrl Pts',(15.,-3.79413538181915,-2.79990975721909));
#42669=CARTESIAN_POINT('Ctrl Pts',(15.,-3.71581656760059,-2.9116041082618));
#42670=CARTESIAN_POINT('Ctrl Pts',(15.,-3.63503278498645,-3.02681387316811));
#42671=CARTESIAN_POINT('Ctrl Pts',(15.,-3.5490737856704,-3.13830875738446));
#42672=CARTESIAN_POINT('Ctrl Pts',(15.,-3.45834874984291,-3.24582141311442));
#42673=CARTESIAN_POINT('Ctrl Pts',(15.,-3.36674247041888,-3.35437837638909));
#42674=CARTESIAN_POINT('Ctrl Pts',(15.,-3.2702766055505,-3.45887601759371));
#42675=CARTESIAN_POINT('Ctrl Pts',(15.,-3.16932511812227,-3.55901400521376));
#42676=CARTESIAN_POINT('Ctrl Pts',(15.,-3.09115822859782,-3.63655100060535));
#42677=CARTESIAN_POINT('Ctrl Pts',(15.,-3.01030098340661,-3.71147378219999));
#42678=CARTESIAN_POINT('Ctrl Pts',(15.,-2.92691083995722,-3.78362897614142));
#42679=CARTESIAN_POINT('Ctrl Pts',(15.,-2.88521576823253,-3.81970657311214));
#42680=CARTESIAN_POINT('Ctrl Pts',(15.,-2.84288727059802,-3.85509206296282));
#42681=CARTESIAN_POINT('Ctrl Pts',(15.,-2.79994392620086,-3.88976489887852));
#42682=CARTESIAN_POINT('Ctrl Pts',(15.,-2.77692979182587,-3.90834671443407));
#42683=CARTESIAN_POINT('Ctrl Pts',(15.,-2.75373905644439,-3.92672383301606));
#42684=CARTESIAN_POINT('Ctrl Pts',(15.,-2.73037450355138,-3.94489297201166));
#42685=CARTESIAN_POINT('Ctrl Pts',(15.,-2.71464882485127,-3.95712184039235));
#42686=CARTESIAN_POINT('Ctrl Pts',(15.,-2.69885251683566,-3.96925018247846));
#42687=CARTESIAN_POINT('Ctrl Pts',(15.,-2.68298667657367,-3.9812772548001));
#42688=CARTESIAN_POINT('Ctrl Pts',(15.,-2.67843952821254,-3.98472421262228));
#42689=CARTESIAN_POINT('Ctrl Pts',(15.,-2.67388666838095,-3.98816285215109));
#42690=CARTESIAN_POINT('Ctrl Pts',(15.,-2.66932812263831,-3.99159315574737));
#42691=CARTESIAN_POINT('Ctrl Pts',(15.,-2.55443810398459,-4.07804784248627));
#42692=CARTESIAN_POINT('Ctrl Pts',(15.,-2.43593971533117,-4.15921041969436));
#42693=CARTESIAN_POINT('Ctrl Pts',(15.,-2.31421368015325,-4.23496729168326));
#42694=CARTESIAN_POINT('Ctrl Pts',(15.,-2.19161738873209,-4.31126577246374));
#42695=CARTESIAN_POINT('Ctrl Pts',(15.,-2.06574656365596,-4.38208139752043));
#42696=CARTESIAN_POINT('Ctrl Pts',(15.,-1.93695462293276,-4.44725913313952));
#42697=CARTESIAN_POINT('Ctrl Pts',(15.,-1.87847558199184,-4.47685362056088));
#42698=CARTESIAN_POINT('Ctrl Pts',(15.,-1.81939386822387,-4.50528518256321));
#42699=CARTESIAN_POINT('Ctrl Pts',(15.,-1.75974066697738,-4.53253631662746));
#42700=CARTESIAN_POINT('Ctrl Pts',(15.,-1.72832141961374,-4.54688944611948));
#42701=CARTESIAN_POINT('Ctrl Pts',(15.,-1.69674361756834,-4.56091507907796));
#42702=CARTESIAN_POINT('Ctrl Pts',(15.,-1.66501170956427,-4.57461043436351));
#42703=CARTESIAN_POINT('Ctrl Pts',(15.,-1.64184014412444,-4.58461118254354));
#42704=CARTESIAN_POINT('Ctrl Pts',(15.,-1.6185938221782,-4.59443257119121));
#42705=CARTESIAN_POINT('Ctrl Pts',(15.,-1.59528099966613,-4.60407127664067));
#42706=CARTESIAN_POINT('Ctrl Pts',(15.,-1.46028192957332,-4.65988675208995));
#42707=CARTESIAN_POINT('Ctrl Pts',(15.,-1.32298927848311,-4.70960834354769));
#42708=CARTESIAN_POINT('Ctrl Pts',(15.,-1.18377213314752,-4.75309202784066));
#42709=CARTESIAN_POINT('Ctrl Pts',(15.,-1.04542344044048,-4.79630445588977));
#42710=CARTESIAN_POINT('Ctrl Pts',(15.,-0.90517353780007,-4.83335688725323));
#42711=CARTESIAN_POINT('Ctrl Pts',(15.,-0.763360003752109,-4.86406332913526));
#42712=CARTESIAN_POINT('Ctrl Pts',(15.,-0.657753741735435,-4.88692992341883));
#42713=CARTESIAN_POINT('Ctrl Pts',(15.,-0.551279803770889,-4.90627644088498));
#42714=CARTESIAN_POINT('Ctrl Pts',(15.,-0.444071852043585,-4.9220081460947));
#42715=CARTESIAN_POINT('Ctrl Pts',(15.,-0.444071852043585,-4.9220081460947));
#42716=CARTESIAN_POINT('Ctrl Pts',(14.9734833546226,-1.26412269067527,-4.84802178039354));
#42717=CARTESIAN_POINT('Ctrl Pts',(14.9469667092451,-2.06002407880351,-4.56317371393828));
#42718=CARTESIAN_POINT('Ctrl Pts',(14.9204500638677,-2.74588424843362,-4.10607174126237));
#42719=CARTESIAN_POINT('Ctrl Pts',(14.8939334184902,-3.43174441806373,-3.64896976858645));
#42720=CARTESIAN_POINT('Ctrl Pts',(14.8674167731128,-4.00756336919571,-3.01961388968989));
#42721=CARTESIAN_POINT('Ctrl Pts',(14.8409001277353,-4.3861789178198,-2.28995662189616));
#42722=CARTESIAN_POINT('Ctrl Pts',(14.8153735700425,-4.75065758802023,-1.58754354976006));
#42723=CARTESIAN_POINT('Ctrl Pts',(14.7898470123497,-4.93238442199734,-0.792179429297219));
#42724=CARTESIAN_POINT('Ctrl Pts',(14.7643204546569,-4.93235156762733,0.00248647065513752));
#42725=CARTESIAN_POINT('Origin',(15.,4.,0.));
#42726=CARTESIAN_POINT('Origin',(15.,0.,0.));
#42727=CARTESIAN_POINT('',(15.,-4.,-4.89858719658941E-16));
#42728=CARTESIAN_POINT('Origin',(15.,0.,0.));
#42729=CARTESIAN_POINT('Ctrl Pts',(26.5,4.59649122554347,-5.29039824318981));
#42730=CARTESIAN_POINT('Ctrl Pts',(26.25,4.59649122554347,-5.29039824318981));
#42731=CARTESIAN_POINT('Ctrl Pts',(26.5,4.91129522759113,-5.10151584196121));
#42732=CARTESIAN_POINT('Ctrl Pts',(26.25,4.91129522759113,-5.10151584196121));
#42733=CARTESIAN_POINT('Ctrl Pts',(26.5,5.25043192007604,-5.1048615648549));
#42734=CARTESIAN_POINT('Ctrl Pts',(26.25,5.25043192007604,-5.1048615648549));
#42735=CARTESIAN_POINT('',(26.5,4.59649122554347,-5.29039824318981));
#42736=CARTESIAN_POINT('',(26.5,5.25043192007604,-5.1048615648549));
#42737=CARTESIAN_POINT('Ctrl Pts',(26.5,4.59649122554347,-5.29039824318981));
#42738=CARTESIAN_POINT('Ctrl Pts',(26.5,4.91129522759113,-5.10151584196121));
#42739=CARTESIAN_POINT('Ctrl Pts',(26.5,5.25043192007604,-5.1048615648549));
#42740=CARTESIAN_POINT('',(26.25,4.59649122554347,-5.29039824318981));
#42741=CARTESIAN_POINT('',(26.5,4.59649122554347,-5.29039824318981));
#42742=CARTESIAN_POINT('',(26.25,5.25043192007604,-5.1048615648549));
#42743=CARTESIAN_POINT('Ctrl Pts',(26.25,4.59649122554347,-5.29039824318981));
#42744=CARTESIAN_POINT('Ctrl Pts',(26.25,4.91129522759113,-5.10151584196121));
#42745=CARTESIAN_POINT('Ctrl Pts',(26.25,5.25043192007604,-5.1048615648549));
#42746=CARTESIAN_POINT('',(26.5,5.25043192007604,-5.1048615648549));
#42747=CARTESIAN_POINT('Ctrl Pts',(26.5,4.13766826737842,-5.75287126208542));
#42748=CARTESIAN_POINT('Ctrl Pts',(26.25,4.13766826737842,-5.75287126208542));
#42749=CARTESIAN_POINT('Ctrl Pts',(26.5,4.30601993948832,-5.46468101482289));
#42750=CARTESIAN_POINT('Ctrl Pts',(26.25,4.30601993948832,-5.46468101482289));
#42751=CARTESIAN_POINT('Ctrl Pts',(26.5,4.59649122554347,-5.29039824318981));
#42752=CARTESIAN_POINT('Ctrl Pts',(26.25,4.59649122554347,-5.29039824318981));
#42753=CARTESIAN_POINT('',(26.5,4.13766826737842,-5.75287126208542));
#42754=CARTESIAN_POINT('Ctrl Pts',(26.5,4.13766826737842,-5.75287126208542));
#42755=CARTESIAN_POINT('Ctrl Pts',(26.5,4.30601993948832,-5.46468101482289));
#42756=CARTESIAN_POINT('Ctrl Pts',(26.5,4.59649122554347,-5.29039824318981));
#42757=CARTESIAN_POINT('',(26.25,4.13766826737842,-5.75287126208542));
#42758=CARTESIAN_POINT('',(26.5,4.13766826737842,-5.75287126208542));
#42759=CARTESIAN_POINT('Ctrl Pts',(26.25,4.13766826737842,-5.75287126208542));
#42760=CARTESIAN_POINT('Ctrl Pts',(26.25,4.30601993948832,-5.46468101482289));
#42761=CARTESIAN_POINT('Ctrl Pts',(26.25,4.59649122554347,-5.29039824318981));
#42762=CARTESIAN_POINT('Ctrl Pts',(26.5,3.99304081447426,-6.39084371396902));
#42763=CARTESIAN_POINT('Ctrl Pts',(26.25,3.99304081447426,-6.39084371396902));
#42764=CARTESIAN_POINT('Ctrl Pts',(26.5,3.96931659526851,-6.04106150934795));
#42765=CARTESIAN_POINT('Ctrl Pts',(26.25,3.96931659526851,-6.04106150934795));
#42766=CARTESIAN_POINT('Ctrl Pts',(26.5,4.13766826737842,-5.75287126208542));
#42767=CARTESIAN_POINT('Ctrl Pts',(26.25,4.13766826737842,-5.75287126208542));
#42768=CARTESIAN_POINT('',(26.5,3.99304081447426,-6.39084371396902));
#42769=CARTESIAN_POINT('Ctrl Pts',(26.5,3.99304081447426,-6.39084371396902));
#42770=CARTESIAN_POINT('Ctrl Pts',(26.5,3.96931659526851,-6.04106150934795));
#42771=CARTESIAN_POINT('Ctrl Pts',(26.5,4.13766826737842,-5.75287126208542));
#42772=CARTESIAN_POINT('',(26.25,3.99304081447426,-6.39084371396902));
#42773=CARTESIAN_POINT('',(26.5,3.99304081447426,-6.39084371396902));
#42774=CARTESIAN_POINT('Ctrl Pts',(26.25,3.99304081447426,-6.39084371396902));
#42775=CARTESIAN_POINT('Ctrl Pts',(26.25,3.96931659526851,-6.04106150934795));
#42776=CARTESIAN_POINT('Ctrl Pts',(26.25,4.13766826737842,-5.75287126208542));
#42777=CARTESIAN_POINT('Ctrl Pts',(26.5,4.22024719228052,-7.07976255996445));
#42778=CARTESIAN_POINT('Ctrl Pts',(26.25,4.22024719228052,-7.07976255996445));
#42779=CARTESIAN_POINT('Ctrl Pts',(26.5,4.01676516145641,-6.74062584192426));
#42780=CARTESIAN_POINT('Ctrl Pts',(26.25,4.01676516145641,-6.74062584192426));
#42781=CARTESIAN_POINT('Ctrl Pts',(26.5,3.99304081447426,-6.39084371396902));
#42782=CARTESIAN_POINT('Ctrl Pts',(26.25,3.99304081447426,-6.39084371396902));
#42783=CARTESIAN_POINT('',(26.5,4.22024719228052,-7.07976255996445));
#42784=CARTESIAN_POINT('Ctrl Pts',(26.5,4.22024719228052,-7.07976255996445));
#42785=CARTESIAN_POINT('Ctrl Pts',(26.5,4.01676516145641,-6.74062584192426));
#42786=CARTESIAN_POINT('Ctrl Pts',(26.5,3.99304081447426,-6.39084371396902));
#42787=CARTESIAN_POINT('',(26.25,4.22024719228052,-7.07976255996445));
#42788=CARTESIAN_POINT('',(26.5,4.22024719228052,-7.07976255996445));
#42789=CARTESIAN_POINT('Ctrl Pts',(26.25,4.22024719228052,-7.07976255996445));
#42790=CARTESIAN_POINT('Ctrl Pts',(26.25,4.01676516145641,-6.74062584192426));
#42791=CARTESIAN_POINT('Ctrl Pts',(26.25,3.99304081447426,-6.39084371396902));
#42792=CARTESIAN_POINT('Ctrl Pts',(26.5,4.70933386374015,-7.60017785881726));
#42793=CARTESIAN_POINT('Ctrl Pts',(26.25,4.70933386374015,-7.60017785881726));
#42794=CARTESIAN_POINT('Ctrl Pts',(26.5,4.42099179255547,-7.41433689375604));
#42795=CARTESIAN_POINT('Ctrl Pts',(26.25,4.42099179255547,-7.41433689375604));
#42796=CARTESIAN_POINT('Ctrl Pts',(26.5,4.22024719228052,-7.07976255996445));
#42797=CARTESIAN_POINT('Ctrl Pts',(26.25,4.22024719228052,-7.07976255996445));
#42798=CARTESIAN_POINT('',(26.5,4.70933386374015,-7.60017785881726));
#42799=CARTESIAN_POINT('Ctrl Pts',(26.5,4.70933386374015,-7.60017785881726));
#42800=CARTESIAN_POINT('Ctrl Pts',(26.5,4.42099179255547,-7.41433689375604));
#42801=CARTESIAN_POINT('Ctrl Pts',(26.5,4.22024719228052,-7.07976255996445));
#42802=CARTESIAN_POINT('',(26.25,4.70933386374015,-7.60017785881726));
#42803=CARTESIAN_POINT('',(26.5,4.70933386374015,-7.60017785881726));
#42804=CARTESIAN_POINT('Ctrl Pts',(26.25,4.70933386374015,-7.60017785881726));
#42805=CARTESIAN_POINT('Ctrl Pts',(26.25,4.42099179255547,-7.41433689375604));
#42806=CARTESIAN_POINT('Ctrl Pts',(26.25,4.22024719228052,-7.07976255996445));
#42807=CARTESIAN_POINT('Ctrl Pts',(26.5,5.33407558018978,-7.78480193252604));
#42808=CARTESIAN_POINT('Ctrl Pts',(26.25,5.33407558018978,-7.78480193252604));
#42809=CARTESIAN_POINT('Ctrl Pts',(26.5,4.99767624158819,-7.78601846610455));
#42810=CARTESIAN_POINT('Ctrl Pts',(26.25,4.99767624158819,-7.78601846610455));
#42811=CARTESIAN_POINT('Ctrl Pts',(26.5,4.70933386374015,-7.60017785881726));
#42812=CARTESIAN_POINT('Ctrl Pts',(26.25,4.70933386374015,-7.60017785881726));
#42813=CARTESIAN_POINT('',(26.5,5.33407558018978,-7.78480193252604));
#42814=CARTESIAN_POINT('Ctrl Pts',(26.5,5.33407558018978,-7.78480193252604));
#42815=CARTESIAN_POINT('Ctrl Pts',(26.5,4.99767624158819,-7.78601846610455));
#42816=CARTESIAN_POINT('Ctrl Pts',(26.5,4.70933386374015,-7.60017785881726));
#42817=CARTESIAN_POINT('',(26.25,5.33407558018978,-7.78480193252604));
#42818=CARTESIAN_POINT('',(26.5,5.33407558018978,-7.78480193252604));
#42819=CARTESIAN_POINT('Ctrl Pts',(26.25,5.33407558018978,-7.78480193252604));
#42820=CARTESIAN_POINT('Ctrl Pts',(26.25,4.99767624158819,-7.78601846610455));
#42821=CARTESIAN_POINT('Ctrl Pts',(26.25,4.70933386374015,-7.60017785881726));
#42822=CARTESIAN_POINT('Ctrl Pts',(26.5,5.97919566517507,-7.59835277734141));
#42823=CARTESIAN_POINT('Ctrl Pts',(26.25,5.97919566517507,-7.59835277734141));
#42824=CARTESIAN_POINT('Ctrl Pts',(26.5,5.67047484212553,-7.78358527117114));
#42825=CARTESIAN_POINT('Ctrl Pts',(26.25,5.67047484212553,-7.78358527117114));
#42826=CARTESIAN_POINT('Ctrl Pts',(26.5,5.33407558018978,-7.78480193252604));
#42827=CARTESIAN_POINT('Ctrl Pts',(26.25,5.33407558018978,-7.78480193252604));
#42828=CARTESIAN_POINT('',(26.5,5.97919566517507,-7.59835277734141));
#42829=CARTESIAN_POINT('Ctrl Pts',(26.5,5.97919566517507,-7.59835277734141));
#42830=CARTESIAN_POINT('Ctrl Pts',(26.5,5.67047484212553,-7.78358527117114));
#42831=CARTESIAN_POINT('Ctrl Pts',(26.5,5.33407558018978,-7.78480193252604));
#42832=CARTESIAN_POINT('',(26.25,5.97919566517507,-7.59835277734141));
#42833=CARTESIAN_POINT('',(26.5,5.97919566517507,-7.59835277734141));
#42834=CARTESIAN_POINT('Ctrl Pts',(26.25,5.97919566517507,-7.59835277734141));
#42835=CARTESIAN_POINT('Ctrl Pts',(26.25,5.67047484212553,-7.78358527117114));
#42836=CARTESIAN_POINT('Ctrl Pts',(26.25,5.33407558018978,-7.78480193252604));
#42837=CARTESIAN_POINT('Ctrl Pts',(26.5,6.56029043175907,-6.82259661503587));
#42838=CARTESIAN_POINT('Ctrl Pts',(26.25,6.56029043175907,-6.82259661503587));
#42839=CARTESIAN_POINT('Ctrl Pts',(26.5,6.45064133476,-7.31548537559045));
#42840=CARTESIAN_POINT('Ctrl Pts',(26.25,6.45064133476,-7.31548537559045));
#42841=CARTESIAN_POINT('Ctrl Pts',(26.5,5.97919566517507,-7.59835277734141));
#42842=CARTESIAN_POINT('Ctrl Pts',(26.25,5.97919566517507,-7.59835277734141));
#42843=CARTESIAN_POINT('',(26.5,6.56029043175907,-6.82259661503587));
#42844=CARTESIAN_POINT('Ctrl Pts',(26.5,6.56029043175907,-6.82259661503587));
#42845=CARTESIAN_POINT('Ctrl Pts',(26.5,6.45064133476,-7.31548537559045));
#42846=CARTESIAN_POINT('Ctrl Pts',(26.5,5.97919566517507,-7.59835277734141));
#42847=CARTESIAN_POINT('',(26.25,6.56029043175907,-6.82259661503587));
#42848=CARTESIAN_POINT('',(26.5,6.56029043175907,-6.82259661503587));
#42849=CARTESIAN_POINT('Ctrl Pts',(26.25,6.56029043175907,-6.82259661503587));
#42850=CARTESIAN_POINT('Ctrl Pts',(26.25,6.45064133476,-7.31548537559045));
#42851=CARTESIAN_POINT('Ctrl Pts',(26.25,5.97919566517507,-7.59835277734141));
#42852=CARTESIAN_POINT('Ctrl Pts',(26.5,6.33688598652166,-5.77461850881057));
#42853=CARTESIAN_POINT('Ctrl Pts',(26.25,6.33688598652166,-5.77461850881057));
#42854=CARTESIAN_POINT('Ctrl Pts',(26.5,6.66993957667428,-6.3297078257316));
#42855=CARTESIAN_POINT('Ctrl Pts',(26.25,6.66993957667428,-6.3297078257316));
#42856=CARTESIAN_POINT('Ctrl Pts',(26.5,6.56029043175907,-6.82259661503587));
#42857=CARTESIAN_POINT('Ctrl Pts',(26.25,6.56029043175907,-6.82259661503587));
#42858=CARTESIAN_POINT('',(26.5,6.33688598652166,-5.77461850881057));
#42859=CARTESIAN_POINT('Ctrl Pts',(26.5,6.33688598652166,-5.77461850881057));
#42860=CARTESIAN_POINT('Ctrl Pts',(26.5,6.66993957667428,-6.3297078257316));
#42861=CARTESIAN_POINT('Ctrl Pts',(26.5,6.56029043175907,-6.82259661503587));
#42862=CARTESIAN_POINT('',(26.25,6.33688598652166,-5.77461850881057));
#42863=CARTESIAN_POINT('',(26.5,6.33688598652166,-5.77461850881057));
#42864=CARTESIAN_POINT('Ctrl Pts',(26.25,6.33688598652166,-5.77461850881057));
#42865=CARTESIAN_POINT('Ctrl Pts',(26.25,6.66993957667428,-6.3297078257316));
#42866=CARTESIAN_POINT('Ctrl Pts',(26.25,6.56029043175907,-6.82259661503587));
#42867=CARTESIAN_POINT('Ctrl Pts',(26.5,5.87517352152691,-5.29465658348726));
#42868=CARTESIAN_POINT('Ctrl Pts',(26.25,5.87517352152691,-5.29465658348726));
#42869=CARTESIAN_POINT('Ctrl Pts',(26.5,6.16077826118914,-5.48110563325636));
#42870=CARTESIAN_POINT('Ctrl Pts',(26.25,6.16077826118914,-5.48110563325636));
#42871=CARTESIAN_POINT('Ctrl Pts',(26.5,6.33688598652166,-5.77461850881057));
#42872=CARTESIAN_POINT('Ctrl Pts',(26.25,6.33688598652166,-5.77461850881057));
#42873=CARTESIAN_POINT('',(26.5,5.87517352152691,-5.29465658348726));
#42874=CARTESIAN_POINT('Ctrl Pts',(26.5,5.87517352152691,-5.29465658348726));
#42875=CARTESIAN_POINT('Ctrl Pts',(26.5,6.16077826118914,-5.48110563325636));
#42876=CARTESIAN_POINT('Ctrl Pts',(26.5,6.33688598652166,-5.77461850881057));
#42877=CARTESIAN_POINT('',(26.25,5.87517352152691,-5.29465658348726));
#42878=CARTESIAN_POINT('',(26.5,5.87517352152691,-5.29465658348726));
#42879=CARTESIAN_POINT('Ctrl Pts',(26.25,5.87517352152691,-5.29465658348726));
#42880=CARTESIAN_POINT('Ctrl Pts',(26.25,6.16077826118914,-5.48110563325636));
#42881=CARTESIAN_POINT('Ctrl Pts',(26.25,6.33688598652166,-5.77461850881057));
#42882=CARTESIAN_POINT('Ctrl Pts',(26.5,5.25043192007604,-5.1048615648549));
#42883=CARTESIAN_POINT('Ctrl Pts',(26.25,5.25043192007604,-5.1048615648549));
#42884=CARTESIAN_POINT('Ctrl Pts',(26.5,5.58956861256095,-5.10820728774859));
#42885=CARTESIAN_POINT('Ctrl Pts',(26.25,5.58956861256095,-5.10820728774859));
#42886=CARTESIAN_POINT('Ctrl Pts',(26.5,5.87517352152691,-5.29465658348726));
#42887=CARTESIAN_POINT('Ctrl Pts',(26.25,5.87517352152691,-5.29465658348726));
#42888=CARTESIAN_POINT('Ctrl Pts',(26.5,5.25043192007604,-5.1048615648549));
#42889=CARTESIAN_POINT('Ctrl Pts',(26.5,5.58956861256095,-5.10820728774859));
#42890=CARTESIAN_POINT('Ctrl Pts',(26.5,5.87517352152691,-5.29465658348726));
#42891=CARTESIAN_POINT('Ctrl Pts',(26.25,5.25043192007604,-5.1048615648549));
#42892=CARTESIAN_POINT('Ctrl Pts',(26.25,5.58956861256095,-5.10820728774859));
#42893=CARTESIAN_POINT('Ctrl Pts',(26.25,5.87517352152691,-5.29465658348726));
#42894=CARTESIAN_POINT('Origin',(26.25,5.3196280859714,-6.44376715403288));
#42895=CARTESIAN_POINT('Origin',(26.5,1.72219374887709,-7.06668375067375));
#42896=CARTESIAN_POINT('',(26.5,1.72219374887709,-7.06668375067375));
#42897=CARTESIAN_POINT('',(26.5,3.94437549748797,-8.11603042842518));
#42898=CARTESIAN_POINT('',(26.5,-0.346179236230716,-6.0899678175011));
#42899=CARTESIAN_POINT('',(26.25,1.72219374887709,-7.06668375067375));
#42900=CARTESIAN_POINT('',(26.5,1.72219374887709,-7.06668375067375));
#42901=CARTESIAN_POINT('',(26.25,3.94437549748797,-8.11603042842518));
#42902=CARTESIAN_POINT('',(26.25,1.72219374887709,-7.06668375067375));
#42903=CARTESIAN_POINT('',(26.5,3.94437549748797,-8.11603042842518));
#42904=CARTESIAN_POINT('Origin',(26.5,1.41955597704928,-7.24826641377043));
#42905=CARTESIAN_POINT('',(26.5,1.41955597704928,-7.24826641377043));
#42906=CARTESIAN_POINT('',(26.5,2.496542694407,-6.6020743833558));
#42907=CARTESIAN_POINT('',(26.25,1.41955597704928,-7.24826641377043));
#42908=CARTESIAN_POINT('',(26.5,1.41955597704928,-7.24826641377043));
#42909=CARTESIAN_POINT('',(26.25,1.41955597704928,-7.24826641377043));
#42910=CARTESIAN_POINT('Origin',(26.5,2.75724489209471,-9.47774793884615));
#42911=CARTESIAN_POINT('',(26.5,2.75724489209471,-9.47774793884615));
#42912=CARTESIAN_POINT('',(26.5,0.301635728689645,-5.3850659998377));
#42913=CARTESIAN_POINT('',(26.25,2.75724489209471,-9.47774793884615));
#42914=CARTESIAN_POINT('',(26.5,2.75724489209471,-9.47774793884615));
#42915=CARTESIAN_POINT('',(26.25,2.75724489209471,-9.47774793884615));
#42916=CARTESIAN_POINT('Origin',(26.5,3.04011233217859,-9.30802747479582));
#42917=CARTESIAN_POINT('',(26.5,3.04011233217859,-9.30802747479582));
#42918=CARTESIAN_POINT('',(26.5,3.97566532949436,-8.74669567640636));
#42919=CARTESIAN_POINT('',(26.25,3.04011233217859,-9.30802747479582));
#42920=CARTESIAN_POINT('',(26.5,3.04011233217859,-9.30802747479582));
#42921=CARTESIAN_POINT('',(26.25,3.04011233217859,-9.30802747479582));
#42922=CARTESIAN_POINT('Origin',(26.5,1.9898531647998,-7.5575955291645));
#42923=CARTESIAN_POINT('',(26.5,1.9898531647998,-7.5575955291645));
#42924=CARTESIAN_POINT('',(26.5,0.05937358508413,-4.34012956297171));
#42925=CARTESIAN_POINT('',(26.25,1.9898531647998,-7.5575955291645));
#42926=CARTESIAN_POINT('',(26.5,1.9898531647998,-7.5575955291645));
#42927=CARTESIAN_POINT('',(26.25,1.9898531647998,-7.5575955291645));
#42928=CARTESIAN_POINT('Origin',(26.5,4.21112243656096,-8.6054214121664));
#42929=CARTESIAN_POINT('',(26.5,4.21112243656096,-8.6054214121664));
#42930=CARTESIAN_POINT('',(26.5,0.828567464789562,-7.00978926834771));
#42931=CARTESIAN_POINT('',(26.25,4.21112243656096,-8.6054214121664));
#42932=CARTESIAN_POINT('',(26.5,4.21112243656096,-8.6054214121664));
#42933=CARTESIAN_POINT('',(26.25,4.21112243656096,-8.6054214121664));
#42934=CARTESIAN_POINT('Origin',(26.5,4.51376012852852,-8.42383879698586));
#42935=CARTESIAN_POINT('',(26.5,4.51376012852852,-8.42383879698586));
#42936=CARTESIAN_POINT('',(26.5,4.71248922766934,-8.30460133750137));
#42937=CARTESIAN_POINT('',(26.25,4.51376012852852,-8.42383879698586));
#42938=CARTESIAN_POINT('',(26.5,4.51376012852852,-8.42383879698586));
#42939=CARTESIAN_POINT('',(26.25,4.51376012852852,-8.42383879698586));
#42940=CARTESIAN_POINT('Origin',(26.5,3.17607121348309,-6.19435727191015));
#42941=CARTESIAN_POINT('',(26.5,3.17607121348309,-6.19435727191015));
#42942=CARTESIAN_POINT('',(26.5,1.38930650760073,-3.21641609543956));
#42943=CARTESIAN_POINT('',(26.25,3.17607121348309,-6.19435727191015));
#42944=CARTESIAN_POINT('',(26.5,3.17607121348309,-6.19435727191015));
#42945=CARTESIAN_POINT('',(26.25,3.17607121348309,-6.19435727191015));
#42946=CARTESIAN_POINT('Origin',(26.5,2.89320385325946,-6.36407768804433));
#42947=CARTESIAN_POINT('',(26.5,2.89320385325946,-6.36407768804433));
#42948=CARTESIAN_POINT('',(26.5,3.23336663251209,-6.15998002049275));
#42949=CARTESIAN_POINT('',(26.25,2.89320385325946,-6.36407768804433));
#42950=CARTESIAN_POINT('',(26.5,2.89320385325946,-6.36407768804433));
#42951=CARTESIAN_POINT('',(26.25,2.89320385325946,-6.36407768804433));
#42952=CARTESIAN_POINT('Origin',(26.5,3.94437549748797,-8.11603042842518));
#42953=CARTESIAN_POINT('',(26.5,1.63202496949136,-4.26211288176416));
#42954=CARTESIAN_POINT('',(26.25,3.94437549748797,-8.11603042842518));
#42955=CARTESIAN_POINT('Origin',(26.25,2.9666580527889,-7.83605260537815));
#42956=CARTESIAN_POINT('Ctrl Pts',(26.5,0.501266317583819,6.69979499726322));
#42957=CARTESIAN_POINT('Ctrl Pts',(26.25,0.501266317583819,6.69979499726322));
#42958=CARTESIAN_POINT('Ctrl Pts',(26.5,0.172902956413169,6.86397667784855));
#42959=CARTESIAN_POINT('Ctrl Pts',(26.25,0.172902956413169,6.86397667784855));
#42960=CARTESIAN_POINT('Ctrl Pts',(26.5,-0.00634856473139531,7.15188948100021));
#42961=CARTESIAN_POINT('Ctrl Pts',(26.25,-0.00634856473139531,7.15188948100021));
#42962=CARTESIAN_POINT('',(26.5,0.501266317583819,6.69979499726322));
#42963=CARTESIAN_POINT('',(26.5,-0.00634856473139531,7.15188948100021));
#42964=CARTESIAN_POINT('Ctrl Pts',(26.5,0.501266317583819,6.69979499726322));
#42965=CARTESIAN_POINT('Ctrl Pts',(26.5,0.172902956413169,6.86397667784855));
#42966=CARTESIAN_POINT('Ctrl Pts',(26.5,-0.00634856473139531,7.15188948100021));
#42967=CARTESIAN_POINT('',(26.25,0.501266317583819,6.69979499726322));
#42968=CARTESIAN_POINT('',(26.5,0.501266317583819,6.69979499726322));
#42969=CARTESIAN_POINT('',(26.25,-0.00634856473139531,7.15188948100021));
#42970=CARTESIAN_POINT('Ctrl Pts',(26.25,0.501266317583819,6.69979499726322));
#42971=CARTESIAN_POINT('Ctrl Pts',(26.25,0.172902956413169,6.86397667784855));
#42972=CARTESIAN_POINT('Ctrl Pts',(26.25,-0.00634856473139531,7.15188948100021));
#42973=CARTESIAN_POINT('',(26.5,-0.00634856473139531,7.15188948100021));
#42974=CARTESIAN_POINT('Ctrl Pts',(26.5,1.13776779423563,6.56099416741769));
#42975=CARTESIAN_POINT('Ctrl Pts',(26.25,1.13776779423563,6.56099416741769));
#42976=CARTESIAN_POINT('Ctrl Pts',(26.5,0.804248894654697,6.54830370872778));
#42977=CARTESIAN_POINT('Ctrl Pts',(26.25,0.804248894654697,6.54830370872778));
#42978=CARTESIAN_POINT('Ctrl Pts',(26.5,0.501266317583819,6.69979499726322));
#42979=CARTESIAN_POINT('Ctrl Pts',(26.25,0.501266317583819,6.69979499726322));
#42980=CARTESIAN_POINT('',(26.5,1.13776779423563,6.56099416741769));
#42981=CARTESIAN_POINT('Ctrl Pts',(26.5,1.13776779423563,6.56099416741769));
#42982=CARTESIAN_POINT('Ctrl Pts',(26.5,0.804248894654697,6.54830370872778));
#42983=CARTESIAN_POINT('Ctrl Pts',(26.5,0.501266317583819,6.69979499726322));
#42984=CARTESIAN_POINT('',(26.25,1.13776779423563,6.56099416741769));
#42985=CARTESIAN_POINT('',(26.5,1.13776779423563,6.56099416741769));
#42986=CARTESIAN_POINT('Ctrl Pts',(26.25,1.13776779423563,6.56099416741769));
#42987=CARTESIAN_POINT('Ctrl Pts',(26.25,0.804248894654697,6.54830370872778));
#42988=CARTESIAN_POINT('Ctrl Pts',(26.25,0.501266317583819,6.69979499726322));
#42989=CARTESIAN_POINT('Ctrl Pts',(26.5,1.75364751708642,6.78148932944435));
#42990=CARTESIAN_POINT('Ctrl Pts',(26.25,1.75364751708642,6.78148932944435));
#42991=CARTESIAN_POINT('Ctrl Pts',(26.5,1.47128669381657,6.57368462610759));
#42992=CARTESIAN_POINT('Ctrl Pts',(26.25,1.47128669381657,6.57368462610759));
#42993=CARTESIAN_POINT('Ctrl Pts',(26.5,1.13776779423563,6.56099416741769));
#42994=CARTESIAN_POINT('Ctrl Pts',(26.25,1.13776779423563,6.56099416741769));
#42995=CARTESIAN_POINT('',(26.5,1.75364751708642,6.78148932944435));
#42996=CARTESIAN_POINT('Ctrl Pts',(26.5,1.75364751708642,6.78148932944435));
#42997=CARTESIAN_POINT('Ctrl Pts',(26.5,1.47128669381657,6.57368462610759));
#42998=CARTESIAN_POINT('Ctrl Pts',(26.5,1.13776779423563,6.56099416741769));
#42999=CARTESIAN_POINT('',(26.25,1.75364751708642,6.78148932944435));
#43000=CARTESIAN_POINT('',(26.5,1.75364751708642,6.78148932944435));
#43001=CARTESIAN_POINT('Ctrl Pts',(26.25,1.75364751708642,6.78148932944435));
#43002=CARTESIAN_POINT('Ctrl Pts',(26.25,1.47128669381657,6.57368462610759));
#43003=CARTESIAN_POINT('Ctrl Pts',(26.25,1.13776779423563,6.56099416741769));
#43004=CARTESIAN_POINT('Ctrl Pts',(26.5,2.21288027971144,7.34303824469154));
#43005=CARTESIAN_POINT('Ctrl Pts',(26.25,2.21288027971144,7.34303824469154));
#43006=CARTESIAN_POINT('Ctrl Pts',(26.5,2.03600820707623,6.98929409942112));
#43007=CARTESIAN_POINT('Ctrl Pts',(26.25,2.03600820707623,6.98929409942112));
#43008=CARTESIAN_POINT('Ctrl Pts',(26.5,1.75364751708642,6.78148932944435));
#43009=CARTESIAN_POINT('Ctrl Pts',(26.25,1.75364751708642,6.78148932944435));
#43010=CARTESIAN_POINT('',(26.5,2.21288027971144,7.34303824469154));
#43011=CARTESIAN_POINT('Ctrl Pts',(26.5,2.21288027971144,7.34303824469154));
#43012=CARTESIAN_POINT('Ctrl Pts',(26.5,2.03600820707623,6.98929409942112));
#43013=CARTESIAN_POINT('Ctrl Pts',(26.5,1.75364751708642,6.78148932944435));
#43014=CARTESIAN_POINT('',(26.25,2.21288027971144,7.34303824469154));
#43015=CARTESIAN_POINT('',(26.5,2.21288027971144,7.34303824469154));
#43016=CARTESIAN_POINT('Ctrl Pts',(26.25,2.21288027971144,7.34303824469154));
#43017=CARTESIAN_POINT('Ctrl Pts',(26.25,2.03600820707623,6.98929409942112));
#43018=CARTESIAN_POINT('Ctrl Pts',(26.25,1.75364751708642,6.78148932944435));
#43019=CARTESIAN_POINT('Ctrl Pts',(26.5,2.38935597751515,8.03506005328157));
#43020=CARTESIAN_POINT('Ctrl Pts',(26.25,2.38935597751515,8.03506005328157));
#43021=CARTESIAN_POINT('Ctrl Pts',(26.5,2.3873729038373,7.69202349294325));
#43022=CARTESIAN_POINT('Ctrl Pts',(26.25,2.3873729038373,7.69202349294325));
#43023=CARTESIAN_POINT('Ctrl Pts',(26.5,2.21288027971144,7.34303824469154));
#43024=CARTESIAN_POINT('Ctrl Pts',(26.25,2.21288027971144,7.34303824469154));
#43025=CARTESIAN_POINT('',(26.5,2.38935597751515,8.03506005328157));
#43026=CARTESIAN_POINT('Ctrl Pts',(26.5,2.38935597751515,8.03506005328157));
#43027=CARTESIAN_POINT('Ctrl Pts',(26.5,2.3873729038373,7.69202349294325));
#43028=CARTESIAN_POINT('Ctrl Pts',(26.5,2.21288027971144,7.34303824469154));
#43029=CARTESIAN_POINT('',(26.25,2.38935597751515,8.03506005328157));
#43030=CARTESIAN_POINT('',(26.5,2.38935597751515,8.03506005328157));
#43031=CARTESIAN_POINT('Ctrl Pts',(26.25,2.38935597751515,8.03506005328157));
#43032=CARTESIAN_POINT('Ctrl Pts',(26.25,2.3873729038373,7.69202349294325));
#43033=CARTESIAN_POINT('Ctrl Pts',(26.25,2.21288027971144,7.34303824469154));
#43034=CARTESIAN_POINT('Ctrl Pts',(26.5,2.20970768169897,8.66125071967288));
#43035=CARTESIAN_POINT('Ctrl Pts',(26.25,2.20970768169897,8.66125071967288));
#43036=CARTESIAN_POINT('Ctrl Pts',(26.5,2.39133858471287,8.3780966802599));
#43037=CARTESIAN_POINT('Ctrl Pts',(26.25,2.39133858471287,8.3780966802599));
#43038=CARTESIAN_POINT('Ctrl Pts',(26.5,2.38935597751515,8.03506005328157));
#43039=CARTESIAN_POINT('Ctrl Pts',(26.25,2.38935597751515,8.03506005328157));
#43040=CARTESIAN_POINT('',(26.5,2.20970768169897,8.66125071967288));
#43041=CARTESIAN_POINT('Ctrl Pts',(26.5,2.20970768169897,8.66125071967288));
#43042=CARTESIAN_POINT('Ctrl Pts',(26.5,2.39133858471287,8.3780966802599));
#43043=CARTESIAN_POINT('Ctrl Pts',(26.5,2.38935597751515,8.03506005328157));
#43044=CARTESIAN_POINT('',(26.25,2.20970768169897,8.66125071967288));
#43045=CARTESIAN_POINT('',(26.5,2.20970768169897,8.66125071967288));
#43046=CARTESIAN_POINT('Ctrl Pts',(26.25,2.20970768169897,8.66125071967288));
#43047=CARTESIAN_POINT('Ctrl Pts',(26.25,2.39133858471287,8.3780966802599));
#43048=CARTESIAN_POINT('Ctrl Pts',(26.25,2.38935597751515,8.03506005328157));
#43049=CARTESIAN_POINT('Ctrl Pts',(26.5,1.70605854689935,9.10541370837869));
#43050=CARTESIAN_POINT('Ctrl Pts',(26.25,1.70605854689935,9.10541370837869));
#43051=CARTESIAN_POINT('Ctrl Pts',(26.5,2.02807671204505,8.94440462580583));
#43052=CARTESIAN_POINT('Ctrl Pts',(26.25,2.02807671204505,8.94440462580583));
#43053=CARTESIAN_POINT('Ctrl Pts',(26.5,2.20970768169897,8.66125071967288));
#43054=CARTESIAN_POINT('Ctrl Pts',(26.25,2.20970768169897,8.66125071967288));
#43055=CARTESIAN_POINT('',(26.5,1.70605854689935,9.10541370837869));
#43056=CARTESIAN_POINT('Ctrl Pts',(26.5,1.70605854689935,9.10541370837869));
#43057=CARTESIAN_POINT('Ctrl Pts',(26.5,2.02807671204505,8.94440462580583));
#43058=CARTESIAN_POINT('Ctrl Pts',(26.5,2.20970768169897,8.66125071967288));
#43059=CARTESIAN_POINT('',(26.25,1.70605854689935,9.10541370837869));
#43060=CARTESIAN_POINT('',(26.5,1.70605854689935,9.10541370837869));
#43061=CARTESIAN_POINT('Ctrl Pts',(26.25,1.70605854689935,9.10541370837869));
#43062=CARTESIAN_POINT('Ctrl Pts',(26.25,2.02807671204505,8.94440462580583));
#43063=CARTESIAN_POINT('Ctrl Pts',(26.25,2.20970768169897,8.66125071967288));
#43064=CARTESIAN_POINT('Ctrl Pts',(26.5,0.739607410070647,9.17917651220862));
#43065=CARTESIAN_POINT('Ctrl Pts',(26.25,0.739607410070647,9.17917651220862));
#43066=CARTESIAN_POINT('Ctrl Pts',(26.5,1.21430658800647,9.35128968782512));
#43067=CARTESIAN_POINT('Ctrl Pts',(26.25,1.21430658800647,9.35128968782512));
#43068=CARTESIAN_POINT('Ctrl Pts',(26.5,1.70605854689935,9.10541370837869));
#43069=CARTESIAN_POINT('Ctrl Pts',(26.25,1.70605854689935,9.10541370837869));
#43070=CARTESIAN_POINT('',(26.5,0.739607410070647,9.17917651220862));
#43071=CARTESIAN_POINT('Ctrl Pts',(26.5,0.739607410070647,9.17917651220862));
#43072=CARTESIAN_POINT('Ctrl Pts',(26.5,1.21430658800647,9.35128968782512));
#43073=CARTESIAN_POINT('Ctrl Pts',(26.5,1.70605854689935,9.10541370837869));
#43074=CARTESIAN_POINT('',(26.25,0.739607410070647,9.17917651220862));
#43075=CARTESIAN_POINT('',(26.5,0.739607410070647,9.17917651220862));
#43076=CARTESIAN_POINT('Ctrl Pts',(26.25,0.739607410070647,9.17917651220862));
#43077=CARTESIAN_POINT('Ctrl Pts',(26.25,1.21430658800647,9.35128968782512));
#43078=CARTESIAN_POINT('Ctrl Pts',(26.25,1.70605854689935,9.10541370837869));
#43079=CARTESIAN_POINT('Ctrl Pts',(26.5,-0.0245909866431014,8.4280650239863));
#43080=CARTESIAN_POINT('Ctrl Pts',(26.25,-0.0245909866431014,8.4280650239863));
#43081=CARTESIAN_POINT('Ctrl Pts',(26.5,0.26490818215481,9.00706336158212));
#43082=CARTESIAN_POINT('Ctrl Pts',(26.25,0.26490818215481,9.00706336158212));
#43083=CARTESIAN_POINT('Ctrl Pts',(26.5,0.739607410070647,9.17917651220862));
#43084=CARTESIAN_POINT('Ctrl Pts',(26.25,0.739607410070647,9.17917651220862));
#43085=CARTESIAN_POINT('',(26.5,-0.0245909866431014,8.4280650239863));
#43086=CARTESIAN_POINT('Ctrl Pts',(26.5,-0.0245909866431014,8.4280650239863));
#43087=CARTESIAN_POINT('Ctrl Pts',(26.5,0.26490818215481,9.00706336158212));
#43088=CARTESIAN_POINT('Ctrl Pts',(26.5,0.739607410070647,9.17917651220862));
#43089=CARTESIAN_POINT('',(26.25,-0.0245909866431014,8.4280650239863));
#43090=CARTESIAN_POINT('',(26.5,-0.0245909866431014,8.4280650239863));
#43091=CARTESIAN_POINT('Ctrl Pts',(26.25,-0.0245909866431014,8.4280650239863));
#43092=CARTESIAN_POINT('Ctrl Pts',(26.25,0.26490818215481,9.00706336158212));
#43093=CARTESIAN_POINT('Ctrl Pts',(26.25,0.739607410070647,9.17917651220862));
#43094=CARTESIAN_POINT('Ctrl Pts',(26.5,-0.181634271720352,7.78085620397245));
#43095=CARTESIAN_POINT('Ctrl Pts',(26.25,-0.181634271720352,7.78085620397245));
#43096=CARTESIAN_POINT('Ctrl Pts',(26.5,-0.177668574184776,8.12190984890295));
#43097=CARTESIAN_POINT('Ctrl Pts',(26.25,-0.177668574184776,8.12190984890295));
#43098=CARTESIAN_POINT('Ctrl Pts',(26.5,-0.0245909866431014,8.4280650239863));
#43099=CARTESIAN_POINT('Ctrl Pts',(26.25,-0.0245909866431014,8.4280650239863));
#43100=CARTESIAN_POINT('',(26.5,-0.181634271720352,7.78085620397245));
#43101=CARTESIAN_POINT('Ctrl Pts',(26.5,-0.181634271720352,7.78085620397245));
#43102=CARTESIAN_POINT('Ctrl Pts',(26.5,-0.177668574184776,8.12190984890295));
#43103=CARTESIAN_POINT('Ctrl Pts',(26.5,-0.0245909866431014,8.4280650239863));
#43104=CARTESIAN_POINT('',(26.25,-0.181634271720352,7.78085620397245));
#43105=CARTESIAN_POINT('',(26.5,-0.181634271720352,7.78085620397245));
#43106=CARTESIAN_POINT('Ctrl Pts',(26.25,-0.181634271720352,7.78085620397245));
#43107=CARTESIAN_POINT('Ctrl Pts',(26.25,-0.177668574184776,8.12190984890295));
#43108=CARTESIAN_POINT('Ctrl Pts',(26.25,-0.0245909866431014,8.4280650239863));
#43109=CARTESIAN_POINT('Ctrl Pts',(26.5,-0.00634856473139531,7.15188948100021));
#43110=CARTESIAN_POINT('Ctrl Pts',(26.25,-0.00634856473139531,7.15188948100021));
#43111=CARTESIAN_POINT('Ctrl Pts',(26.5,-0.18560008587596,7.43980228415186));
#43112=CARTESIAN_POINT('Ctrl Pts',(26.25,-0.18560008587596,7.43980228415186));
#43113=CARTESIAN_POINT('Ctrl Pts',(26.5,-0.181634271720352,7.78085620397245));
#43114=CARTESIAN_POINT('Ctrl Pts',(26.25,-0.181634271720352,7.78085620397245));
#43115=CARTESIAN_POINT('Ctrl Pts',(26.5,-0.00634856473139531,7.15188948100021));
#43116=CARTESIAN_POINT('Ctrl Pts',(26.5,-0.18560008587596,7.43980228415186));
#43117=CARTESIAN_POINT('Ctrl Pts',(26.5,-0.181634271720352,7.78085620397245));
#43118=CARTESIAN_POINT('Ctrl Pts',(26.25,-0.00634856473139531,7.15188948100021));
#43119=CARTESIAN_POINT('Ctrl Pts',(26.25,-0.18560008587596,7.43980228415186));
#43120=CARTESIAN_POINT('Ctrl Pts',(26.25,-0.181634271720352,7.78085620397245));
#43121=CARTESIAN_POINT('Origin',(26.25,1.10286924941845,7.94979669827645));
#43122=CARTESIAN_POINT('Origin',(26.5,3.97287629488924,6.33415360944603));
#43123=CARTESIAN_POINT('',(26.5,3.97287629488924,6.33415360944603));
#43124=CARTESIAN_POINT('',(26.5,2.88150424459951,6.8798396345909));
#43125=CARTESIAN_POINT('',(26.5,3.65055649882275,6.49531350747928));
#43126=CARTESIAN_POINT('',(26.25,3.97287629488924,6.33415360944603));
#43127=CARTESIAN_POINT('',(26.5,3.97287629488924,6.33415360944603));
#43128=CARTESIAN_POINT('',(26.25,2.88150424459951,6.8798396345909));
#43129=CARTESIAN_POINT('',(26.25,3.97287629488924,6.33415360944603));
#43130=CARTESIAN_POINT('',(26.5,2.88150424459951,6.8798396345909));
#43131=CARTESIAN_POINT('Origin',(26.5,4.11009095900857,6.60858293768471));
#43132=CARTESIAN_POINT('',(26.5,4.11009095900857,6.60858293768471));
#43133=CARTESIAN_POINT('',(26.5,2.37736527557078,3.14313157080911));
#43134=CARTESIAN_POINT('',(26.25,4.11009095900857,6.60858293768471));
#43135=CARTESIAN_POINT('',(26.5,4.11009095900857,6.60858293768471));
#43136=CARTESIAN_POINT('',(26.25,4.11009095900857,6.60858293768471));
#43137=CARTESIAN_POINT('Origin',(26.5,3.01871890871885,7.15426896282957));
#43138=CARTESIAN_POINT('',(26.5,3.01871890871885,7.15426896282957));
#43139=CARTESIAN_POINT('',(26.5,3.24208513779722,7.04258584829038));
#43140=CARTESIAN_POINT('',(26.25,3.01871890871885,7.15426896282957));
#43141=CARTESIAN_POINT('',(26.5,3.01871890871885,7.15426896282957));
#43142=CARTESIAN_POINT('',(26.25,3.01871890871885,7.15426896282957));
#43143=CARTESIAN_POINT('Origin',(26.5,3.37880818337419,7.87444751214026));
#43144=CARTESIAN_POINT('',(26.5,3.37880818337419,7.87444751214026));
#43145=CARTESIAN_POINT('',(26.5,1.46603786260872,4.04890687060932));
#43146=CARTESIAN_POINT('',(26.25,3.37880818337419,7.87444751214026));
#43147=CARTESIAN_POINT('',(26.5,3.37880818337419,7.87444751214026));
#43148=CARTESIAN_POINT('',(26.25,3.37880818337419,7.87444751214026));
#43149=CARTESIAN_POINT('Origin',(26.5,4.63991396077107,7.24389462344182));
#43150=CARTESIAN_POINT('',(26.5,4.63991396077107,7.24389462344182));
#43151=CARTESIAN_POINT('',(26.5,4.23272730115101,7.44748795325186));
#43152=CARTESIAN_POINT('',(26.25,4.63991396077107,7.24389462344182));
#43153=CARTESIAN_POINT('',(26.5,4.63991396077107,7.24389462344182));
#43154=CARTESIAN_POINT('',(26.25,4.63991396077107,7.24389462344182));
#43155=CARTESIAN_POINT('Origin',(26.5,4.7771286248904,7.5183239516805));
#43156=CARTESIAN_POINT('',(26.5,4.7771286248904,7.5183239516805));
#43157=CARTESIAN_POINT('',(26.5,2.79575097206527,3.55556864603021));
#43158=CARTESIAN_POINT('',(26.25,4.7771286248904,7.5183239516805));
#43159=CARTESIAN_POINT('',(26.5,4.7771286248904,7.5183239516805));
#43160=CARTESIAN_POINT('',(26.25,4.7771286248904,7.5183239516805));
#43161=CARTESIAN_POINT('Origin',(26.5,3.20828129010392,8.30274761907374));
#43162=CARTESIAN_POINT('',(26.5,3.20828129010392,8.30274761907374));
#43163=CARTESIAN_POINT('',(26.5,3.5855182978771,8.11412911518715));
#43164=CARTESIAN_POINT('',(26.25,3.20828129010392,8.30274761907374));
#43165=CARTESIAN_POINT('',(26.5,3.20828129010392,8.30274761907374));
#43166=CARTESIAN_POINT('',(26.25,3.20828129010392,8.30274761907374));
#43167=CARTESIAN_POINT('Origin',(26.5,2.04552598445364,5.97723700777318));
#43168=CARTESIAN_POINT('',(26.5,2.04552598445364,5.97723700777318));
#43169=CARTESIAN_POINT('',(26.5,0.64552598445364,3.17723700777318));
#43170=CARTESIAN_POINT('',(26.25,2.04552598445364,5.97723700777318));
#43171=CARTESIAN_POINT('',(26.5,2.04552598445364,5.97723700777318));
#43172=CARTESIAN_POINT('',(26.25,2.04552598445364,5.97723700777318));
#43173=CARTESIAN_POINT('Origin',(26.5,2.35326754184325,5.82336622907838));
#43174=CARTESIAN_POINT('',(26.5,2.35326754184325,5.82336622907838));
#43175=CARTESIAN_POINT('',(26.5,2.57663377092163,5.71168311453919));
#43176=CARTESIAN_POINT('',(26.25,2.35326754184325,5.82336622907838));
#43177=CARTESIAN_POINT('',(26.5,2.35326754184325,5.82336622907838));
#43178=CARTESIAN_POINT('',(26.25,2.35326754184325,5.82336622907838));
#43179=CARTESIAN_POINT('Origin',(26.5,2.88150424459951,6.8798396345909));
#43180=CARTESIAN_POINT('',(26.5,1.21738589322138,3.55160293183464));
#43181=CARTESIAN_POINT('',(26.25,2.88150424459951,6.8798396345909));
#43182=CARTESIAN_POINT('Origin',(26.25,3.41132730467202,7.06305692407606));
#43183=CARTESIAN_POINT('Origin',(26.5,5.95733328624929,5.34192511376601));
#43184=CARTESIAN_POINT('',(26.5,5.95733328624929,5.34192511376601));
#43185=CARTESIAN_POINT('',(26.5,4.86596123595957,5.88761113891087));
#43186=CARTESIAN_POINT('',(26.5,4.64278499450278,5.99919925963926));
#43187=CARTESIAN_POINT('',(26.25,5.95733328624929,5.34192511376601));
#43188=CARTESIAN_POINT('',(26.5,5.95733328624929,5.34192511376601));
#43189=CARTESIAN_POINT('',(26.25,4.86596123595957,5.88761113891087));
#43190=CARTESIAN_POINT('',(26.25,5.95733328624929,5.34192511376601));
#43191=CARTESIAN_POINT('',(26.5,4.86596123595957,5.88761113891087));
#43192=CARTESIAN_POINT('Origin',(26.5,6.09454795036863,5.61635444200468));
#43193=CARTESIAN_POINT('',(26.5,6.09454795036863,5.61635444200468));
#43194=CARTESIAN_POINT('',(26.5,4.36182226693084,2.15090307512908));
#43195=CARTESIAN_POINT('',(26.25,6.09454795036863,5.61635444200468));
#43196=CARTESIAN_POINT('',(26.5,6.09454795036863,5.61635444200468));
#43197=CARTESIAN_POINT('',(26.25,6.09454795036863,5.61635444200468));
#43198=CARTESIAN_POINT('Origin',(26.5,5.0031759000789,6.16204046714954));
#43199=CARTESIAN_POINT('',(26.5,5.0031759000789,6.16204046714954));
#43200=CARTESIAN_POINT('',(26.5,4.23431363347725,6.54647160045037));
#43201=CARTESIAN_POINT('',(26.25,5.0031759000789,6.16204046714954));
#43202=CARTESIAN_POINT('',(26.5,5.0031759000789,6.16204046714954));
#43203=CARTESIAN_POINT('',(26.25,5.0031759000789,6.16204046714954));
#43204=CARTESIAN_POINT('Origin',(26.5,5.36326517473425,6.88221901646023));
#43205=CARTESIAN_POINT('',(26.5,5.36326517473425,6.88221901646023));
#43206=CARTESIAN_POINT('',(26.5,3.45049485396878,3.05667837492929));
#43207=CARTESIAN_POINT('',(26.25,5.36326517473425,6.88221901646023));
#43208=CARTESIAN_POINT('',(26.5,5.36326517473425,6.88221901646023));
#43209=CARTESIAN_POINT('',(26.25,5.36326517473425,6.88221901646023));
#43210=CARTESIAN_POINT('Origin',(26.5,6.62437095213113,6.25166612776179));
#43211=CARTESIAN_POINT('',(26.5,6.62437095213113,6.25166612776179));
#43212=CARTESIAN_POINT('',(26.5,5.22495579683104,6.95137370541184));
#43213=CARTESIAN_POINT('',(26.25,6.62437095213113,6.25166612776179));
#43214=CARTESIAN_POINT('',(26.5,6.62437095213113,6.25166612776179));
#43215=CARTESIAN_POINT('',(26.25,6.62437095213113,6.25166612776179));
#43216=CARTESIAN_POINT('Origin',(26.5,6.76158561625046,6.52609545600047));
#43217=CARTESIAN_POINT('',(26.5,6.76158561625046,6.52609545600047));
#43218=CARTESIAN_POINT('',(26.5,4.78020796342532,2.56334015035019));
#43219=CARTESIAN_POINT('',(26.25,6.76158561625046,6.52609545600047));
#43220=CARTESIAN_POINT('',(26.5,6.76158561625046,6.52609545600047));
#43221=CARTESIAN_POINT('',(26.25,6.76158561625046,6.52609545600047));
#43222=CARTESIAN_POINT('Origin',(26.5,5.19273828146398,7.31051912339371));
#43223=CARTESIAN_POINT('',(26.5,5.19273828146398,7.31051912339371));
#43224=CARTESIAN_POINT('',(26.5,4.57774679355713,7.61801486734714));
#43225=CARTESIAN_POINT('',(26.25,5.19273828146398,7.31051912339371));
#43226=CARTESIAN_POINT('',(26.5,5.19273828146398,7.31051912339371));
#43227=CARTESIAN_POINT('',(26.25,5.19273828146398,7.31051912339371));
#43228=CARTESIAN_POINT('Origin',(26.5,4.0299829758137,4.98500851209315));
#43229=CARTESIAN_POINT('',(26.5,4.0299829758137,4.98500851209315));
#43230=CARTESIAN_POINT('',(26.5,2.6299829758137,2.18500851209315));
#43231=CARTESIAN_POINT('',(26.25,4.0299829758137,4.98500851209315));
#43232=CARTESIAN_POINT('',(26.5,4.0299829758137,4.98500851209315));
#43233=CARTESIAN_POINT('',(26.25,4.0299829758137,4.98500851209315));
#43234=CARTESIAN_POINT('Origin',(26.5,4.33772453320331,4.83113773339835));
#43235=CARTESIAN_POINT('',(26.5,4.33772453320331,4.83113773339835));
#43236=CARTESIAN_POINT('',(26.5,3.56886226660165,5.21556886669917));
#43237=CARTESIAN_POINT('',(26.25,4.33772453320331,4.83113773339835));
#43238=CARTESIAN_POINT('',(26.5,4.33772453320331,4.83113773339835));
#43239=CARTESIAN_POINT('',(26.25,4.33772453320331,4.83113773339835));
#43240=CARTESIAN_POINT('Origin',(26.5,4.86596123595957,5.88761113891087));
#43241=CARTESIAN_POINT('',(26.5,3.20184288458144,2.55937443615461));
#43242=CARTESIAN_POINT('',(26.25,4.86596123595957,5.88761113891087));
#43243=CARTESIAN_POINT('Origin',(26.25,5.39578429603208,6.07082842839603));
#43244=CARTESIAN_POINT('Origin',(26.2,3.6,0.));
#43245=CARTESIAN_POINT('',(26.2,-3.6,-4.40872847693047E-16));
#43246=CARTESIAN_POINT('Origin',(26.2,0.,0.));
#43247=CARTESIAN_POINT('',(26.2,-3.,-3.67394039744206E-16));
#43248=CARTESIAN_POINT('Origin',(26.2,0.,0.));
#43249=CARTESIAN_POINT('Origin',(26.4,0.,0.));
#43250=CARTESIAN_POINT('',(26.5,-3.6,4.40872847693047E-16));
#43251=CARTESIAN_POINT('',(26.4,-3.6,-4.40872847693047E-16));
#43252=CARTESIAN_POINT('Origin',(26.5,0.,0.));
#43253=CARTESIAN_POINT('Origin',(26.4,0.,0.));
#43254=CARTESIAN_POINT('',(26.5,-3.,-3.67394039744206E-16));
#43255=CARTESIAN_POINT('',(26.4,-3.,-3.67394039744206E-16));
#43256=CARTESIAN_POINT('Origin',(26.5,0.,0.));
#43257=CARTESIAN_POINT('Origin',(26.5,0.,0.));
#43258=CARTESIAN_POINT('Origin',(17.3,12.8479908659033,-2.32198852487824));
#43259=CARTESIAN_POINT('',(25.7,12.7818649395498,-2.37148237756648));
#43260=CARTESIAN_POINT('',(17.3,12.7818649395498,-2.37148237756648));
#43261=CARTESIAN_POINT('',(21.5,12.7818649395498,-2.37148237756648));
#43262=CARTESIAN_POINT('',(25.7,12.4224745293193,-2.64047847338555));
#43263=CARTESIAN_POINT('',(25.7,12.8479908659033,-2.32198852487824));
#43264=CARTESIAN_POINT('',(17.3,12.4224745293193,-2.64047847338555));
#43265=CARTESIAN_POINT('',(17.3,12.4224745293193,-2.64047847338555));
#43266=CARTESIAN_POINT('',(17.3,12.8479908659033,-2.32198852487824));
#43267=CARTESIAN_POINT('Origin',(17.3,12.5936503594477,-2.67686301927866));
#43268=CARTESIAN_POINT('',(17.3,12.6413834370917,-3.03239588385542));
#43269=CARTESIAN_POINT('Origin',(17.3,0.,0.));
#43270=CARTESIAN_POINT('',(17.3,12.4224745293193,-2.64047847338555));
#43271=CARTESIAN_POINT('Origin',(17.3,12.4224745293193,-2.64047847338555));
#43272=CARTESIAN_POINT('',(25.7,12.6413834370917,-3.03239588385542));
#43273=CARTESIAN_POINT('',(21.5,12.6413834370917,-3.03239588385542));
#43274=CARTESIAN_POINT('',(25.7,12.4224745293193,-2.64047847338555));
#43275=CARTESIAN_POINT('Origin',(25.7,12.5936503594477,-2.67686301927866));
#43276=CARTESIAN_POINT('Origin',(25.7,0.,0.));
#43277=CARTESIAN_POINT('Origin',(17.3,12.0844628794663,-4.94249500908216));
#43278=CARTESIAN_POINT('',(25.7,12.0094916126598,-4.97715894918518));
#43279=CARTESIAN_POINT('',(17.3,12.0094916126598,-4.97715894918518));
#43280=CARTESIAN_POINT('',(21.5,12.0094916126598,-4.97715894918518));
#43281=CARTESIAN_POINT('',(25.7,11.602027312061,-5.16555536706267));
#43282=CARTESIAN_POINT('',(25.7,12.0844628794663,-4.94249500908216));
#43283=CARTESIAN_POINT('',(17.3,11.602027312061,-5.16555536706267));
#43284=CARTESIAN_POINT('',(17.3,11.602027312061,-5.16555536706267));
#43285=CARTESIAN_POINT('',(17.3,12.0844628794663,-4.94249500908216));
#43286=CARTESIAN_POINT('Origin',(17.3,11.7618977671485,-5.23673427960094));
#43287=CARTESIAN_POINT('',(17.3,11.7346683235061,-5.59442216294961));
#43288=CARTESIAN_POINT('Origin',(17.3,0.,0.));
#43289=CARTESIAN_POINT('',(17.3,11.602027312061,-5.16555536706267));
#43290=CARTESIAN_POINT('Origin',(17.3,11.602027312061,-5.16555536706267));
#43291=CARTESIAN_POINT('',(25.7,11.7346683235061,-5.59442216294961));
#43292=CARTESIAN_POINT('',(21.5,11.7346683235061,-5.59442216294961));
#43293=CARTESIAN_POINT('',(25.7,11.602027312061,-5.16555536706267));
#43294=CARTESIAN_POINT('Origin',(25.7,11.7618977671485,-5.23673427960094));
#43295=CARTESIAN_POINT('Origin',(25.7,0.,0.));
#43296=CARTESIAN_POINT('Origin',(17.3,10.7927858775101,-7.3469907446668));
#43297=CARTESIAN_POINT('',(25.7,10.7122458743621,-7.36530979166607));
#43298=CARTESIAN_POINT('',(17.3,10.7122458743621,-7.36530979166607));
#43299=CARTESIAN_POINT('',(21.5,10.7122458743621,-7.36530979166607));
#43300=CARTESIAN_POINT('',(25.7,10.2745158285618,-7.46487270411441));
#43301=CARTESIAN_POINT('',(25.7,10.7927858775101,-7.3469907446668));
#43302=CARTESIAN_POINT('',(17.3,10.2745158285618,-7.46487270411441));
#43303=CARTESIAN_POINT('',(17.3,10.2745158285618,-7.46487270411441));
#43304=CARTESIAN_POINT('',(17.3,10.7927858775101,-7.3469907446668));
#43305=CARTESIAN_POINT('Origin',(17.3,10.4160938025774,-7.5677351232656));
#43306=CARTESIAN_POINT('',(17.3,10.3150918949973,-7.91194534850694));
#43307=CARTESIAN_POINT('Origin',(17.3,0.,0.));
#43308=CARTESIAN_POINT('',(17.3,10.2745158285618,-7.46487270411441));
#43309=CARTESIAN_POINT('Origin',(17.3,10.2745158285618,-7.46487270411441));
#43310=CARTESIAN_POINT('',(25.7,10.3150918949973,-7.91194534850694));
#43311=CARTESIAN_POINT('',(21.5,10.3150918949973,-7.91194534850694));
#43312=CARTESIAN_POINT('',(25.7,10.2745158285618,-7.46487270411441));
#43313=CARTESIAN_POINT('Origin',(25.7,10.4160938025774,-7.5677351232656));
#43314=CARTESIAN_POINT('Origin',(25.7,0.,0.));
#43315=CARTESIAN_POINT('Origin',(17.3,9.02941234317406,-9.43038772993646));
#43316=CARTESIAN_POINT('',(25.7,8.94682358829601,-9.43156125357357));
#43317=CARTESIAN_POINT('',(17.3,8.94682358829601,-9.43156125357357));
#43318=CARTESIAN_POINT('',(21.5,8.94682358829601,-9.43156125357357));
#43319=CARTESIAN_POINT('',(25.7,8.4979587007575,-9.43793928356291));
#43320=CARTESIAN_POINT('',(25.7,9.02941234317406,-9.43038772993646));
#43321=CARTESIAN_POINT('',(17.3,8.4979587007575,-9.43793928356291));
#43322=CARTESIAN_POINT('',(17.3,8.4979587007575,-9.43793928356291));
#43323=CARTESIAN_POINT('',(17.3,9.02941234317406,-9.43038772993646));
#43324=CARTESIAN_POINT('Origin',(17.3,8.6150565568703,-9.56798962802146));
#43325=CARTESIAN_POINT('',(17.3,8.44469645337457,-9.88367855660852));
#43326=CARTESIAN_POINT('Origin',(17.3,0.,0.));
#43327=CARTESIAN_POINT('',(17.3,8.4979587007575,-9.43793928356291));
#43328=CARTESIAN_POINT('Origin',(17.3,8.4979587007575,-9.43793928356291));
#43329=CARTESIAN_POINT('',(25.7,8.44469645337457,-9.88367855660852));
#43330=CARTESIAN_POINT('',(21.5,8.44469645337457,-9.88367855660852));
#43331=CARTESIAN_POINT('',(25.7,8.4979587007575,-9.43793928356291));
#43332=CARTESIAN_POINT('Origin',(25.7,8.6150565568703,-9.56798962802146));
#43333=CARTESIAN_POINT('Origin',(25.7,0.,0.));
#43334=CARTESIAN_POINT('Origin',(17.3,6.87141016151377,-11.1016315193869));
#43335=CARTESIAN_POINT('',(25.7,6.79038217979861,-11.0856082310477));
#43336=CARTESIAN_POINT('',(17.3,6.79038217979861,-11.0856082310477));
#43337=CARTESIAN_POINT('',(21.5,6.79038217979861,-11.0856082310477));
#43338=CARTESIAN_POINT('',(25.7,6.34999999999999,-10.9985226280624));
#43339=CARTESIAN_POINT('',(25.7,6.87141016151377,-11.1016315193869));
#43340=CARTESIAN_POINT('',(17.3,6.34999999999999,-10.9985226280624));
#43341=CARTESIAN_POINT('',(17.3,6.34999999999999,-10.9985226280624));
#43342=CARTESIAN_POINT('',(17.3,6.87141016151377,-11.1016315193869));
#43343=CARTESIAN_POINT('Origin',(17.3,6.43749999999999,-11.1500770737247));
#43344=CARTESIAN_POINT('',(17.3,6.2052272545899,-11.4234475846346));
#43345=CARTESIAN_POINT('Origin',(17.3,0.,0.));
#43346=CARTESIAN_POINT('',(17.3,6.34999999999999,-10.9985226280624));
#43347=CARTESIAN_POINT('Origin',(17.3,6.34999999999999,-10.9985226280624));
#43348=CARTESIAN_POINT('',(25.7,6.2052272545899,-11.4234475846346));
#43349=CARTESIAN_POINT('',(21.5,6.2052272545899,-11.4234475846346));
#43350=CARTESIAN_POINT('',(25.7,6.34999999999999,-10.9985226280624));
#43351=CARTESIAN_POINT('Origin',(25.7,6.43749999999999,-11.1500770737247));
#43352=CARTESIAN_POINT('Origin',(25.7,0.,0.));
#43353=CARTESIAN_POINT('Origin',(17.3,4.41309438311112,-12.2876807399018));
#43354=CARTESIAN_POINT('',(25.7,4.3371684861752,-12.255160934175));
#43355=CARTESIAN_POINT('',(17.3,4.3371684861752,-12.255160934175));
#43356=CARTESIAN_POINT('',(21.5,4.3371684861752,-12.255160934175));
#43357=CARTESIAN_POINT('',(25.7,3.92451582856183,-12.0784177569485));
#43358=CARTESIAN_POINT('',(25.7,4.41309438311112,-12.2876807399018));
#43359=CARTESIAN_POINT('',(17.3,3.92451582856183,-12.0784177569485));
#43360=CARTESIAN_POINT('',(17.3,3.92451582856183,-12.0784177569485));
#43361=CARTESIAN_POINT('',(17.3,4.41309438311112,-12.2876807399018));
#43362=CARTESIAN_POINT('Origin',(17.3,3.97859380257745,-12.2448526473001));
#43363=CARTESIAN_POINT('',(17.3,3.6945598487957,-12.463957137429));
#43364=CARTESIAN_POINT('Origin',(17.3,0.,0.));
#43365=CARTESIAN_POINT('',(17.3,3.92451582856183,-12.0784177569485));
#43366=CARTESIAN_POINT('Origin',(17.3,3.92451582856183,-12.0784177569485));
#43367=CARTESIAN_POINT('',(25.7,3.6945598487957,-12.463957137429));
#43368=CARTESIAN_POINT('',(21.5,3.6945598487957,-12.463957137429));
#43369=CARTESIAN_POINT('',(25.7,3.92451582856183,-12.0784177569485));
#43370=CARTESIAN_POINT('Origin',(25.7,3.97859380257745,-12.2448526473001));
#43371=CARTESIAN_POINT('Origin',(25.7,0.,0.));
#43372=CARTESIAN_POINT('Origin',(17.3,1.76190520379018,-12.9366993492489));
#43373=CARTESIAN_POINT('',(25.7,1.69439971766246,-12.8891042976921));
#43374=CARTESIAN_POINT('',(17.3,1.69439971766246,-12.8891042976921));
#43375=CARTESIAN_POINT('',(21.5,1.69439971766246,-12.8891042976921));
#43376=CARTESIAN_POINT('',(25.7,1.32751148349919,-12.6304280711771));
#43377=CARTESIAN_POINT('',(25.7,1.76190520379018,-12.9366993492489));
#43378=CARTESIAN_POINT('',(17.3,1.32751148349919,-12.6304280711771));
#43379=CARTESIAN_POINT('',(17.3,1.32751148349919,-12.6304280711771));
#43380=CARTESIAN_POINT('',(17.3,1.76190520379018,-12.9366993492489));
#43381=CARTESIAN_POINT('Origin',(17.3,1.34580396457103,-12.8044694028665));
#43382=CARTESIAN_POINT('',(17.3,1.02242244914403,-12.9597319546157));
#43383=CARTESIAN_POINT('Origin',(17.3,0.,0.));
#43384=CARTESIAN_POINT('',(17.3,1.32751148349919,-12.6304280711771));
#43385=CARTESIAN_POINT('Origin',(17.3,1.32751148349919,-12.6304280711771));
#43386=CARTESIAN_POINT('',(25.7,1.02242244914403,-12.9597319546157));
#43387=CARTESIAN_POINT('',(21.5,1.02242244914403,-12.9597319546157));
#43388=CARTESIAN_POINT('',(25.7,1.32751148349919,-12.6304280711771));
#43389=CARTESIAN_POINT('Origin',(25.7,1.34580396457103,-12.8044694028665));
#43390=CARTESIAN_POINT('Origin',(25.7,0.,0.));
#43391=CARTESIAN_POINT('Origin',(17.3,-0.966287687495578,-13.020322119863));
#43392=CARTESIAN_POINT('',(25.7,-1.02242244914404,-12.9597319546157));
#43393=CARTESIAN_POINT('',(17.3,-1.02242244914404,-12.9597319546157));
#43394=CARTESIAN_POINT('',(21.5,-1.02242244914404,-12.9597319546157));
#43395=CARTESIAN_POINT('',(25.7,-1.32751148349921,-12.6304280711771));
#43396=CARTESIAN_POINT('',(25.7,-0.966287687495578,-13.020322119863));
#43397=CARTESIAN_POINT('',(17.3,-1.32751148349921,-12.6304280711771));
#43398=CARTESIAN_POINT('',(17.3,-1.32751148349921,-12.6304280711771));
#43399=CARTESIAN_POINT('',(17.3,-0.966287687495578,-13.020322119863));
#43400=CARTESIAN_POINT('Origin',(17.3,-1.34580396457105,-12.8044694028665));
#43401=CARTESIAN_POINT('',(17.3,-1.69439971766248,-12.8891042976921));
#43402=CARTESIAN_POINT('Origin',(17.3,0.,0.));
#43403=CARTESIAN_POINT('',(17.3,-1.32751148349921,-12.6304280711771));
#43404=CARTESIAN_POINT('Origin',(17.3,-1.32751148349921,-12.6304280711771));
#43405=CARTESIAN_POINT('',(25.7,-1.69439971766248,-12.8891042976921));
#43406=CARTESIAN_POINT('',(21.5,-1.69439971766248,-12.8891042976921));
#43407=CARTESIAN_POINT('',(25.7,-1.32751148349921,-12.6304280711771));
#43408=CARTESIAN_POINT('Origin',(25.7,-1.34580396457105,-12.8044694028665));
#43409=CARTESIAN_POINT('Origin',(25.7,0.,0.));
#43410=CARTESIAN_POINT('Origin',(17.3,-3.65224917007501,-12.5348943354017));
#43411=CARTESIAN_POINT('',(25.7,-3.69455984879571,-12.463957137429));
#43412=CARTESIAN_POINT('',(17.3,-3.69455984879571,-12.463957137429));
#43413=CARTESIAN_POINT('',(21.5,-3.69455984879571,-12.463957137429));
#43414=CARTESIAN_POINT('',(25.7,-3.92451582856183,-12.0784177569485));
#43415=CARTESIAN_POINT('',(25.7,-3.65224917007501,-12.5348943354017));
#43416=CARTESIAN_POINT('',(17.3,-3.92451582856183,-12.0784177569485));
#43417=CARTESIAN_POINT('',(17.3,-3.92451582856183,-12.0784177569485));
#43418=CARTESIAN_POINT('',(17.3,-3.65224917007501,-12.5348943354017));
#43419=CARTESIAN_POINT('Origin',(17.3,-3.97859380257745,-12.2448526473001));
#43420=CARTESIAN_POINT('',(17.3,-4.3371684861752,-12.255160934175));
#43421=CARTESIAN_POINT('Origin',(17.3,0.,0.));
#43422=CARTESIAN_POINT('',(17.3,-3.92451582856183,-12.0784177569485));
#43423=CARTESIAN_POINT('Origin',(17.3,-3.92451582856183,-12.0784177569485));
#43424=CARTESIAN_POINT('',(25.7,-4.3371684861752,-12.255160934175));
#43425=CARTESIAN_POINT('',(21.5,-4.3371684861752,-12.255160934175));
#43426=CARTESIAN_POINT('',(25.7,-3.92451582856183,-12.0784177569485));
#43427=CARTESIAN_POINT('Origin',(25.7,-3.97859380257745,-12.2448526473001));
#43428=CARTESIAN_POINT('Origin',(25.7,0.,0.));
#43429=CARTESIAN_POINT('Origin',(17.3,-6.17858983848623,-11.5016315193869));
#43430=CARTESIAN_POINT('',(25.7,-6.20522725458991,-11.4234475846346));
#43431=CARTESIAN_POINT('',(17.3,-6.20522725458991,-11.4234475846346));
#43432=CARTESIAN_POINT('',(21.5,-6.20522725458991,-11.4234475846346));
#43433=CARTESIAN_POINT('',(25.7,-6.35000000000001,-10.9985226280624));
#43434=CARTESIAN_POINT('',(25.7,-6.17858983848623,-11.5016315193869));
#43435=CARTESIAN_POINT('',(17.3,-6.35000000000001,-10.9985226280624));
#43436=CARTESIAN_POINT('',(17.3,-6.35000000000001,-10.9985226280624));
#43437=CARTESIAN_POINT('',(17.3,-6.17858983848623,-11.5016315193869));
#43438=CARTESIAN_POINT('Origin',(17.3,-6.43750000000001,-11.1500770737246));
#43439=CARTESIAN_POINT('',(17.3,-6.79038217979862,-11.0856082310477));
#43440=CARTESIAN_POINT('Origin',(17.3,0.,0.));
#43441=CARTESIAN_POINT('',(17.3,-6.35000000000001,-10.9985226280624));
#43442=CARTESIAN_POINT('Origin',(17.3,-6.35000000000001,-10.9985226280624));
#43443=CARTESIAN_POINT('',(25.7,-6.79038217979862,-11.0856082310477));
#43444=CARTESIAN_POINT('',(21.5,-6.79038217979862,-11.0856082310477));
#43445=CARTESIAN_POINT('',(25.7,-6.35000000000001,-10.9985226280624));
#43446=CARTESIAN_POINT('Origin',(25.7,-6.43750000000001,-11.1500770737246));
#43447=CARTESIAN_POINT('Origin',(25.7,0.,0.));
#43448=CARTESIAN_POINT('Origin',(17.3,-8.43489648279215,-9.96569221502354));
#43449=CARTESIAN_POINT('',(25.7,-8.44469645337458,-9.88367855660851));
#43450=CARTESIAN_POINT('',(17.3,-8.44469645337458,-9.88367855660851));
#43451=CARTESIAN_POINT('',(21.5,-8.44469645337458,-9.88367855660851));
#43452=CARTESIAN_POINT('',(25.7,-8.4979587007575,-9.4379392835629));
#43453=CARTESIAN_POINT('',(25.7,-8.43489648279215,-9.96569221502354));
#43454=CARTESIAN_POINT('',(17.3,-8.4979587007575,-9.4379392835629));
#43455=CARTESIAN_POINT('',(17.3,-8.4979587007575,-9.4379392835629));
#43456=CARTESIAN_POINT('',(17.3,-8.43489648279215,-9.96569221502354));
#43457=CARTESIAN_POINT('Origin',(17.3,-8.6150565568703,-9.56798962802145));
#43458=CARTESIAN_POINT('',(17.3,-8.94682358829601,-9.43156125357356));
#43459=CARTESIAN_POINT('Origin',(17.3,0.,0.));
#43460=CARTESIAN_POINT('',(17.3,-8.4979587007575,-9.4379392835629));
#43461=CARTESIAN_POINT('Origin',(17.3,-8.4979587007575,-9.4379392835629));
#43462=CARTESIAN_POINT('',(25.7,-8.94682358829601,-9.43156125357356));
#43463=CARTESIAN_POINT('',(21.5,-8.94682358829601,-9.43156125357356));
#43464=CARTESIAN_POINT('',(25.7,-8.4979587007575,-9.4379392835629));
#43465=CARTESIAN_POINT('Origin',(25.7,-8.6150565568703,-9.56798962802145));
#43466=CARTESIAN_POINT('Origin',(25.7,0.,0.));
#43467=CARTESIAN_POINT('Origin',(17.3,-10.3225576756761,-7.99420434016675));
#43468=CARTESIAN_POINT('',(25.7,-10.3150918949973,-7.91194534850694));
#43469=CARTESIAN_POINT('',(17.3,-10.3150918949973,-7.91194534850694));
#43470=CARTESIAN_POINT('',(21.5,-10.3150918949973,-7.91194534850694));
#43471=CARTESIAN_POINT('',(25.7,-10.2745158285618,-7.46487270411441));
#43472=CARTESIAN_POINT('',(25.7,-10.3225576756761,-7.99420434016675));
#43473=CARTESIAN_POINT('',(17.3,-10.2745158285618,-7.46487270411441));
#43474=CARTESIAN_POINT('',(17.3,-10.2745158285618,-7.46487270411441));
#43475=CARTESIAN_POINT('',(17.3,-10.3225576756761,-7.99420434016675));
#43476=CARTESIAN_POINT('Origin',(17.3,-10.4160938025774,-7.56773512326559));
#43477=CARTESIAN_POINT('',(17.3,-10.7122458743621,-7.36530979166607));
#43478=CARTESIAN_POINT('Origin',(17.3,0.,0.));
#43479=CARTESIAN_POINT('',(17.3,-10.2745158285618,-7.46487270411441));
#43480=CARTESIAN_POINT('Origin',(17.3,-10.2745158285618,-7.46487270411441));
#43481=CARTESIAN_POINT('',(25.7,-10.7122458743621,-7.36530979166607));
#43482=CARTESIAN_POINT('',(21.5,-10.7122458743621,-7.36530979166607));
#43483=CARTESIAN_POINT('',(25.7,-10.2745158285618,-7.46487270411441));
#43484=CARTESIAN_POINT('Origin',(25.7,-10.4160938025774,-7.56773512326559));
#43485=CARTESIAN_POINT('Origin',(25.7,0.,0.));
#43486=CARTESIAN_POINT('Origin',(17.3,-11.7590735650056,-5.67333137519623));
#43487=CARTESIAN_POINT('',(25.7,-11.7346683235061,-5.59442216294959));
#43488=CARTESIAN_POINT('',(17.3,-11.7346683235061,-5.59442216294959));
#43489=CARTESIAN_POINT('',(21.5,-11.7346683235061,-5.59442216294959));
#43490=CARTESIAN_POINT('',(25.7,-11.602027312061,-5.16555536706266));
#43491=CARTESIAN_POINT('',(25.7,-11.7590735650056,-5.67333137519623));
#43492=CARTESIAN_POINT('',(17.3,-11.602027312061,-5.16555536706266));
#43493=CARTESIAN_POINT('',(17.3,-11.602027312061,-5.16555536706266));
#43494=CARTESIAN_POINT('',(17.3,-11.7590735650056,-5.67333137519623));
#43495=CARTESIAN_POINT('Origin',(17.3,-11.7618977671485,-5.23673427960092));
#43496=CARTESIAN_POINT('',(17.3,-12.0094916126598,-4.97715894918517));
#43497=CARTESIAN_POINT('Origin',(17.3,0.,0.));
#43498=CARTESIAN_POINT('',(17.3,-11.602027312061,-5.16555536706266));
#43499=CARTESIAN_POINT('Origin',(17.3,-11.602027312061,-5.16555536706266));
#43500=CARTESIAN_POINT('',(25.7,-12.0094916126598,-4.97715894918517));
#43501=CARTESIAN_POINT('',(21.5,-12.0094916126598,-4.97715894918517));
#43502=CARTESIAN_POINT('',(25.7,-11.602027312061,-5.16555536706266));
#43503=CARTESIAN_POINT('Origin',(25.7,-11.7618977671485,-5.23673427960092));
#43504=CARTESIAN_POINT('Origin',(25.7,0.,0.));
#43505=CARTESIAN_POINT('Origin',(17.3,-12.6816615132491,-3.10450660546528));
#43506=CARTESIAN_POINT('',(25.7,-12.6413834370917,-3.03239588385541));
#43507=CARTESIAN_POINT('',(17.3,-12.6413834370917,-3.03239588385541));
#43508=CARTESIAN_POINT('',(21.5,-12.6413834370917,-3.03239588385541));
#43509=CARTESIAN_POINT('',(25.7,-12.4224745293193,-2.64047847338554));
#43510=CARTESIAN_POINT('',(25.7,-12.6816615132491,-3.10450660546528));
#43511=CARTESIAN_POINT('',(17.3,-12.4224745293193,-2.64047847338554));
#43512=CARTESIAN_POINT('',(17.3,-12.4224745293193,-2.64047847338554));
#43513=CARTESIAN_POINT('',(17.3,-12.6816615132491,-3.10450660546528));
#43514=CARTESIAN_POINT('Origin',(17.3,-12.5936503594478,-2.67686301927865));
#43515=CARTESIAN_POINT('',(17.3,-12.7818649395498,-2.37148237756647));
#43516=CARTESIAN_POINT('Origin',(17.3,0.,0.));
#43517=CARTESIAN_POINT('',(17.3,-12.4224745293193,-2.64047847338554));
#43518=CARTESIAN_POINT('Origin',(17.3,-12.4224745293193,-2.64047847338554));
#43519=CARTESIAN_POINT('',(25.7,-12.7818649395498,-2.37148237756647));
#43520=CARTESIAN_POINT('',(21.5,-12.7818649395498,-2.37148237756647));
#43521=CARTESIAN_POINT('',(25.7,-12.4224745293193,-2.64047847338554));
#43522=CARTESIAN_POINT('Origin',(25.7,-12.5936503594478,-2.67686301927865));
#43523=CARTESIAN_POINT('Origin',(25.7,0.,0.));
#43524=CARTESIAN_POINT('Origin',(17.3,-13.05,-0.399999999999998));
#43525=CARTESIAN_POINT('',(25.7,-12.9956094343885,-0.337839353586883));
#43526=CARTESIAN_POINT('',(17.3,-12.9956094343885,-0.337839353586883));
#43527=CARTESIAN_POINT('',(21.5,-12.9956094343885,-0.337839353586883));
#43528=CARTESIAN_POINT('',(25.7,-12.7,1.55530143491714E-15));
#43529=CARTESIAN_POINT('',(25.7,-13.05,-0.399999999999998));
#43530=CARTESIAN_POINT('',(17.3,-12.7,1.55530143491714E-15));
#43531=CARTESIAN_POINT('',(17.3,-12.7,1.55530143491714E-15));
#43532=CARTESIAN_POINT('',(17.3,-13.05,-0.399999999999998));
#43533=CARTESIAN_POINT('Origin',(17.3,-12.875,1.57673275390222E-15));
#43534=CARTESIAN_POINT('',(17.3,-13.,-1.59204083889156E-15));
#43535=CARTESIAN_POINT('Origin',(17.3,0.,0.));
#43536=CARTESIAN_POINT('',(17.3,-12.9956094343885,0.337839353586885));
#43537=CARTESIAN_POINT('',(17.3,-12.7,1.55530143491714E-15));
#43538=CARTESIAN_POINT('Origin',(17.3,0.,0.));
#43539=CARTESIAN_POINT('Origin',(17.3,-12.7,1.55530143491714E-15));
#43540=CARTESIAN_POINT('',(25.7,-12.9956094343885,0.337839353586885));
#43541=CARTESIAN_POINT('',(21.5,-12.9956094343885,0.337839353586885));
#43542=CARTESIAN_POINT('',(25.7,-12.7,1.55530143491714E-15));
#43543=CARTESIAN_POINT('Origin',(25.7,-12.875,1.57673275390222E-15));
#43544=CARTESIAN_POINT('',(25.7,-13.,-1.59204083889156E-15));
#43545=CARTESIAN_POINT('Origin',(25.7,0.,0.));
#43546=CARTESIAN_POINT('Origin',(25.7,0.,0.));
#43547=CARTESIAN_POINT('Origin',(17.3,-12.8479908659033,2.32198852487824));
#43548=CARTESIAN_POINT('',(25.7,-12.7818649395498,2.37148237756648));
#43549=CARTESIAN_POINT('',(17.3,-12.7818649395498,2.37148237756648));
#43550=CARTESIAN_POINT('',(21.5,-12.7818649395498,2.37148237756648));
#43551=CARTESIAN_POINT('',(25.7,-12.4224745293193,2.64047847338555));
#43552=CARTESIAN_POINT('',(25.7,-12.8479908659033,2.32198852487824));
#43553=CARTESIAN_POINT('',(17.3,-12.4224745293193,2.64047847338555));
#43554=CARTESIAN_POINT('',(17.3,-12.4224745293193,2.64047847338555));
#43555=CARTESIAN_POINT('',(17.3,-12.8479908659033,2.32198852487824));
#43556=CARTESIAN_POINT('Origin',(17.3,-12.5936503594477,2.67686301927866));
#43557=CARTESIAN_POINT('',(17.3,-12.6413834370917,3.03239588385542));
#43558=CARTESIAN_POINT('Origin',(17.3,0.,0.));
#43559=CARTESIAN_POINT('',(17.3,-12.4224745293193,2.64047847338555));
#43560=CARTESIAN_POINT('Origin',(17.3,-12.4224745293193,2.64047847338555));
#43561=CARTESIAN_POINT('',(25.7,-12.6413834370917,3.03239588385542));
#43562=CARTESIAN_POINT('',(21.5,-12.6413834370917,3.03239588385542));
#43563=CARTESIAN_POINT('',(25.7,-12.4224745293193,2.64047847338555));
#43564=CARTESIAN_POINT('Origin',(25.7,-12.5936503594477,2.67686301927866));
#43565=CARTESIAN_POINT('Origin',(25.7,0.,0.));
#43566=CARTESIAN_POINT('Origin',(17.3,-12.0844628794663,4.94249500908216));
#43567=CARTESIAN_POINT('',(25.7,-12.0094916126598,4.97715894918518));
#43568=CARTESIAN_POINT('',(17.3,-12.0094916126598,4.97715894918518));
#43569=CARTESIAN_POINT('',(21.5,-12.0094916126598,4.97715894918518));
#43570=CARTESIAN_POINT('',(25.7,-11.602027312061,5.16555536706267));
#43571=CARTESIAN_POINT('',(25.7,-12.0844628794663,4.94249500908216));
#43572=CARTESIAN_POINT('',(17.3,-11.602027312061,5.16555536706267));
#43573=CARTESIAN_POINT('',(17.3,-11.602027312061,5.16555536706267));
#43574=CARTESIAN_POINT('',(17.3,-12.0844628794663,4.94249500908216));
#43575=CARTESIAN_POINT('Origin',(17.3,-11.7618977671485,5.23673427960093));
#43576=CARTESIAN_POINT('',(17.3,-11.7346683235061,5.5944221629496));
#43577=CARTESIAN_POINT('Origin',(17.3,0.,0.));
#43578=CARTESIAN_POINT('',(17.3,-11.602027312061,5.16555536706267));
#43579=CARTESIAN_POINT('Origin',(17.3,-11.602027312061,5.16555536706267));
#43580=CARTESIAN_POINT('',(25.7,-11.7346683235061,5.5944221629496));
#43581=CARTESIAN_POINT('',(21.5,-11.7346683235061,5.5944221629496));
#43582=CARTESIAN_POINT('',(25.7,-11.602027312061,5.16555536706267));
#43583=CARTESIAN_POINT('Origin',(25.7,-11.7618977671485,5.23673427960093));
#43584=CARTESIAN_POINT('Origin',(25.7,0.,0.));
#43585=CARTESIAN_POINT('Origin',(17.3,-10.7927858775101,7.3469907446668));
#43586=CARTESIAN_POINT('',(25.7,-10.7122458743621,7.36530979166607));
#43587=CARTESIAN_POINT('',(17.3,-10.7122458743621,7.36530979166607));
#43588=CARTESIAN_POINT('',(21.5,-10.7122458743621,7.36530979166607));
#43589=CARTESIAN_POINT('',(25.7,-10.2745158285618,7.46487270411441));
#43590=CARTESIAN_POINT('',(25.7,-10.7927858775101,7.3469907446668));
#43591=CARTESIAN_POINT('',(17.3,-10.2745158285618,7.46487270411441));
#43592=CARTESIAN_POINT('',(17.3,-10.2745158285618,7.46487270411441));
#43593=CARTESIAN_POINT('',(17.3,-10.7927858775101,7.3469907446668));
#43594=CARTESIAN_POINT('Origin',(17.3,-10.4160938025774,7.56773512326559));
#43595=CARTESIAN_POINT('',(17.3,-10.3150918949973,7.91194534850694));
#43596=CARTESIAN_POINT('Origin',(17.3,0.,0.));
#43597=CARTESIAN_POINT('',(17.3,-10.2745158285618,7.46487270411441));
#43598=CARTESIAN_POINT('Origin',(17.3,-10.2745158285618,7.46487270411441));
#43599=CARTESIAN_POINT('',(25.7,-10.3150918949973,7.91194534850694));
#43600=CARTESIAN_POINT('',(21.5,-10.3150918949973,7.91194534850694));
#43601=CARTESIAN_POINT('',(25.7,-10.2745158285618,7.46487270411441));
#43602=CARTESIAN_POINT('Origin',(25.7,-10.4160938025774,7.56773512326559));
#43603=CARTESIAN_POINT('Origin',(25.7,0.,0.));
#43604=CARTESIAN_POINT('Origin',(17.3,-9.02941234317406,9.43038772993646));
#43605=CARTESIAN_POINT('',(25.7,-8.94682358829601,9.43156125357357));
#43606=CARTESIAN_POINT('',(17.3,-8.94682358829601,9.43156125357357));
#43607=CARTESIAN_POINT('',(21.5,-8.94682358829601,9.43156125357357));
#43608=CARTESIAN_POINT('',(25.7,-8.4979587007575,9.43793928356291));
#43609=CARTESIAN_POINT('',(25.7,-9.02941234317406,9.43038772993646));
#43610=CARTESIAN_POINT('',(17.3,-8.4979587007575,9.43793928356291));
#43611=CARTESIAN_POINT('',(17.3,-8.4979587007575,9.43793928356291));
#43612=CARTESIAN_POINT('',(17.3,-9.02941234317406,9.43038772993646));
#43613=CARTESIAN_POINT('Origin',(17.3,-8.6150565568703,9.56798962802145));
#43614=CARTESIAN_POINT('',(17.3,-8.44469645337457,9.88367855660852));
#43615=CARTESIAN_POINT('Origin',(17.3,0.,0.));
#43616=CARTESIAN_POINT('',(17.3,-8.4979587007575,9.43793928356291));
#43617=CARTESIAN_POINT('Origin',(17.3,-8.4979587007575,9.43793928356291));
#43618=CARTESIAN_POINT('',(25.7,-8.44469645337457,9.88367855660852));
#43619=CARTESIAN_POINT('',(21.5,-8.44469645337457,9.88367855660852));
#43620=CARTESIAN_POINT('',(25.7,-8.4979587007575,9.43793928356291));
#43621=CARTESIAN_POINT('Origin',(25.7,-8.6150565568703,9.56798962802145));
#43622=CARTESIAN_POINT('Origin',(25.7,0.,0.));
#43623=CARTESIAN_POINT('Origin',(17.3,-6.87141016151377,11.1016315193869));
#43624=CARTESIAN_POINT('',(25.7,-6.79038217979861,11.0856082310477));
#43625=CARTESIAN_POINT('',(17.3,-6.79038217979861,11.0856082310477));
#43626=CARTESIAN_POINT('',(21.5,-6.79038217979861,11.0856082310477));
#43627=CARTESIAN_POINT('',(25.7,-6.35,10.9985226280624));
#43628=CARTESIAN_POINT('',(25.7,-6.87141016151377,11.1016315193869));
#43629=CARTESIAN_POINT('',(17.3,-6.35,10.9985226280624));
#43630=CARTESIAN_POINT('',(17.3,-6.35,10.9985226280624));
#43631=CARTESIAN_POINT('',(17.3,-6.87141016151377,11.1016315193869));
#43632=CARTESIAN_POINT('Origin',(17.3,-6.4375,11.1500770737247));
#43633=CARTESIAN_POINT('',(17.3,-6.2052272545899,11.4234475846346));
#43634=CARTESIAN_POINT('Origin',(17.3,0.,0.));
#43635=CARTESIAN_POINT('',(17.3,-6.35,10.9985226280624));
#43636=CARTESIAN_POINT('Origin',(17.3,-6.35,10.9985226280624));
#43637=CARTESIAN_POINT('',(25.7,-6.2052272545899,11.4234475846346));
#43638=CARTESIAN_POINT('',(21.5,-6.2052272545899,11.4234475846346));
#43639=CARTESIAN_POINT('',(25.7,-6.35,10.9985226280624));
#43640=CARTESIAN_POINT('Origin',(25.7,-6.4375,11.1500770737247));
#43641=CARTESIAN_POINT('Origin',(25.7,0.,0.));
#43642=CARTESIAN_POINT('Origin',(17.3,-4.41309438311112,12.2876807399018));
#43643=CARTESIAN_POINT('',(25.7,-4.3371684861752,12.255160934175));
#43644=CARTESIAN_POINT('',(17.3,-4.3371684861752,12.255160934175));
#43645=CARTESIAN_POINT('',(21.5,-4.3371684861752,12.255160934175));
#43646=CARTESIAN_POINT('',(25.7,-3.92451582856183,12.0784177569485));
#43647=CARTESIAN_POINT('',(25.7,-4.41309438311112,12.2876807399018));
#43648=CARTESIAN_POINT('',(17.3,-3.92451582856183,12.0784177569485));
#43649=CARTESIAN_POINT('',(17.3,-3.92451582856183,12.0784177569485));
#43650=CARTESIAN_POINT('',(17.3,-4.41309438311112,12.2876807399018));
#43651=CARTESIAN_POINT('Origin',(17.3,-3.97859380257745,12.2448526473001));
#43652=CARTESIAN_POINT('',(17.3,-3.6945598487957,12.463957137429));
#43653=CARTESIAN_POINT('Origin',(17.3,0.,0.));
#43654=CARTESIAN_POINT('',(17.3,-3.92451582856183,12.0784177569485));
#43655=CARTESIAN_POINT('Origin',(17.3,-3.92451582856183,12.0784177569485));
#43656=CARTESIAN_POINT('',(25.7,-3.6945598487957,12.463957137429));
#43657=CARTESIAN_POINT('',(21.5,-3.6945598487957,12.463957137429));
#43658=CARTESIAN_POINT('',(25.7,-3.92451582856183,12.0784177569485));
#43659=CARTESIAN_POINT('Origin',(25.7,-3.97859380257745,12.2448526473001));
#43660=CARTESIAN_POINT('Origin',(25.7,0.,0.));
#43661=CARTESIAN_POINT('Origin',(17.3,-1.76190520379019,12.9366993492489));
#43662=CARTESIAN_POINT('',(25.7,-1.69439971766247,12.8891042976921));
#43663=CARTESIAN_POINT('',(17.3,-1.69439971766247,12.8891042976921));
#43664=CARTESIAN_POINT('',(21.5,-1.69439971766247,12.8891042976921));
#43665=CARTESIAN_POINT('',(25.7,-1.3275114834992,12.6304280711771));
#43666=CARTESIAN_POINT('',(25.7,-1.76190520379019,12.9366993492489));
#43667=CARTESIAN_POINT('',(17.3,-1.3275114834992,12.6304280711771));
#43668=CARTESIAN_POINT('',(17.3,-1.3275114834992,12.6304280711771));
#43669=CARTESIAN_POINT('',(17.3,-1.76190520379019,12.9366993492489));
#43670=CARTESIAN_POINT('Origin',(17.3,-1.34580396457104,12.8044694028665));
#43671=CARTESIAN_POINT('',(17.3,-1.02242244914403,12.9597319546157));
#43672=CARTESIAN_POINT('Origin',(17.3,0.,0.));
#43673=CARTESIAN_POINT('',(17.3,-1.3275114834992,12.6304280711771));
#43674=CARTESIAN_POINT('Origin',(17.3,-1.3275114834992,12.6304280711771));
#43675=CARTESIAN_POINT('',(25.7,-1.02242244914403,12.9597319546157));
#43676=CARTESIAN_POINT('',(21.5,-1.02242244914403,12.9597319546157));
#43677=CARTESIAN_POINT('',(25.7,-1.3275114834992,12.6304280711771));
#43678=CARTESIAN_POINT('Origin',(25.7,-1.34580396457104,12.8044694028665));
#43679=CARTESIAN_POINT('Origin',(25.7,0.,0.));
#43680=CARTESIAN_POINT('Origin',(17.3,0.966287687495571,13.020322119863));
#43681=CARTESIAN_POINT('',(25.7,1.02242244914404,12.9597319546157));
#43682=CARTESIAN_POINT('',(17.3,1.02242244914404,12.9597319546157));
#43683=CARTESIAN_POINT('',(21.5,1.02242244914404,12.9597319546157));
#43684=CARTESIAN_POINT('',(25.7,1.3275114834992,12.6304280711771));
#43685=CARTESIAN_POINT('',(25.7,0.966287687495571,13.020322119863));
#43686=CARTESIAN_POINT('',(17.3,1.3275114834992,12.6304280711771));
#43687=CARTESIAN_POINT('',(17.3,1.3275114834992,12.6304280711771));
#43688=CARTESIAN_POINT('',(17.3,0.966287687495571,13.020322119863));
#43689=CARTESIAN_POINT('Origin',(17.3,1.34580396457104,12.8044694028665));
#43690=CARTESIAN_POINT('',(17.3,1.69439971766247,12.8891042976921));
#43691=CARTESIAN_POINT('Origin',(17.3,0.,0.));
#43692=CARTESIAN_POINT('',(17.3,1.3275114834992,12.6304280711771));
#43693=CARTESIAN_POINT('Origin',(17.3,1.3275114834992,12.6304280711771));
#43694=CARTESIAN_POINT('',(25.7,1.69439971766247,12.8891042976921));
#43695=CARTESIAN_POINT('',(21.5,1.69439971766247,12.8891042976921));
#43696=CARTESIAN_POINT('',(25.7,1.3275114834992,12.6304280711771));
#43697=CARTESIAN_POINT('Origin',(25.7,1.34580396457104,12.8044694028665));
#43698=CARTESIAN_POINT('Origin',(25.7,0.,0.));
#43699=CARTESIAN_POINT('Origin',(17.3,3.652249170075,12.5348943354017));
#43700=CARTESIAN_POINT('',(25.7,3.69455984879571,12.463957137429));
#43701=CARTESIAN_POINT('',(17.3,3.69455984879571,12.463957137429));
#43702=CARTESIAN_POINT('',(21.5,3.69455984879571,12.463957137429));
#43703=CARTESIAN_POINT('',(25.7,3.92451582856183,12.0784177569485));
#43704=CARTESIAN_POINT('',(25.7,3.652249170075,12.5348943354017));
#43705=CARTESIAN_POINT('',(17.3,3.92451582856183,12.0784177569485));
#43706=CARTESIAN_POINT('',(17.3,3.92451582856183,12.0784177569485));
#43707=CARTESIAN_POINT('',(17.3,3.652249170075,12.5348943354017));
#43708=CARTESIAN_POINT('Origin',(17.3,3.97859380257745,12.2448526473001));
#43709=CARTESIAN_POINT('',(17.3,4.3371684861752,12.255160934175));
#43710=CARTESIAN_POINT('Origin',(17.3,0.,0.));
#43711=CARTESIAN_POINT('',(17.3,3.92451582856183,12.0784177569485));
#43712=CARTESIAN_POINT('Origin',(17.3,3.92451582856183,12.0784177569485));
#43713=CARTESIAN_POINT('',(25.7,4.3371684861752,12.255160934175));
#43714=CARTESIAN_POINT('',(21.5,4.3371684861752,12.255160934175));
#43715=CARTESIAN_POINT('',(25.7,3.92451582856183,12.0784177569485));
#43716=CARTESIAN_POINT('Origin',(25.7,3.97859380257745,12.2448526473001));
#43717=CARTESIAN_POINT('Origin',(25.7,0.,0.));
#43718=CARTESIAN_POINT('Origin',(17.3,6.17858983848623,11.5016315193869));
#43719=CARTESIAN_POINT('',(25.7,6.20522725458991,11.4234475846346));
#43720=CARTESIAN_POINT('',(17.3,6.20522725458991,11.4234475846346));
#43721=CARTESIAN_POINT('',(21.5,6.20522725458991,11.4234475846346));
#43722=CARTESIAN_POINT('',(25.7,6.35,10.9985226280624));
#43723=CARTESIAN_POINT('',(25.7,6.17858983848623,11.5016315193869));
#43724=CARTESIAN_POINT('',(17.3,6.35,10.9985226280624));
#43725=CARTESIAN_POINT('',(17.3,6.35,10.9985226280624));
#43726=CARTESIAN_POINT('',(17.3,6.17858983848623,11.5016315193869));
#43727=CARTESIAN_POINT('Origin',(17.3,6.4375,11.1500770737246));
#43728=CARTESIAN_POINT('',(17.3,6.79038217979862,11.0856082310477));
#43729=CARTESIAN_POINT('Origin',(17.3,0.,0.));
#43730=CARTESIAN_POINT('',(17.3,6.35,10.9985226280624));
#43731=CARTESIAN_POINT('Origin',(17.3,6.35,10.9985226280624));
#43732=CARTESIAN_POINT('',(25.7,6.79038217979862,11.0856082310477));
#43733=CARTESIAN_POINT('',(21.5,6.79038217979862,11.0856082310477));
#43734=CARTESIAN_POINT('',(25.7,6.35,10.9985226280624));
#43735=CARTESIAN_POINT('Origin',(25.7,6.4375,11.1500770737246));
#43736=CARTESIAN_POINT('Origin',(25.7,0.,0.));
#43737=CARTESIAN_POINT('Origin',(17.3,8.43489648279215,9.96569221502354));
#43738=CARTESIAN_POINT('',(25.7,8.44469645337458,9.88367855660851));
#43739=CARTESIAN_POINT('',(17.3,8.44469645337458,9.88367855660851));
#43740=CARTESIAN_POINT('',(21.5,8.44469645337458,9.88367855660851));
#43741=CARTESIAN_POINT('',(25.7,8.4979587007575,9.43793928356291));
#43742=CARTESIAN_POINT('',(25.7,8.43489648279215,9.96569221502354));
#43743=CARTESIAN_POINT('',(17.3,8.4979587007575,9.43793928356291));
#43744=CARTESIAN_POINT('',(17.3,8.4979587007575,9.43793928356291));
#43745=CARTESIAN_POINT('',(17.3,8.43489648279215,9.96569221502354));
#43746=CARTESIAN_POINT('Origin',(17.3,8.6150565568703,9.56798962802145));
#43747=CARTESIAN_POINT('',(17.3,8.94682358829601,9.43156125357356));
#43748=CARTESIAN_POINT('Origin',(17.3,0.,0.));
#43749=CARTESIAN_POINT('',(17.3,8.4979587007575,9.43793928356291));
#43750=CARTESIAN_POINT('Origin',(17.3,8.4979587007575,9.43793928356291));
#43751=CARTESIAN_POINT('',(25.7,8.94682358829601,9.43156125357356));
#43752=CARTESIAN_POINT('',(21.5,8.94682358829601,9.43156125357356));
#43753=CARTESIAN_POINT('',(25.7,8.4979587007575,9.43793928356291));
#43754=CARTESIAN_POINT('Origin',(25.7,8.6150565568703,9.56798962802145));
#43755=CARTESIAN_POINT('Origin',(25.7,0.,0.));
#43756=CARTESIAN_POINT('Origin',(17.3,10.3225576756761,7.99420434016675));
#43757=CARTESIAN_POINT('',(25.7,10.3150918949973,7.91194534850694));
#43758=CARTESIAN_POINT('',(17.3,10.3150918949973,7.91194534850694));
#43759=CARTESIAN_POINT('',(21.5,10.3150918949973,7.91194534850694));
#43760=CARTESIAN_POINT('',(25.7,10.2745158285618,7.46487270411441));
#43761=CARTESIAN_POINT('',(25.7,10.3225576756761,7.99420434016675));
#43762=CARTESIAN_POINT('',(17.3,10.2745158285618,7.46487270411441));
#43763=CARTESIAN_POINT('',(17.3,10.2745158285618,7.46487270411441));
#43764=CARTESIAN_POINT('',(17.3,10.3225576756761,7.99420434016675));
#43765=CARTESIAN_POINT('Origin',(17.3,10.4160938025774,7.56773512326559));
#43766=CARTESIAN_POINT('',(17.3,10.7122458743621,7.36530979166607));
#43767=CARTESIAN_POINT('Origin',(17.3,0.,0.));
#43768=CARTESIAN_POINT('',(17.3,10.2745158285618,7.46487270411441));
#43769=CARTESIAN_POINT('Origin',(17.3,10.2745158285618,7.46487270411441));
#43770=CARTESIAN_POINT('',(25.7,10.7122458743621,7.36530979166607));
#43771=CARTESIAN_POINT('',(21.5,10.7122458743621,7.36530979166607));
#43772=CARTESIAN_POINT('',(25.7,10.2745158285618,7.46487270411441));
#43773=CARTESIAN_POINT('Origin',(25.7,10.4160938025774,7.56773512326559));
#43774=CARTESIAN_POINT('Origin',(25.7,0.,0.));
#43775=CARTESIAN_POINT('Origin',(17.3,11.7590735650056,5.67333137519623));
#43776=CARTESIAN_POINT('',(25.7,11.7346683235061,5.59442216294959));
#43777=CARTESIAN_POINT('',(17.3,11.7346683235061,5.59442216294959));
#43778=CARTESIAN_POINT('',(21.5,11.7346683235061,5.59442216294959));
#43779=CARTESIAN_POINT('',(25.7,11.602027312061,5.16555536706266));
#43780=CARTESIAN_POINT('',(25.7,11.7590735650056,5.67333137519623));
#43781=CARTESIAN_POINT('',(17.3,11.602027312061,5.16555536706266));
#43782=CARTESIAN_POINT('',(17.3,11.602027312061,5.16555536706266));
#43783=CARTESIAN_POINT('',(17.3,11.7590735650056,5.67333137519623));
#43784=CARTESIAN_POINT('Origin',(17.3,11.7618977671485,5.23673427960093));
#43785=CARTESIAN_POINT('',(17.3,12.0094916126598,4.97715894918518));
#43786=CARTESIAN_POINT('Origin',(17.3,0.,0.));
#43787=CARTESIAN_POINT('',(17.3,11.602027312061,5.16555536706266));
#43788=CARTESIAN_POINT('Origin',(17.3,11.602027312061,5.16555536706266));
#43789=CARTESIAN_POINT('',(25.7,12.0094916126598,4.97715894918518));
#43790=CARTESIAN_POINT('',(21.5,12.0094916126598,4.97715894918518));
#43791=CARTESIAN_POINT('',(25.7,11.602027312061,5.16555536706266));
#43792=CARTESIAN_POINT('Origin',(25.7,11.7618977671485,5.23673427960093));
#43793=CARTESIAN_POINT('Origin',(25.7,0.,0.));
#43794=CARTESIAN_POINT('Origin',(17.3,12.6816615132491,3.10450660546528));
#43795=CARTESIAN_POINT('',(25.7,12.6413834370917,3.03239588385541));
#43796=CARTESIAN_POINT('',(17.3,12.6413834370917,3.03239588385541));
#43797=CARTESIAN_POINT('',(21.5,12.6413834370917,3.03239588385541));
#43798=CARTESIAN_POINT('',(25.7,12.4224745293193,2.64047847338554));
#43799=CARTESIAN_POINT('',(25.7,12.6816615132491,3.10450660546528));
#43800=CARTESIAN_POINT('',(17.3,12.4224745293193,2.64047847338554));
#43801=CARTESIAN_POINT('',(17.3,12.4224745293193,2.64047847338554));
#43802=CARTESIAN_POINT('',(17.3,12.6816615132491,3.10450660546528));
#43803=CARTESIAN_POINT('Origin',(17.3,12.5936503594478,2.67686301927865));
#43804=CARTESIAN_POINT('',(17.3,12.7818649395498,2.37148237756647));
#43805=CARTESIAN_POINT('Origin',(17.3,0.,0.));
#43806=CARTESIAN_POINT('',(17.3,12.4224745293193,2.64047847338554));
#43807=CARTESIAN_POINT('Origin',(17.3,12.4224745293193,2.64047847338554));
#43808=CARTESIAN_POINT('',(25.7,12.7818649395498,2.37148237756647));
#43809=CARTESIAN_POINT('',(21.5,12.7818649395498,2.37148237756647));
#43810=CARTESIAN_POINT('',(25.7,12.4224745293193,2.64047847338554));
#43811=CARTESIAN_POINT('Origin',(25.7,12.5936503594478,2.67686301927865));
#43812=CARTESIAN_POINT('Origin',(25.7,0.,0.));
#43813=CARTESIAN_POINT('Origin',(17.3,13.05,0.4));
#43814=CARTESIAN_POINT('',(25.7,12.9956094343885,0.337839353586883));
#43815=CARTESIAN_POINT('',(17.3,12.9956094343885,0.337839353586883));
#43816=CARTESIAN_POINT('',(21.5,12.9956094343885,0.337839353586883));
#43817=CARTESIAN_POINT('',(25.7,12.7,0.));
#43818=CARTESIAN_POINT('',(25.7,13.05,0.4));
#43819=CARTESIAN_POINT('',(17.3,12.7,0.));
#43820=CARTESIAN_POINT('',(17.3,12.7,0.));
#43821=CARTESIAN_POINT('',(17.3,13.05,0.4));
#43822=CARTESIAN_POINT('Origin',(17.3,12.875,0.));
#43823=CARTESIAN_POINT('',(17.3,12.9956094343885,-0.337839353586884));
#43824=CARTESIAN_POINT('Origin',(17.3,0.,0.));
#43825=CARTESIAN_POINT('',(17.3,12.7,0.));
#43826=CARTESIAN_POINT('Origin',(17.3,12.7,0.));
#43827=CARTESIAN_POINT('',(25.7,12.9956094343885,-0.337839353586884));
#43828=CARTESIAN_POINT('',(21.5,12.9956094343885,-0.337839353586884));
#43829=CARTESIAN_POINT('',(25.7,12.7,0.));
#43830=CARTESIAN_POINT('Origin',(25.7,12.875,0.));
#43831=CARTESIAN_POINT('Origin',(25.7,0.,0.));
#43832=CARTESIAN_POINT('Origin',(0.,1.5,0.));
#43833=CARTESIAN_POINT('',(2.77555756156289E-16,-1.5,-1.83697019872103E-16));
#43834=CARTESIAN_POINT('Origin',(0.,0.,0.));
#43835=CARTESIAN_POINT('Origin',(1.,0.,0.));
#43836=CARTESIAN_POINT('',(2.,-4.5,-5.51091059616309E-16));
#43837=CARTESIAN_POINT('Origin',(2.,0.,0.));
#43838=CARTESIAN_POINT('',(1.,-3.,-3.67394039744206E-16));
#43839=CARTESIAN_POINT('Origin',(2.25,0.,0.));
#43840=CARTESIAN_POINT('',(2.25,-4.75,-5.81707229594993E-16));
#43841=CARTESIAN_POINT('Origin',(8.75,0.,0.));
#43842=CARTESIAN_POINT('Origin',(15.75,0.,0.));
#43843=CARTESIAN_POINT('',(16.5,-4.,-4.89858719658941E-16));
#43844=CARTESIAN_POINT('Origin',(16.5,0.,0.));
#43845=CARTESIAN_POINT('',(15.75,-4.,-4.89858719658941E-16));
#43846=CARTESIAN_POINT('Origin',(16.5,12.4,0.));
#43847=CARTESIAN_POINT('',(16.5,-12.4,-1.51856203094272E-15));
#43848=CARTESIAN_POINT('Origin',(16.5,0.,0.));
#43849=CARTESIAN_POINT('Origin',(16.8,0.,0.));
#43850=CARTESIAN_POINT('',(17.1,-13.,-1.59204083889156E-15));
#43851=CARTESIAN_POINT('Origin',(17.1,0.,0.));
#43852=CARTESIAN_POINT('',(16.8,-12.7,-1.55530143491714E-15));
#43853=CARTESIAN_POINT('Origin',(21.5,0.,0.));
#43854=CARTESIAN_POINT('',(25.9,-13.,-1.59204083889156E-15));
#43855=CARTESIAN_POINT('Origin',(25.9,0.,0.));
#43856=CARTESIAN_POINT('',(21.5,-13.,-1.59204083889156E-15));
#43857=CARTESIAN_POINT('',(21.5,-13.,-1.59204083889156E-15));
#43858=CARTESIAN_POINT('Origin',(26.2,0.,0.));
#43859=CARTESIAN_POINT('',(26.5,-12.4,-1.51856203094272E-15));
#43860=CARTESIAN_POINT('Origin',(26.5,0.,0.));
#43861=CARTESIAN_POINT('',(26.2,-12.7,-1.55530143491714E-15));
#43862=CARTESIAN_POINT('Origin',(26.5,0.,0.));
#45207=UNCERTAINTY_MEASURE_WITH_UNIT(LENGTH_MEASURE(0.01),#45237,
'DISTANCE_ACCURACY_VALUE',
'Maximum model space distance between geometric entities at asserted c
onnectivities');
#45214=UNCERTAINTY_MEASURE_WITH_UNIT(LENGTH_MEASURE(0.01),#45237,
'DISTANCE_ACCURACY_VALUE',
'Maximum model space distance between geometric entities at asserted c
onnectivities');
#45229=(
GEOMETRIC_REPRESENTATION_CONTEXT(3)
GLOBAL_UNCERTAINTY_ASSIGNED_CONTEXT((#45207))
GLOBAL_UNIT_ASSIGNED_CONTEXT((#45237,#45239,#45240))
REPRESENTATION_CONTEXT('','3D')
);
#45236=(
GEOMETRIC_REPRESENTATION_CONTEXT(3)
GLOBAL_UNCERTAINTY_ASSIGNED_CONTEXT((#45214))
GLOBAL_UNIT_ASSIGNED_CONTEXT((#45237,#45239,#45240))
REPRESENTATION_CONTEXT('','3D')
);
#45237=(
LENGTH_UNIT()
NAMED_UNIT(*)
SI_UNIT(.MILLI.,.METRE.)
);
#45239=(
NAMED_UNIT(*)
PLANE_ANGLE_UNIT()
SI_UNIT($,.RADIAN.)
);
#45240=(
NAMED_UNIT(*)
SI_UNIT($,.STERADIAN.)
SOLID_ANGLE_UNIT()
);
#45255=SHAPE_DEFINITION_REPRESENTATION(#45276,#45327);
#45276=PRODUCT_DEFINITION_SHAPE('',$,#45349);
#45327=SHAPE_REPRESENTATION('',(#17601),#45229);
#45334=PRODUCT_DEFINITION_CONTEXT('part definition',#45399,'design');
#45349=PRODUCT_DEFINITION('2026-10-25-23-38-30-333',
'20_Oil_Return_Valve_Knob_M10x1',#45370,#45334);
#45370=PRODUCT_DEFINITION_FORMATION('',$,#45415);
#45399=APPLICATION_CONTEXT(
'Core Data for Automotive Mechanical Design Process');
#45400=PRODUCT_CONTEXT('part definition',#45399,'mechanical');
#45415=PRODUCT('2026-10-25-23-38-30-333',
'20_Oil_Return_Valve_Knob_M10x1',$,(#45400));
#45471=COLOUR_RGB('Sky Blue',0.24,0.69,0.87);
#45472=FILL_AREA_STYLE_COLOUR('',#45471);
#45473=FILL_AREA_STYLE('',(#45472));
#45474=SURFACE_STYLE_FILL_AREA(#45473);
#45475=SURFACE_SIDE_STYLE('',(#45474));
#45476=SURFACE_STYLE_USAGE(.BOTH.,#45475);
#45477=PRESENTATION_STYLE_ASSIGNMENT((#45476));
ENDSEC;
END-ISO-10303-21;
